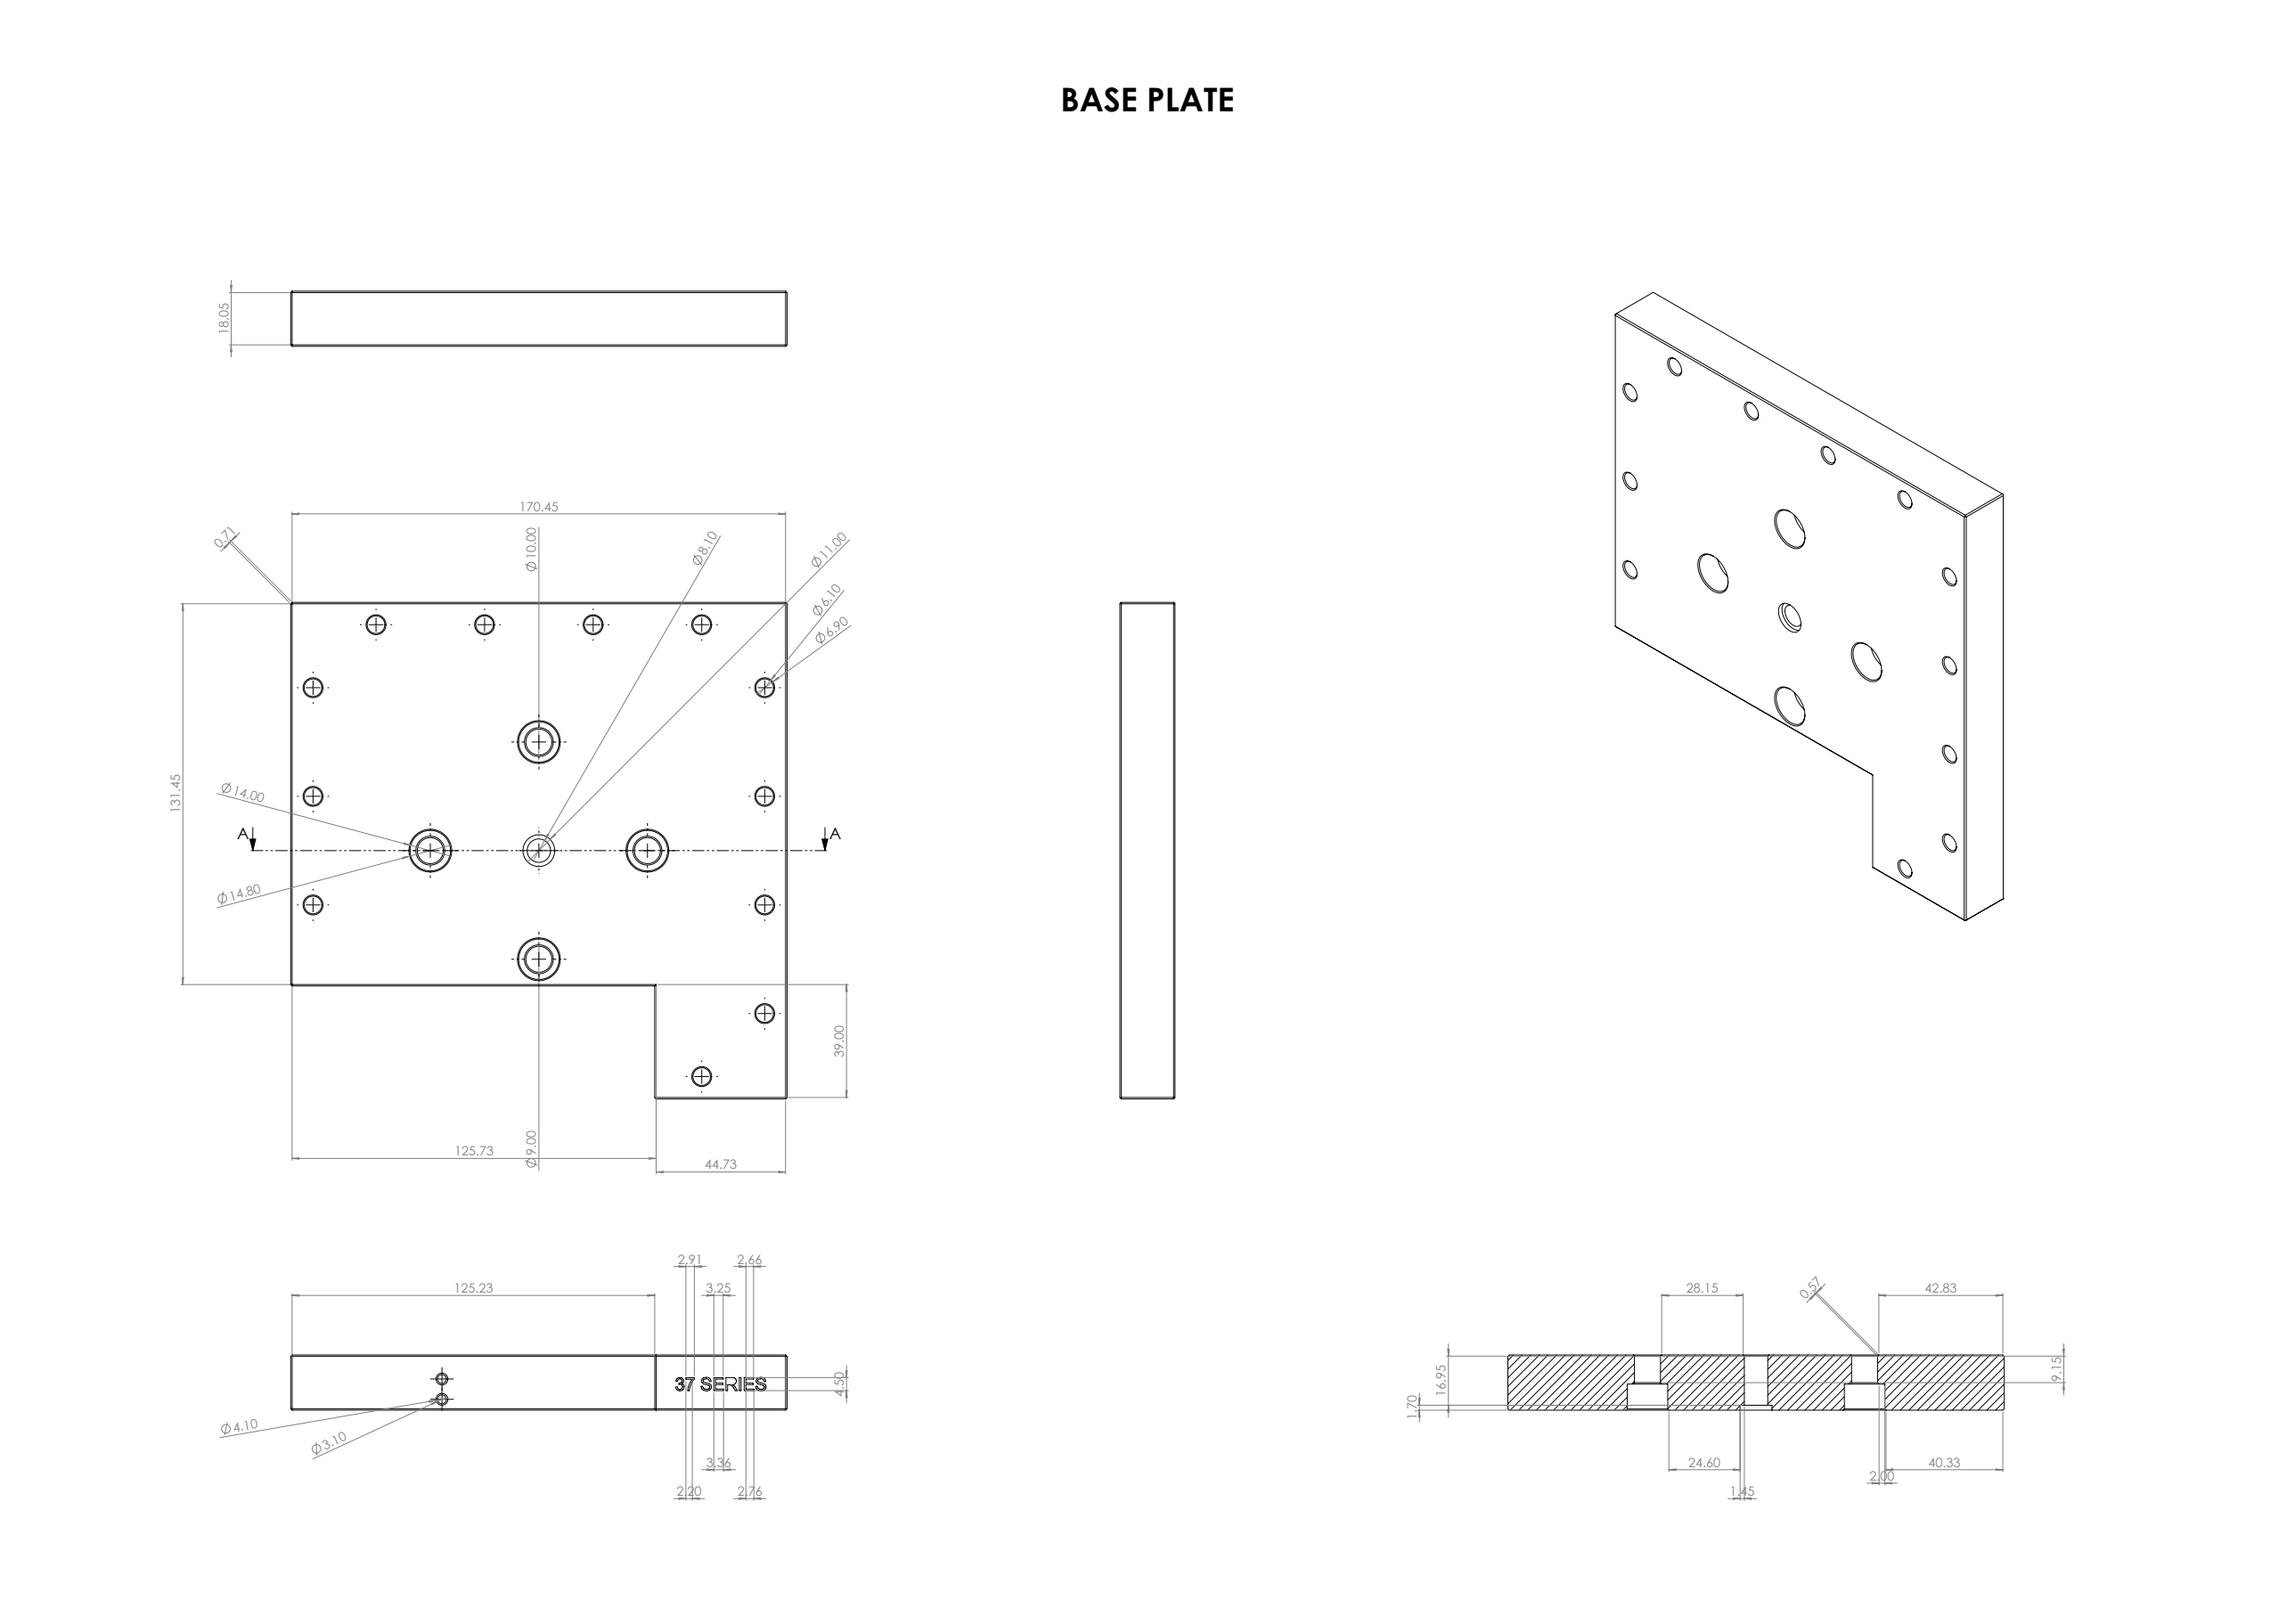
ISO-10303-21;
HEADER;
/* Generated by software containing ST-Developer
 * from STEP Tools, Inc. (www.steptools.com) 
 */

FILE_DESCRIPTION(
/* description */ (''),
/* implementation_level */ '2;1');

FILE_NAME(
/* name */ '01_Base_Plate.step',
/* time_stamp */ '2026-10-21T01:56:51-07:00',
/* author */ (''),
/* organization */ (''),
/* preprocessor_version */ 'ST-DEVELOPER v20.2',
/* originating_system */ 'Autodesk Translation Framework v15.15.0.0',
/* authorisation */ '');

FILE_SCHEMA (('AUTOMOTIVE_DESIGN { 1 0 10303 214 3 1 1 }'));
ENDSEC;

DATA;
#10=MECHANICAL_DESIGN_GEOMETRIC_PRESENTATION_REPRESENTATION('',(#270),#82384);
#232=SHAPE_REPRESENTATION_RELATIONSHIP('SRR','None',#82466,#251);
#251=ADVANCED_BREP_SHAPE_REPRESENTATION('',(#289),#82365);
#270=STYLED_ITEM('',(#82610),#289);
#289=MANIFOLD_SOLID_BREP('Body1',#30661);
#308=B_SPLINE_SURFACE_WITH_KNOTS('',2,1,((#41609,#41610),(#41611,#41612),
(#41613,#41614)),.UNSPECIFIED.,.F.,.F.,.F.,(3,3),(2,2),(0.,1.),(0.,0.0299999999999994),
 .UNSPECIFIED.);
#309=B_SPLINE_SURFACE_WITH_KNOTS('',2,1,((#41620,#41621),(#41622,#41623),
(#41624,#41625)),.UNSPECIFIED.,.F.,.F.,.F.,(3,3),(2,2),(0.,1.),(0.,0.0299999999999994),
 .UNSPECIFIED.);
#310=B_SPLINE_SURFACE_WITH_KNOTS('',2,1,((#41631,#41632),(#41633,#41634),
(#41635,#41636)),.UNSPECIFIED.,.F.,.F.,.F.,(3,3),(2,2),(0.,1.),(0.,0.0299999999999994),
 .UNSPECIFIED.);
#311=B_SPLINE_SURFACE_WITH_KNOTS('',2,1,((#41642,#41643),(#41644,#41645),
(#41646,#41647)),.UNSPECIFIED.,.F.,.F.,.F.,(3,3),(2,2),(0.,1.),(0.,0.0299999999999994),
 .UNSPECIFIED.);
#312=B_SPLINE_SURFACE_WITH_KNOTS('',2,1,((#41665,#41666),(#41667,#41668),
(#41669,#41670)),.UNSPECIFIED.,.F.,.F.,.F.,(3,3),(2,2),(0.,1.),(0.,0.0299999999999994),
 .UNSPECIFIED.);
#313=B_SPLINE_SURFACE_WITH_KNOTS('',2,1,((#41676,#41677),(#41678,#41679),
(#41680,#41681)),.UNSPECIFIED.,.F.,.F.,.F.,(3,3),(2,2),(0.,1.),(0.,0.0299999999999994),
 .UNSPECIFIED.);
#314=B_SPLINE_SURFACE_WITH_KNOTS('',2,1,((#41687,#41688),(#41689,#41690),
(#41691,#41692)),.UNSPECIFIED.,.F.,.F.,.F.,(3,3),(2,2),(0.,1.),(0.,0.0299999999999994),
 .UNSPECIFIED.);
#315=B_SPLINE_SURFACE_WITH_KNOTS('',2,1,((#41698,#41699),(#41700,#41701),
(#41702,#41703)),.UNSPECIFIED.,.F.,.F.,.F.,(3,3),(2,2),(0.,1.),(0.,0.0299999999999994),
 .UNSPECIFIED.);
#316=B_SPLINE_SURFACE_WITH_KNOTS('',2,1,((#41709,#41710),(#41711,#41712),
(#41713,#41714)),.UNSPECIFIED.,.F.,.F.,.F.,(3,3),(2,2),(0.,1.),(0.,0.0299999999999994),
 .UNSPECIFIED.);
#317=B_SPLINE_SURFACE_WITH_KNOTS('',2,1,((#41720,#41721),(#41722,#41723),
(#41724,#41725)),.UNSPECIFIED.,.F.,.F.,.F.,(3,3),(2,2),(0.,1.),(0.,0.0299999999999994),
 .UNSPECIFIED.);
#318=B_SPLINE_SURFACE_WITH_KNOTS('',2,1,((#41731,#41732),(#41733,#41734),
(#41735,#41736)),.UNSPECIFIED.,.F.,.F.,.F.,(3,3),(2,2),(0.,1.),(0.,0.0299999999999994),
 .UNSPECIFIED.);
#319=B_SPLINE_SURFACE_WITH_KNOTS('',2,1,((#41806,#41807),(#41808,#41809),
(#41810,#41811)),.UNSPECIFIED.,.F.,.F.,.F.,(3,3),(2,2),(0.,1.),(0.,0.0299999999999994),
 .UNSPECIFIED.);
#320=B_SPLINE_SURFACE_WITH_KNOTS('',2,1,((#41819,#41820),(#41821,#41822),
(#41823,#41824)),.UNSPECIFIED.,.F.,.F.,.F.,(3,3),(2,2),(0.,1.),(0.,0.0299999999999994),
 .UNSPECIFIED.);
#321=B_SPLINE_SURFACE_WITH_KNOTS('',2,1,((#41834,#41835),(#41836,#41837),
(#41838,#41839)),.UNSPECIFIED.,.F.,.F.,.F.,(3,3),(2,2),(0.,1.),(0.,0.0299999999999994),
 .UNSPECIFIED.);
#322=B_SPLINE_SURFACE_WITH_KNOTS('',2,1,((#41845,#41846),(#41847,#41848),
(#41849,#41850)),.UNSPECIFIED.,.F.,.F.,.F.,(3,3),(2,2),(0.,1.),(0.,0.0299999999999994),
 .UNSPECIFIED.);
#323=B_SPLINE_SURFACE_WITH_KNOTS('',2,1,((#41856,#41857),(#41858,#41859),
(#41860,#41861)),.UNSPECIFIED.,.F.,.F.,.F.,(3,3),(2,2),(0.,1.),(0.,0.0299999999999994),
 .UNSPECIFIED.);
#324=B_SPLINE_SURFACE_WITH_KNOTS('',2,1,((#41883,#41884),(#41885,#41886),
(#41887,#41888)),.UNSPECIFIED.,.F.,.F.,.F.,(3,3),(2,2),(0.,1.),(0.,0.0299999999999994),
 .UNSPECIFIED.);
#325=B_SPLINE_SURFACE_WITH_KNOTS('',2,1,((#41893,#41894),(#41895,#41896),
(#41897,#41898)),.UNSPECIFIED.,.F.,.F.,.F.,(3,3),(2,2),(0.,1.),(0.,0.0299999999999994),
 .UNSPECIFIED.);
#326=B_SPLINE_SURFACE_WITH_KNOTS('',2,1,((#41906,#41907),(#41908,#41909),
(#41910,#41911)),.UNSPECIFIED.,.F.,.F.,.F.,(3,3),(2,2),(0.,1.),(0.,0.0299999999999994),
 .UNSPECIFIED.);
#327=B_SPLINE_SURFACE_WITH_KNOTS('',2,1,((#41917,#41918),(#41919,#41920),
(#41921,#41922)),.UNSPECIFIED.,.F.,.F.,.F.,(3,3),(2,2),(0.,1.),(0.,0.0299999999999994),
 .UNSPECIFIED.);
#328=B_SPLINE_SURFACE_WITH_KNOTS('',2,1,((#41928,#41929),(#41930,#41931),
(#41932,#41933)),.UNSPECIFIED.,.F.,.F.,.F.,(3,3),(2,2),(0.,1.),(0.,0.0299999999999994),
 .UNSPECIFIED.);
#329=B_SPLINE_SURFACE_WITH_KNOTS('',2,1,((#41939,#41940),(#41941,#41942),
(#41943,#41944)),.UNSPECIFIED.,.F.,.F.,.F.,(3,3),(2,2),(0.,1.),(0.,0.0299999999999994),
 .UNSPECIFIED.);
#330=B_SPLINE_SURFACE_WITH_KNOTS('',2,1,((#41950,#41951),(#41952,#41953),
(#41954,#41955)),.UNSPECIFIED.,.F.,.F.,.F.,(3,3),(2,2),(0.,1.),(0.,0.0299999999999994),
 .UNSPECIFIED.);
#331=B_SPLINE_SURFACE_WITH_KNOTS('',2,1,((#41961,#41962),(#41963,#41964),
(#41965,#41966)),.UNSPECIFIED.,.F.,.F.,.F.,(3,3),(2,2),(0.,1.),(0.,0.0299999999999994),
 .UNSPECIFIED.);
#332=B_SPLINE_SURFACE_WITH_KNOTS('',2,1,((#41972,#41973),(#41974,#41975),
(#41976,#41977)),.UNSPECIFIED.,.F.,.F.,.F.,(3,3),(2,2),(0.,1.),(0.,0.0299999999999994),
 .UNSPECIFIED.);
#333=B_SPLINE_SURFACE_WITH_KNOTS('',2,1,((#41983,#41984),(#41985,#41986),
(#41987,#41988)),.UNSPECIFIED.,.F.,.F.,.F.,(3,3),(2,2),(0.,1.),(0.,0.0299999999999994),
 .UNSPECIFIED.);
#334=B_SPLINE_SURFACE_WITH_KNOTS('',2,1,((#41994,#41995),(#41996,#41997),
(#41998,#41999)),.UNSPECIFIED.,.F.,.F.,.F.,(3,3),(2,2),(0.,1.),(0.,0.0299999999999994),
 .UNSPECIFIED.);
#335=B_SPLINE_SURFACE_WITH_KNOTS('',2,1,((#42005,#42006),(#42007,#42008),
(#42009,#42010)),.UNSPECIFIED.,.F.,.F.,.F.,(3,3),(2,2),(0.,1.),(0.,0.0299999999999994),
 .UNSPECIFIED.);
#336=B_SPLINE_SURFACE_WITH_KNOTS('',2,1,((#42016,#42017),(#42018,#42019),
(#42020,#42021)),.UNSPECIFIED.,.F.,.F.,.F.,(3,3),(2,2),(0.,1.),(0.,0.0299999999999994),
 .UNSPECIFIED.);
#337=B_SPLINE_SURFACE_WITH_KNOTS('',2,1,((#42027,#42028),(#42029,#42030),
(#42031,#42032)),.UNSPECIFIED.,.F.,.F.,.F.,(3,3),(2,2),(0.,1.),(0.,0.0299999999999994),
 .UNSPECIFIED.);
#338=B_SPLINE_SURFACE_WITH_KNOTS('',2,1,((#42042,#42043),(#42044,#42045),
(#42046,#42047)),.UNSPECIFIED.,.F.,.F.,.F.,(3,3),(2,2),(0.,1.),(0.,0.0299999999999994),
 .UNSPECIFIED.);
#339=B_SPLINE_SURFACE_WITH_KNOTS('',2,1,((#42053,#42054),(#42055,#42056),
(#42057,#42058)),.UNSPECIFIED.,.F.,.F.,.F.,(3,3),(2,2),(0.,1.),(0.,0.0299999999999994),
 .UNSPECIFIED.);
#340=B_SPLINE_SURFACE_WITH_KNOTS('',2,1,((#42064,#42065),(#42066,#42067),
(#42068,#42069)),.UNSPECIFIED.,.F.,.F.,.F.,(3,3),(2,2),(0.,1.),(0.,0.0299999999999994),
 .UNSPECIFIED.);
#341=B_SPLINE_SURFACE_WITH_KNOTS('',2,1,((#42075,#42076),(#42077,#42078),
(#42079,#42080)),.UNSPECIFIED.,.F.,.F.,.F.,(3,3),(2,2),(0.,1.),(0.,0.0299999999999994),
 .UNSPECIFIED.);
#342=B_SPLINE_SURFACE_WITH_KNOTS('',2,1,((#42086,#42087),(#42088,#42089),
(#42090,#42091)),.UNSPECIFIED.,.F.,.F.,.F.,(3,3),(2,2),(0.,1.),(0.,0.0299999999999994),
 .UNSPECIFIED.);
#343=B_SPLINE_SURFACE_WITH_KNOTS('',2,1,((#42097,#42098),(#42099,#42100),
(#42101,#42102)),.UNSPECIFIED.,.F.,.F.,.F.,(3,3),(2,2),(0.,1.),(0.,0.0299999999999994),
 .UNSPECIFIED.);
#344=B_SPLINE_SURFACE_WITH_KNOTS('',2,1,((#42108,#42109),(#42110,#42111),
(#42112,#42113)),.UNSPECIFIED.,.F.,.F.,.F.,(3,3),(2,2),(0.,1.),(0.,0.0299999999999994),
 .UNSPECIFIED.);
#345=B_SPLINE_SURFACE_WITH_KNOTS('',2,1,((#42119,#42120),(#42121,#42122),
(#42123,#42124)),.UNSPECIFIED.,.F.,.F.,.F.,(3,3),(2,2),(0.,1.),(0.,0.0299999999999994),
 .UNSPECIFIED.);
#346=B_SPLINE_SURFACE_WITH_KNOTS('',2,1,((#42130,#42131),(#42132,#42133),
(#42134,#42135)),.UNSPECIFIED.,.F.,.F.,.F.,(3,3),(2,2),(0.,1.),(0.,0.0299999999999994),
 .UNSPECIFIED.);
#347=B_SPLINE_SURFACE_WITH_KNOTS('',2,1,((#42141,#42142),(#42143,#42144),
(#42145,#42146)),.UNSPECIFIED.,.F.,.F.,.F.,(3,3),(2,2),(0.,1.),(0.,0.0299999999999994),
 .UNSPECIFIED.);
#348=B_SPLINE_SURFACE_WITH_KNOTS('',2,1,((#42152,#42153),(#42154,#42155),
(#42156,#42157)),.UNSPECIFIED.,.F.,.F.,.F.,(3,3),(2,2),(0.,1.),(0.,0.0299999999999994),
 .UNSPECIFIED.);
#349=B_SPLINE_SURFACE_WITH_KNOTS('',2,1,((#42163,#42164),(#42165,#42166),
(#42167,#42168)),.UNSPECIFIED.,.F.,.F.,.F.,(3,3),(2,2),(0.,1.),(0.,0.0299999999999994),
 .UNSPECIFIED.);
#350=B_SPLINE_SURFACE_WITH_KNOTS('',2,1,((#42174,#42175),(#42176,#42177),
(#42178,#42179)),.UNSPECIFIED.,.F.,.F.,.F.,(3,3),(2,2),(0.,1.),(0.,0.0299999999999994),
 .UNSPECIFIED.);
#351=B_SPLINE_SURFACE_WITH_KNOTS('',2,1,((#42185,#42186),(#42187,#42188),
(#42189,#42190)),.UNSPECIFIED.,.F.,.F.,.F.,(3,3),(2,2),(0.,1.),(0.,0.0299999999999994),
 .UNSPECIFIED.);
#352=B_SPLINE_SURFACE_WITH_KNOTS('',2,1,((#42196,#42197),(#42198,#42199),
(#42200,#42201)),.UNSPECIFIED.,.F.,.F.,.F.,(3,3),(2,2),(0.,1.),(0.,0.0299999999999994),
 .UNSPECIFIED.);
#353=B_SPLINE_SURFACE_WITH_KNOTS('',2,1,((#42207,#42208),(#42209,#42210),
(#42211,#42212)),.UNSPECIFIED.,.F.,.F.,.F.,(3,3),(2,2),(0.,1.),(0.,0.0299999999999994),
 .UNSPECIFIED.);
#354=B_SPLINE_SURFACE_WITH_KNOTS('',2,1,((#42218,#42219),(#42220,#42221),
(#42222,#42223)),.UNSPECIFIED.,.F.,.F.,.F.,(3,3),(2,2),(0.,1.),(0.,0.0299999999999994),
 .UNSPECIFIED.);
#355=B_SPLINE_SURFACE_WITH_KNOTS('',2,1,((#42229,#42230),(#42231,#42232),
(#42233,#42234)),.UNSPECIFIED.,.F.,.F.,.F.,(3,3),(2,2),(0.,1.),(0.,0.0299999999999994),
 .UNSPECIFIED.);
#356=B_SPLINE_SURFACE_WITH_KNOTS('',2,1,((#42244,#42245),(#42246,#42247),
(#42248,#42249)),.UNSPECIFIED.,.F.,.F.,.F.,(3,3),(2,2),(0.,1.),(0.,0.0299999999999994),
 .UNSPECIFIED.);
#357=B_SPLINE_SURFACE_WITH_KNOTS('',2,1,((#42255,#42256),(#42257,#42258),
(#42259,#42260)),.UNSPECIFIED.,.F.,.F.,.F.,(3,3),(2,2),(0.,1.),(0.,0.0299999999999994),
 .UNSPECIFIED.);
#358=B_SPLINE_SURFACE_WITH_KNOTS('',2,1,((#42265,#42266),(#42267,#42268),
(#42269,#42270)),.UNSPECIFIED.,.F.,.F.,.F.,(3,3),(2,2),(0.,1.),(0.,0.0299999999999994),
 .UNSPECIFIED.);
#359=B_SPLINE_SURFACE_WITH_KNOTS('',2,1,((#42278,#42279),(#42280,#42281),
(#42282,#42283)),.UNSPECIFIED.,.F.,.F.,.F.,(3,3),(2,2),(0.,1.),(0.,0.0299999999999994),
 .UNSPECIFIED.);
#360=B_SPLINE_SURFACE_WITH_KNOTS('',2,1,((#42289,#42290),(#42291,#42292),
(#42293,#42294)),.UNSPECIFIED.,.F.,.F.,.F.,(3,3),(2,2),(0.,1.),(0.,0.0299999999999994),
 .UNSPECIFIED.);
#361=B_SPLINE_SURFACE_WITH_KNOTS('',2,1,((#42300,#42301),(#42302,#42303),
(#42304,#42305)),.UNSPECIFIED.,.F.,.F.,.F.,(3,3),(2,2),(0.,1.),(0.,0.0299999999999994),
 .UNSPECIFIED.);
#362=B_SPLINE_SURFACE_WITH_KNOTS('',2,1,((#42311,#42312),(#42313,#42314),
(#42315,#42316)),.UNSPECIFIED.,.F.,.F.,.F.,(3,3),(2,2),(0.,1.),(0.,0.0299999999999994),
 .UNSPECIFIED.);
#363=B_SPLINE_SURFACE_WITH_KNOTS('',2,1,((#42322,#42323),(#42324,#42325),
(#42326,#42327)),.UNSPECIFIED.,.F.,.F.,.F.,(3,3),(2,2),(0.,1.),(0.,0.0299999999999994),
 .UNSPECIFIED.);
#364=B_SPLINE_SURFACE_WITH_KNOTS('',2,1,((#42333,#42334),(#42335,#42336),
(#42337,#42338)),.UNSPECIFIED.,.F.,.F.,.F.,(3,3),(2,2),(0.,1.),(0.,0.0299999999999994),
 .UNSPECIFIED.);
#365=B_SPLINE_SURFACE_WITH_KNOTS('',2,1,((#42344,#42345),(#42346,#42347),
(#42348,#42349)),.UNSPECIFIED.,.F.,.F.,.F.,(3,3),(2,2),(0.,1.),(0.,0.0299999999999994),
 .UNSPECIFIED.);
#366=B_SPLINE_SURFACE_WITH_KNOTS('',2,1,((#42355,#42356),(#42357,#42358),
(#42359,#42360)),.UNSPECIFIED.,.F.,.F.,.F.,(3,3),(2,2),(0.,1.),(0.,0.0299999999999994),
 .UNSPECIFIED.);
#367=B_SPLINE_SURFACE_WITH_KNOTS('',2,1,((#42366,#42367),(#42368,#42369),
(#42370,#42371)),.UNSPECIFIED.,.F.,.F.,.F.,(3,3),(2,2),(0.,1.),(0.,0.0299999999999994),
 .UNSPECIFIED.);
#368=B_SPLINE_SURFACE_WITH_KNOTS('',2,1,((#42377,#42378),(#42379,#42380),
(#42381,#42382)),.UNSPECIFIED.,.F.,.F.,.F.,(3,3),(2,2),(0.,1.),(0.,0.0299999999999994),
 .UNSPECIFIED.);
#369=B_SPLINE_SURFACE_WITH_KNOTS('',2,1,((#42392,#42393),(#42394,#42395),
(#42396,#42397)),.UNSPECIFIED.,.F.,.F.,.F.,(3,3),(2,2),(0.,1.),(0.,0.0299999999999994),
 .UNSPECIFIED.);
#370=B_SPLINE_SURFACE_WITH_KNOTS('',2,1,((#42403,#42404),(#42405,#42406),
(#42407,#42408)),.UNSPECIFIED.,.F.,.F.,.F.,(3,3),(2,2),(0.,1.),(0.,0.0299999999999994),
 .UNSPECIFIED.);
#371=B_SPLINE_SURFACE_WITH_KNOTS('',2,1,((#42414,#42415),(#42416,#42417),
(#42418,#42419)),.UNSPECIFIED.,.F.,.F.,.F.,(3,3),(2,2),(0.,1.),(0.,0.0299999999999994),
 .UNSPECIFIED.);
#372=B_SPLINE_SURFACE_WITH_KNOTS('',2,1,((#42425,#42426),(#42427,#42428),
(#42429,#42430)),.UNSPECIFIED.,.F.,.F.,.F.,(3,3),(2,2),(0.,1.),(0.,0.0299999999999994),
 .UNSPECIFIED.);
#373=B_SPLINE_SURFACE_WITH_KNOTS('',2,1,((#42436,#42437),(#42438,#42439),
(#42440,#42441)),.UNSPECIFIED.,.F.,.F.,.F.,(3,3),(2,2),(0.,1.),(0.,0.0299999999999994),
 .UNSPECIFIED.);
#374=B_SPLINE_SURFACE_WITH_KNOTS('',2,1,((#42447,#42448),(#42449,#42450),
(#42451,#42452)),.UNSPECIFIED.,.F.,.F.,.F.,(3,3),(2,2),(0.,1.),(0.,0.0299999999999994),
 .UNSPECIFIED.);
#375=B_SPLINE_SURFACE_WITH_KNOTS('',2,1,((#42458,#42459),(#42460,#42461),
(#42462,#42463)),.UNSPECIFIED.,.F.,.F.,.F.,(3,3),(2,2),(0.,1.),(0.,0.0299999999999994),
 .UNSPECIFIED.);
#376=B_SPLINE_SURFACE_WITH_KNOTS('',2,1,((#42473,#42474),(#42475,#42476),
(#42477,#42478)),.UNSPECIFIED.,.F.,.F.,.F.,(3,3),(2,2),(0.,1.),(0.,0.0299999999999994),
 .UNSPECIFIED.);
#377=B_SPLINE_SURFACE_WITH_KNOTS('',2,1,((#42484,#42485),(#42486,#42487),
(#42488,#42489)),.UNSPECIFIED.,.F.,.F.,.F.,(3,3),(2,2),(0.,1.),(0.,0.0299999999999994),
 .UNSPECIFIED.);
#378=B_SPLINE_SURFACE_WITH_KNOTS('',2,1,((#42495,#42496),(#42497,#42498),
(#42499,#42500)),.UNSPECIFIED.,.F.,.F.,.F.,(3,3),(2,2),(0.,1.),(0.,0.0299999999999994),
 .UNSPECIFIED.);
#379=B_SPLINE_SURFACE_WITH_KNOTS('',2,1,((#42506,#42507),(#42508,#42509),
(#42510,#42511)),.UNSPECIFIED.,.F.,.F.,.F.,(3,3),(2,2),(0.,1.),(0.,0.0299999999999994),
 .UNSPECIFIED.);
#380=B_SPLINE_SURFACE_WITH_KNOTS('',2,1,((#42517,#42518),(#42519,#42520),
(#42521,#42522)),.UNSPECIFIED.,.F.,.F.,.F.,(3,3),(2,2),(0.,1.),(0.,0.0299999999999994),
 .UNSPECIFIED.);
#381=B_SPLINE_SURFACE_WITH_KNOTS('',2,1,((#42528,#42529),(#42530,#42531),
(#42532,#42533)),.UNSPECIFIED.,.F.,.F.,.F.,(3,3),(2,2),(0.,1.),(0.,0.0299999999999994),
 .UNSPECIFIED.);
#382=B_SPLINE_SURFACE_WITH_KNOTS('',2,1,((#42539,#42540),(#42541,#42542),
(#42543,#42544)),.UNSPECIFIED.,.F.,.F.,.F.,(3,3),(2,2),(0.,1.),(0.,0.0299999999999994),
 .UNSPECIFIED.);
#383=B_SPLINE_SURFACE_WITH_KNOTS('',2,1,((#42554,#42555),(#42556,#42557),
(#42558,#42559)),.UNSPECIFIED.,.F.,.F.,.F.,(3,3),(2,2),(0.,1.),(0.,0.0299999999999994),
 .UNSPECIFIED.);
#384=B_SPLINE_SURFACE_WITH_KNOTS('',2,1,((#42565,#42566),(#42567,#42568),
(#42569,#42570)),.UNSPECIFIED.,.F.,.F.,.F.,(3,3),(2,2),(0.,1.),(0.,0.0299999999999994),
 .UNSPECIFIED.);
#385=B_SPLINE_SURFACE_WITH_KNOTS('',2,1,((#42592,#42593),(#42594,#42595),
(#42596,#42597)),.UNSPECIFIED.,.F.,.F.,.F.,(3,3),(2,2),(0.,1.),(0.,0.0299999999999994),
 .UNSPECIFIED.);
#386=B_SPLINE_SURFACE_WITH_KNOTS('',2,1,((#42605,#42606),(#42607,#42608),
(#42609,#42610)),.UNSPECIFIED.,.F.,.F.,.F.,(3,3),(2,2),(0.,1.),(0.,0.0299999999999994),
 .UNSPECIFIED.);
#387=B_SPLINE_SURFACE_WITH_KNOTS('',2,1,((#42616,#42617),(#42618,#42619),
(#42620,#42621)),.UNSPECIFIED.,.F.,.F.,.F.,(3,3),(2,2),(0.,1.),(0.,0.0299999999999994),
 .UNSPECIFIED.);
#388=B_SPLINE_SURFACE_WITH_KNOTS('',2,1,((#42627,#42628),(#42629,#42630),
(#42631,#42632)),.UNSPECIFIED.,.F.,.F.,.F.,(3,3),(2,2),(0.,1.),(0.,0.0299999999999994),
 .UNSPECIFIED.);
#389=B_SPLINE_SURFACE_WITH_KNOTS('',2,1,((#42638,#42639),(#42640,#42641),
(#42642,#42643)),.UNSPECIFIED.,.F.,.F.,.F.,(3,3),(2,2),(0.,1.),(0.,0.0299999999999994),
 .UNSPECIFIED.);
#390=B_SPLINE_SURFACE_WITH_KNOTS('',2,1,((#42649,#42650),(#42651,#42652),
(#42653,#42654)),.UNSPECIFIED.,.F.,.F.,.F.,(3,3),(2,2),(0.,1.),(0.,0.0299999999999994),
 .UNSPECIFIED.);
#391=B_SPLINE_SURFACE_WITH_KNOTS('',2,1,((#42660,#42661),(#42662,#42663),
(#42664,#42665)),.UNSPECIFIED.,.F.,.F.,.F.,(3,3),(2,2),(0.,1.),(0.,0.0299999999999994),
 .UNSPECIFIED.);
#392=B_SPLINE_SURFACE_WITH_KNOTS('',2,1,((#42671,#42672),(#42673,#42674),
(#42675,#42676)),.UNSPECIFIED.,.F.,.F.,.F.,(3,3),(2,2),(0.,1.),(0.,0.0299999999999994),
 .UNSPECIFIED.);
#393=B_SPLINE_SURFACE_WITH_KNOTS('',2,1,((#42682,#42683),(#42684,#42685),
(#42686,#42687)),.UNSPECIFIED.,.F.,.F.,.F.,(3,3),(2,2),(0.,1.),(0.,0.0299999999999994),
 .UNSPECIFIED.);
#394=B_SPLINE_SURFACE_WITH_KNOTS('',2,1,((#42693,#42694),(#42695,#42696),
(#42697,#42698)),.UNSPECIFIED.,.F.,.F.,.F.,(3,3),(2,2),(0.,1.),(0.,0.0299999999999994),
 .UNSPECIFIED.);
#395=B_SPLINE_SURFACE_WITH_KNOTS('',2,1,((#42704,#42705),(#42706,#42707),
(#42708,#42709)),.UNSPECIFIED.,.F.,.F.,.F.,(3,3),(2,2),(0.,1.),(0.,0.0299999999999994),
 .UNSPECIFIED.);
#396=B_SPLINE_SURFACE_WITH_KNOTS('',2,1,((#42715,#42716),(#42717,#42718),
(#42719,#42720)),.UNSPECIFIED.,.F.,.F.,.F.,(3,3),(2,2),(0.,1.),(0.,0.0299999999999994),
 .UNSPECIFIED.);
#397=B_SPLINE_SURFACE_WITH_KNOTS('',2,1,((#42726,#42727),(#42728,#42729),
(#42730,#42731)),.UNSPECIFIED.,.F.,.F.,.F.,(3,3),(2,2),(0.,1.),(0.,0.0299999999999994),
 .UNSPECIFIED.);
#398=B_SPLINE_SURFACE_WITH_KNOTS('',2,1,((#42741,#42742),(#42743,#42744),
(#42745,#42746)),.UNSPECIFIED.,.F.,.F.,.F.,(3,3),(2,2),(0.,1.),(0.,0.0299999999999994),
 .UNSPECIFIED.);
#399=B_SPLINE_SURFACE_WITH_KNOTS('',2,1,((#42752,#42753),(#42754,#42755),
(#42756,#42757)),.UNSPECIFIED.,.F.,.F.,.F.,(3,3),(2,2),(0.,1.),(0.,0.0299999999999994),
 .UNSPECIFIED.);
#400=B_SPLINE_SURFACE_WITH_KNOTS('',2,1,((#42763,#42764),(#42765,#42766),
(#42767,#42768)),.UNSPECIFIED.,.F.,.F.,.F.,(3,3),(2,2),(0.,1.),(0.,0.0299999999999994),
 .UNSPECIFIED.);
#401=B_SPLINE_SURFACE_WITH_KNOTS('',2,1,((#42774,#42775),(#42776,#42777),
(#42778,#42779)),.UNSPECIFIED.,.F.,.F.,.F.,(3,3),(2,2),(0.,1.),(0.,0.0299999999999994),
 .UNSPECIFIED.);
#402=B_SPLINE_SURFACE_WITH_KNOTS('',2,1,((#42785,#42786),(#42787,#42788),
(#42789,#42790)),.UNSPECIFIED.,.F.,.F.,.F.,(3,3),(2,2),(0.,1.),(0.,0.0299999999999994),
 .UNSPECIFIED.);
#403=B_SPLINE_SURFACE_WITH_KNOTS('',2,1,((#42796,#42797),(#42798,#42799),
(#42800,#42801)),.UNSPECIFIED.,.F.,.F.,.F.,(3,3),(2,2),(0.,1.),(0.,0.0299999999999994),
 .UNSPECIFIED.);
#404=B_SPLINE_SURFACE_WITH_KNOTS('',2,1,((#42807,#42808),(#42809,#42810),
(#42811,#42812)),.UNSPECIFIED.,.F.,.F.,.F.,(3,3),(2,2),(0.,1.),(0.,0.0299999999999994),
 .UNSPECIFIED.);
#405=B_SPLINE_SURFACE_WITH_KNOTS('',2,1,((#42818,#42819),(#42820,#42821),
(#42822,#42823)),.UNSPECIFIED.,.F.,.F.,.F.,(3,3),(2,2),(0.,1.),(0.,0.0299999999999994),
 .UNSPECIFIED.);
#406=B_SPLINE_SURFACE_WITH_KNOTS('',2,1,((#42829,#42830),(#42831,#42832),
(#42833,#42834)),.UNSPECIFIED.,.F.,.F.,.F.,(3,3),(2,2),(0.,1.),(0.,0.0299999999999994),
 .UNSPECIFIED.);
#407=B_SPLINE_SURFACE_WITH_KNOTS('',2,1,((#42840,#42841),(#42842,#42843),
(#42844,#42845)),.UNSPECIFIED.,.F.,.F.,.F.,(3,3),(2,2),(0.,1.),(0.,0.0299999999999994),
 .UNSPECIFIED.);
#408=B_SPLINE_SURFACE_WITH_KNOTS('',2,1,((#42851,#42852),(#42853,#42854),
(#42855,#42856)),.UNSPECIFIED.,.F.,.F.,.F.,(3,3),(2,2),(0.,1.),(0.,0.0299999999999994),
 .UNSPECIFIED.);
#409=B_SPLINE_SURFACE_WITH_KNOTS('',2,1,((#42862,#42863),(#42864,#42865),
(#42866,#42867)),.UNSPECIFIED.,.F.,.F.,.F.,(3,3),(2,2),(0.,1.),(0.,0.0299999999999994),
 .UNSPECIFIED.);
#410=B_SPLINE_SURFACE_WITH_KNOTS('',2,1,((#42873,#42874),(#42875,#42876),
(#42877,#42878)),.UNSPECIFIED.,.F.,.F.,.F.,(3,3),(2,2),(0.,1.),(0.,0.0299999999999994),
 .UNSPECIFIED.);
#411=B_SPLINE_SURFACE_WITH_KNOTS('',2,1,((#42884,#42885),(#42886,#42887),
(#42888,#42889)),.UNSPECIFIED.,.F.,.F.,.F.,(3,3),(2,2),(0.,1.),(0.,0.0299999999999994),
 .UNSPECIFIED.);
#412=B_SPLINE_SURFACE_WITH_KNOTS('',2,1,((#42895,#42896),(#42897,#42898),
(#42899,#42900)),.UNSPECIFIED.,.F.,.F.,.F.,(3,3),(2,2),(0.,1.),(0.,0.0299999999999994),
 .UNSPECIFIED.);
#413=B_SPLINE_SURFACE_WITH_KNOTS('',2,1,((#42906,#42907),(#42908,#42909),
(#42910,#42911)),.UNSPECIFIED.,.F.,.F.,.F.,(3,3),(2,2),(0.,1.),(0.,0.0299999999999994),
 .UNSPECIFIED.);
#414=B_SPLINE_SURFACE_WITH_KNOTS('',2,1,((#42917,#42918),(#42919,#42920),
(#42921,#42922)),.UNSPECIFIED.,.F.,.F.,.F.,(3,3),(2,2),(0.,1.),(0.,0.0299999999999994),
 .UNSPECIFIED.);
#415=B_SPLINE_SURFACE_WITH_KNOTS('',2,1,((#42928,#42929),(#42930,#42931),
(#42932,#42933)),.UNSPECIFIED.,.F.,.F.,.F.,(3,3),(2,2),(0.,1.),(0.,0.0299999999999994),
 .UNSPECIFIED.);
#416=B_SPLINE_SURFACE_WITH_KNOTS('',2,1,((#42943,#42944),(#42945,#42946),
(#42947,#42948)),.UNSPECIFIED.,.F.,.F.,.F.,(3,3),(2,2),(0.,1.),(0.,0.0299999999999994),
 .UNSPECIFIED.);
#417=B_SPLINE_SURFACE_WITH_KNOTS('',2,1,((#42954,#42955),(#42956,#42957),
(#42958,#42959)),.UNSPECIFIED.,.F.,.F.,.F.,(3,3),(2,2),(0.,1.),(0.,0.0299999999999994),
 .UNSPECIFIED.);
#433=CYLINDRICAL_SURFACE('',#30907,1.55);
#434=CYLINDRICAL_SURFACE('',#30911,1.55);
#435=CYLINDRICAL_SURFACE('',#30916,4.5);
#436=CYLINDRICAL_SURFACE('',#30923,4.5);
#437=CYLINDRICAL_SURFACE('',#30930,4.5);
#438=CYLINDRICAL_SURFACE('',#30937,4.5);
#439=CYLINDRICAL_SURFACE('',#31038,4.05);
#440=CYLINDRICAL_SURFACE('',#31042,3.05);
#441=CYLINDRICAL_SURFACE('',#31046,3.05);
#442=CYLINDRICAL_SURFACE('',#31050,3.05);
#443=CYLINDRICAL_SURFACE('',#31054,3.05000000000001);
#444=CYLINDRICAL_SURFACE('',#31058,3.05);
#445=CYLINDRICAL_SURFACE('',#31062,3.05000000000001);
#446=CYLINDRICAL_SURFACE('',#31066,3.05);
#447=CYLINDRICAL_SURFACE('',#31070,3.05);
#448=CYLINDRICAL_SURFACE('',#31074,3.05000000000001);
#449=CYLINDRICAL_SURFACE('',#31078,3.05);
#450=CYLINDRICAL_SURFACE('',#31082,3.05000000000001);
#451=CYLINDRICAL_SURFACE('',#31086,3.05);
#452=CYLINDRICAL_SURFACE('',#31090,7.);
#453=CYLINDRICAL_SURFACE('',#31093,7.);
#454=CYLINDRICAL_SURFACE('',#31096,7.);
#455=CYLINDRICAL_SURFACE('',#31099,7.);
#456=CYLINDRICAL_SURFACE('',#31118,5.5);
#1036=CIRCLE('',#30903,2.05);
#1037=CIRCLE('',#30904,1.55);
#1038=CIRCLE('',#30906,2.05);
#1039=CIRCLE('',#30908,1.55);
#1040=CIRCLE('',#30910,1.55);
#1041=CIRCLE('',#30912,1.55);
#1042=CIRCLE('',#30914,4.5);
#1043=CIRCLE('',#30915,5.);
#1044=CIRCLE('',#30917,4.5);
#1045=CIRCLE('',#30919,7.);
#1046=CIRCLE('',#30921,4.5);
#1047=CIRCLE('',#30922,5.);
#1048=CIRCLE('',#30924,4.5);
#1049=CIRCLE('',#30926,7.);
#1050=CIRCLE('',#30928,4.5);
#1051=CIRCLE('',#30929,5.);
#1052=CIRCLE('',#30931,4.5);
#1053=CIRCLE('',#30933,7.);
#1054=CIRCLE('',#30935,4.5);
#1055=CIRCLE('',#30936,5.);
#1056=CIRCLE('',#30938,4.5);
#1057=CIRCLE('',#30940,7.);
#1058=CIRCLE('',#30956,3.45);
#1059=CIRCLE('',#30957,3.45);
#1060=CIRCLE('',#30958,3.45);
#1061=CIRCLE('',#30959,3.45);
#1062=CIRCLE('',#30960,3.45);
#1063=CIRCLE('',#30961,3.45);
#1064=CIRCLE('',#30962,7.4);
#1065=CIRCLE('',#30963,7.4);
#1066=CIRCLE('',#30964,5.5);
#1067=CIRCLE('',#30965,7.4);
#1068=CIRCLE('',#30966,7.4);
#1069=CIRCLE('',#30967,3.45);
#1070=CIRCLE('',#30968,3.45);
#1071=CIRCLE('',#30969,3.45);
#1072=CIRCLE('',#30970,3.45);
#1073=CIRCLE('',#30971,3.45);
#1074=CIRCLE('',#30972,3.45);
#1075=CIRCLE('',#30975,4.45);
#1076=CIRCLE('',#30976,4.9);
#1077=CIRCLE('',#30977,4.9);
#1078=CIRCLE('',#30978,4.9);
#1079=CIRCLE('',#30979,4.9);
#1080=CIRCLE('',#31037,4.05);
#1081=CIRCLE('',#31039,4.05);
#1082=CIRCLE('',#31041,3.05);
#1083=CIRCLE('',#31043,3.05);
#1084=CIRCLE('',#31045,3.05);
#1085=CIRCLE('',#31047,3.05);
#1086=CIRCLE('',#31049,3.05);
#1087=CIRCLE('',#31051,3.05);
#1088=CIRCLE('',#31053,3.05000000000001);
#1089=CIRCLE('',#31055,3.05000000000001);
#1090=CIRCLE('',#31057,3.05);
#1091=CIRCLE('',#31059,3.05);
#1092=CIRCLE('',#31061,3.05000000000001);
#1093=CIRCLE('',#31063,3.05000000000001);
#1094=CIRCLE('',#31065,3.05);
#1095=CIRCLE('',#31067,3.05);
#1096=CIRCLE('',#31069,3.05);
#1097=CIRCLE('',#31071,3.05);
#1098=CIRCLE('',#31073,3.05000000000001);
#1099=CIRCLE('',#31075,3.05000000000001);
#1100=CIRCLE('',#31077,3.05);
#1101=CIRCLE('',#31079,3.05);
#1102=CIRCLE('',#31081,3.05000000000001);
#1103=CIRCLE('',#31083,3.05000000000001);
#1104=CIRCLE('',#31085,3.05);
#1105=CIRCLE('',#31087,3.05);
#1106=CIRCLE('',#31089,7.);
#1107=CIRCLE('',#31092,7.);
#1108=CIRCLE('',#31095,7.);
#1109=CIRCLE('',#31098,7.);
#1110=CIRCLE('',#31119,5.5);
#1872=CONICAL_SURFACE('',#30902,1.8,0.785398163397448);
#1873=CONICAL_SURFACE('',#30909,1.8,0.785398163397448);
#1874=CONICAL_SURFACE('',#30913,4.75,0.785398163397448);
#1875=CONICAL_SURFACE('',#30920,4.75,0.785398163397446);
#1876=CONICAL_SURFACE('',#30927,4.75,0.785398163397446);
#1877=CONICAL_SURFACE('',#30934,4.75,0.785398163397448);
#1878=CONICAL_SURFACE('',#31036,4.25,0.785398163397448);
#1879=CONICAL_SURFACE('',#31040,3.25,0.785398163397448);
#1880=CONICAL_SURFACE('',#31044,3.25,0.785398163397448);
#1881=CONICAL_SURFACE('',#31048,3.25,0.785398163397448);
#1882=CONICAL_SURFACE('',#31052,3.25,0.785398163397437);
#1883=CONICAL_SURFACE('',#31056,3.25,0.785398163397448);
#1884=CONICAL_SURFACE('',#31060,3.25,0.785398163397437);
#1885=CONICAL_SURFACE('',#31064,3.25,0.785398163397448);
#1886=CONICAL_SURFACE('',#31068,3.25,0.785398163397448);
#1887=CONICAL_SURFACE('',#31072,3.25,0.785398163397437);
#1888=CONICAL_SURFACE('',#31076,3.25,0.785398163397448);
#1889=CONICAL_SURFACE('',#31080,3.25,0.785398163397437);
#1890=CONICAL_SURFACE('',#31084,3.25,0.785398163397448);
#1891=CONICAL_SURFACE('',#31088,7.2,0.785398163397448);
#1892=CONICAL_SURFACE('',#31091,7.2,0.785398163397448);
#1893=CONICAL_SURFACE('',#31094,7.2,0.785398163397448);
#1894=CONICAL_SURFACE('',#31097,7.2,0.785398163397448);
#1895=CONICAL_SURFACE('',#31100,4.7,0.785398163397448);
#1896=CONICAL_SURFACE('',#31101,4.7,0.785398163397448);
#1897=CONICAL_SURFACE('',#31102,4.7,0.785398163397448);
#1898=CONICAL_SURFACE('',#31103,4.7,0.785398163397448);
#2083=B_SPLINE_CURVE_WITH_KNOTS('',2,(#40862,#40863,#40864),
 .UNSPECIFIED.,.F.,.F.,(3,3),(0.,1.),.UNSPECIFIED.);
#2084=B_SPLINE_CURVE_WITH_KNOTS('',2,(#40866,#40867,#40868),
 .UNSPECIFIED.,.F.,.F.,(3,3),(0.,1.),.UNSPECIFIED.);
#2085=B_SPLINE_CURVE_WITH_KNOTS('',2,(#40870,#40871,#40872),
 .UNSPECIFIED.,.F.,.F.,(3,3),(0.,1.),.UNSPECIFIED.);
#2086=B_SPLINE_CURVE_WITH_KNOTS('',2,(#40874,#40875,#40876),
 .UNSPECIFIED.,.F.,.F.,(3,3),(0.,1.),.UNSPECIFIED.);
#2087=B_SPLINE_CURVE_WITH_KNOTS('',2,(#40878,#40879,#40880),
 .UNSPECIFIED.,.F.,.F.,(3,3),(0.,1.),.UNSPECIFIED.);
#2088=B_SPLINE_CURVE_WITH_KNOTS('',2,(#40882,#40883,#40884),
 .UNSPECIFIED.,.F.,.F.,(3,3),(0.,1.),.UNSPECIFIED.);
#2089=B_SPLINE_CURVE_WITH_KNOTS('',2,(#40886,#40887,#40888),
 .UNSPECIFIED.,.F.,.F.,(3,3),(0.,1.),.UNSPECIFIED.);
#2090=B_SPLINE_CURVE_WITH_KNOTS('',2,(#40896,#40897,#40898),
 .UNSPECIFIED.,.F.,.F.,(3,3),(0.,1.),.UNSPECIFIED.);
#2091=B_SPLINE_CURVE_WITH_KNOTS('',2,(#40900,#40901,#40902),
 .UNSPECIFIED.,.F.,.F.,(3,3),(0.,1.),.UNSPECIFIED.);
#2092=B_SPLINE_CURVE_WITH_KNOTS('',2,(#40904,#40905,#40906),
 .UNSPECIFIED.,.F.,.F.,(3,3),(0.,1.),.UNSPECIFIED.);
#2093=B_SPLINE_CURVE_WITH_KNOTS('',2,(#40907,#40908,#40909),
 .UNSPECIFIED.,.F.,.F.,(3,3),(0.,1.),.UNSPECIFIED.);
#2094=B_SPLINE_CURVE_WITH_KNOTS('',2,(#40936,#40937,#40938),
 .UNSPECIFIED.,.F.,.F.,(3,3),(0.,1.),.UNSPECIFIED.);
#2095=B_SPLINE_CURVE_WITH_KNOTS('',2,(#40940,#40941,#40942),
 .UNSPECIFIED.,.F.,.F.,(3,3),(0.,1.),.UNSPECIFIED.);
#2096=B_SPLINE_CURVE_WITH_KNOTS('',2,(#40952,#40953,#40954),
 .UNSPECIFIED.,.F.,.F.,(3,3),(0.,1.),.UNSPECIFIED.);
#2097=B_SPLINE_CURVE_WITH_KNOTS('',2,(#40956,#40957,#40958),
 .UNSPECIFIED.,.F.,.F.,(3,3),(0.,1.),.UNSPECIFIED.);
#2098=B_SPLINE_CURVE_WITH_KNOTS('',2,(#40960,#40961,#40962),
 .UNSPECIFIED.,.F.,.F.,(3,3),(0.,1.),.UNSPECIFIED.);
#2099=B_SPLINE_CURVE_WITH_KNOTS('',2,(#40965,#40966,#40967),
 .UNSPECIFIED.,.F.,.F.,(3,3),(0.,1.),.UNSPECIFIED.);
#2100=B_SPLINE_CURVE_WITH_KNOTS('',2,(#40970,#40971,#40972),
 .UNSPECIFIED.,.F.,.F.,(3,3),(0.,1.),.UNSPECIFIED.);
#2101=B_SPLINE_CURVE_WITH_KNOTS('',2,(#40974,#40975,#40976),
 .UNSPECIFIED.,.F.,.F.,(3,3),(0.,1.),.UNSPECIFIED.);
#2102=B_SPLINE_CURVE_WITH_KNOTS('',2,(#40978,#40979,#40980),
 .UNSPECIFIED.,.F.,.F.,(3,3),(0.,1.),.UNSPECIFIED.);
#2103=B_SPLINE_CURVE_WITH_KNOTS('',2,(#40984,#40985,#40986),
 .UNSPECIFIED.,.F.,.F.,(3,3),(0.,1.),.UNSPECIFIED.);
#2104=B_SPLINE_CURVE_WITH_KNOTS('',2,(#40988,#40989,#40990),
 .UNSPECIFIED.,.F.,.F.,(3,3),(0.,1.),.UNSPECIFIED.);
#2105=B_SPLINE_CURVE_WITH_KNOTS('',2,(#40992,#40993,#40994),
 .UNSPECIFIED.,.F.,.F.,(3,3),(0.,1.),.UNSPECIFIED.);
#2106=B_SPLINE_CURVE_WITH_KNOTS('',2,(#40996,#40997,#40998),
 .UNSPECIFIED.,.F.,.F.,(3,3),(0.,1.),.UNSPECIFIED.);
#2107=B_SPLINE_CURVE_WITH_KNOTS('',2,(#41000,#41001,#41002),
 .UNSPECIFIED.,.F.,.F.,(3,3),(0.,1.),.UNSPECIFIED.);
#2108=B_SPLINE_CURVE_WITH_KNOTS('',2,(#41004,#41005,#41006),
 .UNSPECIFIED.,.F.,.F.,(3,3),(0.,1.),.UNSPECIFIED.);
#2109=B_SPLINE_CURVE_WITH_KNOTS('',2,(#41008,#41009,#41010),
 .UNSPECIFIED.,.F.,.F.,(3,3),(0.,1.),.UNSPECIFIED.);
#2110=B_SPLINE_CURVE_WITH_KNOTS('',2,(#41012,#41013,#41014),
 .UNSPECIFIED.,.F.,.F.,(3,3),(0.,1.),.UNSPECIFIED.);
#2111=B_SPLINE_CURVE_WITH_KNOTS('',2,(#41016,#41017,#41018),
 .UNSPECIFIED.,.F.,.F.,(3,3),(0.,1.),.UNSPECIFIED.);
#2112=B_SPLINE_CURVE_WITH_KNOTS('',2,(#41020,#41021,#41022),
 .UNSPECIFIED.,.F.,.F.,(3,3),(0.,1.),.UNSPECIFIED.);
#2113=B_SPLINE_CURVE_WITH_KNOTS('',2,(#41024,#41025,#41026),
 .UNSPECIFIED.,.F.,.F.,(3,3),(0.,1.),.UNSPECIFIED.);
#2114=B_SPLINE_CURVE_WITH_KNOTS('',2,(#41028,#41029,#41030),
 .UNSPECIFIED.,.F.,.F.,(3,3),(0.,1.),.UNSPECIFIED.);
#2115=B_SPLINE_CURVE_WITH_KNOTS('',2,(#41032,#41033,#41034),
 .UNSPECIFIED.,.F.,.F.,(3,3),(0.,1.),.UNSPECIFIED.);
#2116=B_SPLINE_CURVE_WITH_KNOTS('',2,(#41036,#41037,#41038),
 .UNSPECIFIED.,.F.,.F.,(3,3),(0.,1.),.UNSPECIFIED.);
#2117=B_SPLINE_CURVE_WITH_KNOTS('',2,(#41040,#41041,#41042),
 .UNSPECIFIED.,.F.,.F.,(3,3),(0.,1.),.UNSPECIFIED.);
#2118=B_SPLINE_CURVE_WITH_KNOTS('',2,(#41044,#41045,#41046),
 .UNSPECIFIED.,.F.,.F.,(3,3),(0.,1.),.UNSPECIFIED.);
#2119=B_SPLINE_CURVE_WITH_KNOTS('',2,(#41048,#41049,#41050),
 .UNSPECIFIED.,.F.,.F.,(3,3),(0.,1.),.UNSPECIFIED.);
#2120=B_SPLINE_CURVE_WITH_KNOTS('',2,(#41052,#41053,#41054),
 .UNSPECIFIED.,.F.,.F.,(3,3),(0.,1.),.UNSPECIFIED.);
#2121=B_SPLINE_CURVE_WITH_KNOTS('',2,(#41058,#41059,#41060),
 .UNSPECIFIED.,.F.,.F.,(3,3),(0.,1.),.UNSPECIFIED.);
#2122=B_SPLINE_CURVE_WITH_KNOTS('',2,(#41062,#41063,#41064),
 .UNSPECIFIED.,.F.,.F.,(3,3),(0.,1.),.UNSPECIFIED.);
#2123=B_SPLINE_CURVE_WITH_KNOTS('',2,(#41066,#41067,#41068),
 .UNSPECIFIED.,.F.,.F.,(3,3),(0.,1.),.UNSPECIFIED.);
#2124=B_SPLINE_CURVE_WITH_KNOTS('',2,(#41070,#41071,#41072),
 .UNSPECIFIED.,.F.,.F.,(3,3),(0.,1.),.UNSPECIFIED.);
#2125=B_SPLINE_CURVE_WITH_KNOTS('',2,(#41074,#41075,#41076),
 .UNSPECIFIED.,.F.,.F.,(3,3),(0.,1.),.UNSPECIFIED.);
#2126=B_SPLINE_CURVE_WITH_KNOTS('',2,(#41078,#41079,#41080),
 .UNSPECIFIED.,.F.,.F.,(3,3),(0.,1.),.UNSPECIFIED.);
#2127=B_SPLINE_CURVE_WITH_KNOTS('',2,(#41082,#41083,#41084),
 .UNSPECIFIED.,.F.,.F.,(3,3),(0.,1.),.UNSPECIFIED.);
#2128=B_SPLINE_CURVE_WITH_KNOTS('',2,(#41086,#41087,#41088),
 .UNSPECIFIED.,.F.,.F.,(3,3),(0.,1.),.UNSPECIFIED.);
#2129=B_SPLINE_CURVE_WITH_KNOTS('',2,(#41090,#41091,#41092),
 .UNSPECIFIED.,.F.,.F.,(3,3),(0.,1.),.UNSPECIFIED.);
#2130=B_SPLINE_CURVE_WITH_KNOTS('',2,(#41094,#41095,#41096),
 .UNSPECIFIED.,.F.,.F.,(3,3),(0.,1.),.UNSPECIFIED.);
#2131=B_SPLINE_CURVE_WITH_KNOTS('',2,(#41098,#41099,#41100),
 .UNSPECIFIED.,.F.,.F.,(3,3),(0.,1.),.UNSPECIFIED.);
#2132=B_SPLINE_CURVE_WITH_KNOTS('',2,(#41101,#41102,#41103),
 .UNSPECIFIED.,.F.,.F.,(3,3),(0.,1.),.UNSPECIFIED.);
#2133=B_SPLINE_CURVE_WITH_KNOTS('',2,(#41106,#41107,#41108),
 .UNSPECIFIED.,.F.,.F.,(3,3),(0.,1.),.UNSPECIFIED.);
#2134=B_SPLINE_CURVE_WITH_KNOTS('',2,(#41110,#41111,#41112),
 .UNSPECIFIED.,.F.,.F.,(3,3),(0.,1.),.UNSPECIFIED.);
#2135=B_SPLINE_CURVE_WITH_KNOTS('',2,(#41114,#41115,#41116),
 .UNSPECIFIED.,.F.,.F.,(3,3),(0.,1.),.UNSPECIFIED.);
#2136=B_SPLINE_CURVE_WITH_KNOTS('',2,(#41120,#41121,#41122),
 .UNSPECIFIED.,.F.,.F.,(3,3),(0.,1.),.UNSPECIFIED.);
#2137=B_SPLINE_CURVE_WITH_KNOTS('',2,(#41124,#41125,#41126),
 .UNSPECIFIED.,.F.,.F.,(3,3),(0.,1.),.UNSPECIFIED.);
#2138=B_SPLINE_CURVE_WITH_KNOTS('',2,(#41128,#41129,#41130),
 .UNSPECIFIED.,.F.,.F.,(3,3),(0.,1.),.UNSPECIFIED.);
#2139=B_SPLINE_CURVE_WITH_KNOTS('',2,(#41132,#41133,#41134),
 .UNSPECIFIED.,.F.,.F.,(3,3),(0.,1.),.UNSPECIFIED.);
#2140=B_SPLINE_CURVE_WITH_KNOTS('',2,(#41136,#41137,#41138),
 .UNSPECIFIED.,.F.,.F.,(3,3),(0.,1.),.UNSPECIFIED.);
#2141=B_SPLINE_CURVE_WITH_KNOTS('',2,(#41140,#41141,#41142),
 .UNSPECIFIED.,.F.,.F.,(3,3),(0.,1.),.UNSPECIFIED.);
#2142=B_SPLINE_CURVE_WITH_KNOTS('',2,(#41144,#41145,#41146),
 .UNSPECIFIED.,.F.,.F.,(3,3),(0.,1.),.UNSPECIFIED.);
#2143=B_SPLINE_CURVE_WITH_KNOTS('',2,(#41150,#41151,#41152),
 .UNSPECIFIED.,.F.,.F.,(3,3),(0.,1.),.UNSPECIFIED.);
#2144=B_SPLINE_CURVE_WITH_KNOTS('',2,(#41154,#41155,#41156),
 .UNSPECIFIED.,.F.,.F.,(3,3),(0.,1.),.UNSPECIFIED.);
#2145=B_SPLINE_CURVE_WITH_KNOTS('',2,(#41158,#41159,#41160),
 .UNSPECIFIED.,.F.,.F.,(3,3),(0.,1.),.UNSPECIFIED.);
#2146=B_SPLINE_CURVE_WITH_KNOTS('',2,(#41162,#41163,#41164),
 .UNSPECIFIED.,.F.,.F.,(3,3),(0.,1.),.UNSPECIFIED.);
#2147=B_SPLINE_CURVE_WITH_KNOTS('',2,(#41166,#41167,#41168),
 .UNSPECIFIED.,.F.,.F.,(3,3),(0.,1.),.UNSPECIFIED.);
#2148=B_SPLINE_CURVE_WITH_KNOTS('',2,(#41170,#41171,#41172),
 .UNSPECIFIED.,.F.,.F.,(3,3),(0.,1.),.UNSPECIFIED.);
#2149=B_SPLINE_CURVE_WITH_KNOTS('',2,(#41174,#41175,#41176),
 .UNSPECIFIED.,.F.,.F.,(3,3),(0.,1.),.UNSPECIFIED.);
#2150=B_SPLINE_CURVE_WITH_KNOTS('',2,(#41180,#41181,#41182),
 .UNSPECIFIED.,.F.,.F.,(3,3),(0.,1.),.UNSPECIFIED.);
#2151=B_SPLINE_CURVE_WITH_KNOTS('',2,(#41184,#41185,#41186),
 .UNSPECIFIED.,.F.,.F.,(3,3),(0.,1.),.UNSPECIFIED.);
#2152=B_SPLINE_CURVE_WITH_KNOTS('',2,(#41188,#41189,#41190),
 .UNSPECIFIED.,.F.,.F.,(3,3),(0.,1.),.UNSPECIFIED.);
#2153=B_SPLINE_CURVE_WITH_KNOTS('',2,(#41192,#41193,#41194),
 .UNSPECIFIED.,.F.,.F.,(3,3),(0.,1.),.UNSPECIFIED.);
#2154=B_SPLINE_CURVE_WITH_KNOTS('',2,(#41196,#41197,#41198),
 .UNSPECIFIED.,.F.,.F.,(3,3),(0.,1.),.UNSPECIFIED.);
#2155=B_SPLINE_CURVE_WITH_KNOTS('',2,(#41200,#41201,#41202),
 .UNSPECIFIED.,.F.,.F.,(3,3),(0.,1.),.UNSPECIFIED.);
#2156=B_SPLINE_CURVE_WITH_KNOTS('',2,(#41204,#41205,#41206),
 .UNSPECIFIED.,.F.,.F.,(3,3),(0.,1.),.UNSPECIFIED.);
#2157=B_SPLINE_CURVE_WITH_KNOTS('',2,(#41208,#41209,#41210),
 .UNSPECIFIED.,.F.,.F.,(3,3),(0.,1.),.UNSPECIFIED.);
#2158=B_SPLINE_CURVE_WITH_KNOTS('',2,(#41212,#41213,#41214),
 .UNSPECIFIED.,.F.,.F.,(3,3),(0.,1.),.UNSPECIFIED.);
#2159=B_SPLINE_CURVE_WITH_KNOTS('',2,(#41215,#41216,#41217),
 .UNSPECIFIED.,.F.,.F.,(3,3),(0.,1.),.UNSPECIFIED.);
#2160=B_SPLINE_CURVE_WITH_KNOTS('',2,(#41228,#41229,#41230),
 .UNSPECIFIED.,.F.,.F.,(3,3),(0.,1.),.UNSPECIFIED.);
#2161=B_SPLINE_CURVE_WITH_KNOTS('',2,(#41232,#41233,#41234),
 .UNSPECIFIED.,.F.,.F.,(3,3),(0.,1.),.UNSPECIFIED.);
#2162=B_SPLINE_CURVE_WITH_KNOTS('',2,(#41236,#41237,#41238),
 .UNSPECIFIED.,.F.,.F.,(3,3),(0.,1.),.UNSPECIFIED.);
#2163=B_SPLINE_CURVE_WITH_KNOTS('',2,(#41242,#41243,#41244),
 .UNSPECIFIED.,.F.,.F.,(3,3),(0.,1.),.UNSPECIFIED.);
#2164=B_SPLINE_CURVE_WITH_KNOTS('',2,(#41246,#41247,#41248),
 .UNSPECIFIED.,.F.,.F.,(3,3),(0.,1.),.UNSPECIFIED.);
#2165=B_SPLINE_CURVE_WITH_KNOTS('',2,(#41250,#41251,#41252),
 .UNSPECIFIED.,.F.,.F.,(3,3),(0.,1.),.UNSPECIFIED.);
#2166=B_SPLINE_CURVE_WITH_KNOTS('',2,(#41254,#41255,#41256),
 .UNSPECIFIED.,.F.,.F.,(3,3),(0.,1.),.UNSPECIFIED.);
#2167=B_SPLINE_CURVE_WITH_KNOTS('',2,(#41258,#41259,#41260),
 .UNSPECIFIED.,.F.,.F.,(3,3),(0.,1.),.UNSPECIFIED.);
#2168=B_SPLINE_CURVE_WITH_KNOTS('',2,(#41262,#41263,#41264),
 .UNSPECIFIED.,.F.,.F.,(3,3),(0.,1.),.UNSPECIFIED.);
#2169=B_SPLINE_CURVE_WITH_KNOTS('',2,(#41266,#41267,#41268),
 .UNSPECIFIED.,.F.,.F.,(3,3),(0.,1.),.UNSPECIFIED.);
#2170=B_SPLINE_CURVE_WITH_KNOTS('',2,(#41270,#41271,#41272),
 .UNSPECIFIED.,.F.,.F.,(3,3),(0.,1.),.UNSPECIFIED.);
#2171=B_SPLINE_CURVE_WITH_KNOTS('',2,(#41274,#41275,#41276),
 .UNSPECIFIED.,.F.,.F.,(3,3),(0.,1.),.UNSPECIFIED.);
#2172=B_SPLINE_CURVE_WITH_KNOTS('',2,(#41278,#41279,#41280),
 .UNSPECIFIED.,.F.,.F.,(3,3),(0.,1.),.UNSPECIFIED.);
#2173=B_SPLINE_CURVE_WITH_KNOTS('',2,(#41282,#41283,#41284),
 .UNSPECIFIED.,.F.,.F.,(3,3),(0.,1.),.UNSPECIFIED.);
#2174=B_SPLINE_CURVE_WITH_KNOTS('',2,(#41286,#41287,#41288),
 .UNSPECIFIED.,.F.,.F.,(3,3),(0.,1.),.UNSPECIFIED.);
#2175=B_SPLINE_CURVE_WITH_KNOTS('',2,(#41290,#41291,#41292),
 .UNSPECIFIED.,.F.,.F.,(3,3),(0.,1.),.UNSPECIFIED.);
#2176=B_SPLINE_CURVE_WITH_KNOTS('',2,(#41294,#41295,#41296),
 .UNSPECIFIED.,.F.,.F.,(3,3),(0.,1.),.UNSPECIFIED.);
#2177=B_SPLINE_CURVE_WITH_KNOTS('',2,(#41298,#41299,#41300),
 .UNSPECIFIED.,.F.,.F.,(3,3),(0.,1.),.UNSPECIFIED.);
#2178=B_SPLINE_CURVE_WITH_KNOTS('',2,(#41302,#41303,#41304),
 .UNSPECIFIED.,.F.,.F.,(3,3),(0.,1.),.UNSPECIFIED.);
#2179=B_SPLINE_CURVE_WITH_KNOTS('',2,(#41306,#41307,#41308),
 .UNSPECIFIED.,.F.,.F.,(3,3),(0.,1.),.UNSPECIFIED.);
#2180=B_SPLINE_CURVE_WITH_KNOTS('',2,(#41310,#41311,#41312),
 .UNSPECIFIED.,.F.,.F.,(3,3),(0.,1.),.UNSPECIFIED.);
#2181=B_SPLINE_CURVE_WITH_KNOTS('',2,(#41316,#41317,#41318),
 .UNSPECIFIED.,.F.,.F.,(3,3),(0.,1.),.UNSPECIFIED.);
#2182=B_SPLINE_CURVE_WITH_KNOTS('',2,(#41320,#41321,#41322),
 .UNSPECIFIED.,.F.,.F.,(3,3),(0.,1.),.UNSPECIFIED.);
#2183=B_SPLINE_CURVE_WITH_KNOTS('',2,(#41324,#41325,#41326),
 .UNSPECIFIED.,.F.,.F.,(3,3),(0.,1.),.UNSPECIFIED.);
#2184=B_SPLINE_CURVE_WITH_KNOTS('',2,(#41328,#41329,#41330),
 .UNSPECIFIED.,.F.,.F.,(3,3),(0.,1.),.UNSPECIFIED.);
#2185=B_SPLINE_CURVE_WITH_KNOTS('',2,(#41332,#41333,#41334),
 .UNSPECIFIED.,.F.,.F.,(3,3),(0.,1.),.UNSPECIFIED.);
#2186=B_SPLINE_CURVE_WITH_KNOTS('',2,(#41336,#41337,#41338),
 .UNSPECIFIED.,.F.,.F.,(3,3),(0.,1.),.UNSPECIFIED.);
#2187=B_SPLINE_CURVE_WITH_KNOTS('',2,(#41340,#41341,#41342),
 .UNSPECIFIED.,.F.,.F.,(3,3),(0.,1.),.UNSPECIFIED.);
#2188=B_SPLINE_CURVE_WITH_KNOTS('',2,(#41344,#41345,#41346),
 .UNSPECIFIED.,.F.,.F.,(3,3),(0.,1.),.UNSPECIFIED.);
#2189=B_SPLINE_CURVE_WITH_KNOTS('',2,(#41348,#41349,#41350),
 .UNSPECIFIED.,.F.,.F.,(3,3),(0.,1.),.UNSPECIFIED.);
#2190=B_SPLINE_CURVE_WITH_KNOTS('',2,(#41352,#41353,#41354),
 .UNSPECIFIED.,.F.,.F.,(3,3),(0.,1.),.UNSPECIFIED.);
#2191=B_SPLINE_CURVE_WITH_KNOTS('',2,(#41356,#41357,#41358),
 .UNSPECIFIED.,.F.,.F.,(3,3),(0.,1.),.UNSPECIFIED.);
#2192=B_SPLINE_CURVE_WITH_KNOTS('',2,(#41359,#41360,#41361),
 .UNSPECIFIED.,.F.,.F.,(3,3),(0.,1.),.UNSPECIFIED.);
#2193=B_SPLINE_CURVE_WITH_KNOTS('',2,(#41617,#41618,#41619),
 .UNSPECIFIED.,.F.,.F.,(3,3),(0.,1.),.UNSPECIFIED.);
#2194=B_SPLINE_CURVE_WITH_KNOTS('',2,(#41628,#41629,#41630),
 .UNSPECIFIED.,.F.,.F.,(3,3),(0.,1.),.UNSPECIFIED.);
#2195=B_SPLINE_CURVE_WITH_KNOTS('',2,(#41639,#41640,#41641),
 .UNSPECIFIED.,.F.,.F.,(3,3),(0.,1.),.UNSPECIFIED.);
#2196=B_SPLINE_CURVE_WITH_KNOTS('',2,(#41650,#41651,#41652),
 .UNSPECIFIED.,.F.,.F.,(3,3),(0.,1.),.UNSPECIFIED.);
#2197=B_SPLINE_CURVE_WITH_KNOTS('',2,(#41673,#41674,#41675),
 .UNSPECIFIED.,.F.,.F.,(3,3),(0.,1.),.UNSPECIFIED.);
#2198=B_SPLINE_CURVE_WITH_KNOTS('',2,(#41684,#41685,#41686),
 .UNSPECIFIED.,.F.,.F.,(3,3),(0.,1.),.UNSPECIFIED.);
#2199=B_SPLINE_CURVE_WITH_KNOTS('',2,(#41695,#41696,#41697),
 .UNSPECIFIED.,.F.,.F.,(3,3),(0.,1.),.UNSPECIFIED.);
#2200=B_SPLINE_CURVE_WITH_KNOTS('',2,(#41706,#41707,#41708),
 .UNSPECIFIED.,.F.,.F.,(3,3),(0.,1.),.UNSPECIFIED.);
#2201=B_SPLINE_CURVE_WITH_KNOTS('',2,(#41717,#41718,#41719),
 .UNSPECIFIED.,.F.,.F.,(3,3),(0.,1.),.UNSPECIFIED.);
#2202=B_SPLINE_CURVE_WITH_KNOTS('',2,(#41728,#41729,#41730),
 .UNSPECIFIED.,.F.,.F.,(3,3),(0.,1.),.UNSPECIFIED.);
#2203=B_SPLINE_CURVE_WITH_KNOTS('',2,(#41739,#41740,#41741),
 .UNSPECIFIED.,.F.,.F.,(3,3),(0.,1.),.UNSPECIFIED.);
#2204=B_SPLINE_CURVE_WITH_KNOTS('',2,(#41815,#41816,#41817),
 .UNSPECIFIED.,.F.,.F.,(3,3),(0.,1.),.UNSPECIFIED.);
#2205=B_SPLINE_CURVE_WITH_KNOTS('',2,(#41827,#41828,#41829),
 .UNSPECIFIED.,.F.,.F.,(3,3),(0.,1.),.UNSPECIFIED.);
#2206=B_SPLINE_CURVE_WITH_KNOTS('',2,(#41842,#41843,#41844),
 .UNSPECIFIED.,.F.,.F.,(3,3),(0.,1.),.UNSPECIFIED.);
#2207=B_SPLINE_CURVE_WITH_KNOTS('',2,(#41853,#41854,#41855),
 .UNSPECIFIED.,.F.,.F.,(3,3),(0.,1.),.UNSPECIFIED.);
#2208=B_SPLINE_CURVE_WITH_KNOTS('',2,(#41864,#41865,#41866),
 .UNSPECIFIED.,.F.,.F.,(3,3),(0.,1.),.UNSPECIFIED.);
#2209=B_SPLINE_CURVE_WITH_KNOTS('',2,(#41889,#41890,#41891),
 .UNSPECIFIED.,.F.,.F.,(3,3),(0.,1.),.UNSPECIFIED.);
#2210=B_SPLINE_CURVE_WITH_KNOTS('',2,(#41902,#41903,#41904),
 .UNSPECIFIED.,.F.,.F.,(3,3),(0.,1.),.UNSPECIFIED.);
#2211=B_SPLINE_CURVE_WITH_KNOTS('',2,(#41914,#41915,#41916),
 .UNSPECIFIED.,.F.,.F.,(3,3),(0.,1.),.UNSPECIFIED.);
#2212=B_SPLINE_CURVE_WITH_KNOTS('',2,(#41925,#41926,#41927),
 .UNSPECIFIED.,.F.,.F.,(3,3),(0.,1.),.UNSPECIFIED.);
#2213=B_SPLINE_CURVE_WITH_KNOTS('',2,(#41936,#41937,#41938),
 .UNSPECIFIED.,.F.,.F.,(3,3),(0.,1.),.UNSPECIFIED.);
#2214=B_SPLINE_CURVE_WITH_KNOTS('',2,(#41947,#41948,#41949),
 .UNSPECIFIED.,.F.,.F.,(3,3),(0.,1.),.UNSPECIFIED.);
#2215=B_SPLINE_CURVE_WITH_KNOTS('',2,(#41958,#41959,#41960),
 .UNSPECIFIED.,.F.,.F.,(3,3),(0.,1.),.UNSPECIFIED.);
#2216=B_SPLINE_CURVE_WITH_KNOTS('',2,(#41969,#41970,#41971),
 .UNSPECIFIED.,.F.,.F.,(3,3),(0.,1.),.UNSPECIFIED.);
#2217=B_SPLINE_CURVE_WITH_KNOTS('',2,(#41980,#41981,#41982),
 .UNSPECIFIED.,.F.,.F.,(3,3),(0.,1.),.UNSPECIFIED.);
#2218=B_SPLINE_CURVE_WITH_KNOTS('',2,(#41991,#41992,#41993),
 .UNSPECIFIED.,.F.,.F.,(3,3),(0.,1.),.UNSPECIFIED.);
#2219=B_SPLINE_CURVE_WITH_KNOTS('',2,(#42002,#42003,#42004),
 .UNSPECIFIED.,.F.,.F.,(3,3),(0.,1.),.UNSPECIFIED.);
#2220=B_SPLINE_CURVE_WITH_KNOTS('',2,(#42013,#42014,#42015),
 .UNSPECIFIED.,.F.,.F.,(3,3),(0.,1.),.UNSPECIFIED.);
#2221=B_SPLINE_CURVE_WITH_KNOTS('',2,(#42024,#42025,#42026),
 .UNSPECIFIED.,.F.,.F.,(3,3),(0.,1.),.UNSPECIFIED.);
#2222=B_SPLINE_CURVE_WITH_KNOTS('',2,(#42035,#42036,#42037),
 .UNSPECIFIED.,.F.,.F.,(3,3),(0.,1.),.UNSPECIFIED.);
#2223=B_SPLINE_CURVE_WITH_KNOTS('',2,(#42050,#42051,#42052),
 .UNSPECIFIED.,.F.,.F.,(3,3),(0.,1.),.UNSPECIFIED.);
#2224=B_SPLINE_CURVE_WITH_KNOTS('',2,(#42061,#42062,#42063),
 .UNSPECIFIED.,.F.,.F.,(3,3),(0.,1.),.UNSPECIFIED.);
#2225=B_SPLINE_CURVE_WITH_KNOTS('',2,(#42072,#42073,#42074),
 .UNSPECIFIED.,.F.,.F.,(3,3),(0.,1.),.UNSPECIFIED.);
#2226=B_SPLINE_CURVE_WITH_KNOTS('',2,(#42083,#42084,#42085),
 .UNSPECIFIED.,.F.,.F.,(3,3),(0.,1.),.UNSPECIFIED.);
#2227=B_SPLINE_CURVE_WITH_KNOTS('',2,(#42094,#42095,#42096),
 .UNSPECIFIED.,.F.,.F.,(3,3),(0.,1.),.UNSPECIFIED.);
#2228=B_SPLINE_CURVE_WITH_KNOTS('',2,(#42105,#42106,#42107),
 .UNSPECIFIED.,.F.,.F.,(3,3),(0.,1.),.UNSPECIFIED.);
#2229=B_SPLINE_CURVE_WITH_KNOTS('',2,(#42116,#42117,#42118),
 .UNSPECIFIED.,.F.,.F.,(3,3),(0.,1.),.UNSPECIFIED.);
#2230=B_SPLINE_CURVE_WITH_KNOTS('',2,(#42127,#42128,#42129),
 .UNSPECIFIED.,.F.,.F.,(3,3),(0.,1.),.UNSPECIFIED.);
#2231=B_SPLINE_CURVE_WITH_KNOTS('',2,(#42138,#42139,#42140),
 .UNSPECIFIED.,.F.,.F.,(3,3),(0.,1.),.UNSPECIFIED.);
#2232=B_SPLINE_CURVE_WITH_KNOTS('',2,(#42149,#42150,#42151),
 .UNSPECIFIED.,.F.,.F.,(3,3),(0.,1.),.UNSPECIFIED.);
#2233=B_SPLINE_CURVE_WITH_KNOTS('',2,(#42160,#42161,#42162),
 .UNSPECIFIED.,.F.,.F.,(3,3),(0.,1.),.UNSPECIFIED.);
#2234=B_SPLINE_CURVE_WITH_KNOTS('',2,(#42171,#42172,#42173),
 .UNSPECIFIED.,.F.,.F.,(3,3),(0.,1.),.UNSPECIFIED.);
#2235=B_SPLINE_CURVE_WITH_KNOTS('',2,(#42182,#42183,#42184),
 .UNSPECIFIED.,.F.,.F.,(3,3),(0.,1.),.UNSPECIFIED.);
#2236=B_SPLINE_CURVE_WITH_KNOTS('',2,(#42193,#42194,#42195),
 .UNSPECIFIED.,.F.,.F.,(3,3),(0.,1.),.UNSPECIFIED.);
#2237=B_SPLINE_CURVE_WITH_KNOTS('',2,(#42204,#42205,#42206),
 .UNSPECIFIED.,.F.,.F.,(3,3),(0.,1.),.UNSPECIFIED.);
#2238=B_SPLINE_CURVE_WITH_KNOTS('',2,(#42215,#42216,#42217),
 .UNSPECIFIED.,.F.,.F.,(3,3),(0.,1.),.UNSPECIFIED.);
#2239=B_SPLINE_CURVE_WITH_KNOTS('',2,(#42226,#42227,#42228),
 .UNSPECIFIED.,.F.,.F.,(3,3),(0.,1.),.UNSPECIFIED.);
#2240=B_SPLINE_CURVE_WITH_KNOTS('',2,(#42237,#42238,#42239),
 .UNSPECIFIED.,.F.,.F.,(3,3),(0.,1.),.UNSPECIFIED.);
#2241=B_SPLINE_CURVE_WITH_KNOTS('',2,(#42252,#42253,#42254),
 .UNSPECIFIED.,.F.,.F.,(3,3),(0.,1.),.UNSPECIFIED.);
#2242=B_SPLINE_CURVE_WITH_KNOTS('',2,(#42261,#42262,#42263),
 .UNSPECIFIED.,.F.,.F.,(3,3),(0.,1.),.UNSPECIFIED.);
#2243=B_SPLINE_CURVE_WITH_KNOTS('',2,(#42274,#42275,#42276),
 .UNSPECIFIED.,.F.,.F.,(3,3),(0.,1.),.UNSPECIFIED.);
#2244=B_SPLINE_CURVE_WITH_KNOTS('',2,(#42286,#42287,#42288),
 .UNSPECIFIED.,.F.,.F.,(3,3),(0.,1.),.UNSPECIFIED.);
#2245=B_SPLINE_CURVE_WITH_KNOTS('',2,(#42297,#42298,#42299),
 .UNSPECIFIED.,.F.,.F.,(3,3),(0.,1.),.UNSPECIFIED.);
#2246=B_SPLINE_CURVE_WITH_KNOTS('',2,(#42308,#42309,#42310),
 .UNSPECIFIED.,.F.,.F.,(3,3),(0.,1.),.UNSPECIFIED.);
#2247=B_SPLINE_CURVE_WITH_KNOTS('',2,(#42319,#42320,#42321),
 .UNSPECIFIED.,.F.,.F.,(3,3),(0.,1.),.UNSPECIFIED.);
#2248=B_SPLINE_CURVE_WITH_KNOTS('',2,(#42330,#42331,#42332),
 .UNSPECIFIED.,.F.,.F.,(3,3),(0.,1.),.UNSPECIFIED.);
#2249=B_SPLINE_CURVE_WITH_KNOTS('',2,(#42341,#42342,#42343),
 .UNSPECIFIED.,.F.,.F.,(3,3),(0.,1.),.UNSPECIFIED.);
#2250=B_SPLINE_CURVE_WITH_KNOTS('',2,(#42352,#42353,#42354),
 .UNSPECIFIED.,.F.,.F.,(3,3),(0.,1.),.UNSPECIFIED.);
#2251=B_SPLINE_CURVE_WITH_KNOTS('',2,(#42363,#42364,#42365),
 .UNSPECIFIED.,.F.,.F.,(3,3),(0.,1.),.UNSPECIFIED.);
#2252=B_SPLINE_CURVE_WITH_KNOTS('',2,(#42374,#42375,#42376),
 .UNSPECIFIED.,.F.,.F.,(3,3),(0.,1.),.UNSPECIFIED.);
#2253=B_SPLINE_CURVE_WITH_KNOTS('',2,(#42385,#42386,#42387),
 .UNSPECIFIED.,.F.,.F.,(3,3),(0.,1.),.UNSPECIFIED.);
#2254=B_SPLINE_CURVE_WITH_KNOTS('',2,(#42400,#42401,#42402),
 .UNSPECIFIED.,.F.,.F.,(3,3),(0.,1.),.UNSPECIFIED.);
#2255=B_SPLINE_CURVE_WITH_KNOTS('',2,(#42411,#42412,#42413),
 .UNSPECIFIED.,.F.,.F.,(3,3),(0.,1.),.UNSPECIFIED.);
#2256=B_SPLINE_CURVE_WITH_KNOTS('',2,(#42422,#42423,#42424),
 .UNSPECIFIED.,.F.,.F.,(3,3),(0.,1.),.UNSPECIFIED.);
#2257=B_SPLINE_CURVE_WITH_KNOTS('',2,(#42433,#42434,#42435),
 .UNSPECIFIED.,.F.,.F.,(3,3),(0.,1.),.UNSPECIFIED.);
#2258=B_SPLINE_CURVE_WITH_KNOTS('',2,(#42444,#42445,#42446),
 .UNSPECIFIED.,.F.,.F.,(3,3),(0.,1.),.UNSPECIFIED.);
#2259=B_SPLINE_CURVE_WITH_KNOTS('',2,(#42455,#42456,#42457),
 .UNSPECIFIED.,.F.,.F.,(3,3),(0.,1.),.UNSPECIFIED.);
#2260=B_SPLINE_CURVE_WITH_KNOTS('',2,(#42466,#42467,#42468),
 .UNSPECIFIED.,.F.,.F.,(3,3),(0.,1.),.UNSPECIFIED.);
#2261=B_SPLINE_CURVE_WITH_KNOTS('',2,(#42481,#42482,#42483),
 .UNSPECIFIED.,.F.,.F.,(3,3),(0.,1.),.UNSPECIFIED.);
#2262=B_SPLINE_CURVE_WITH_KNOTS('',2,(#42492,#42493,#42494),
 .UNSPECIFIED.,.F.,.F.,(3,3),(0.,1.),.UNSPECIFIED.);
#2263=B_SPLINE_CURVE_WITH_KNOTS('',2,(#42503,#42504,#42505),
 .UNSPECIFIED.,.F.,.F.,(3,3),(0.,1.),.UNSPECIFIED.);
#2264=B_SPLINE_CURVE_WITH_KNOTS('',2,(#42514,#42515,#42516),
 .UNSPECIFIED.,.F.,.F.,(3,3),(0.,1.),.UNSPECIFIED.);
#2265=B_SPLINE_CURVE_WITH_KNOTS('',2,(#42525,#42526,#42527),
 .UNSPECIFIED.,.F.,.F.,(3,3),(0.,1.),.UNSPECIFIED.);
#2266=B_SPLINE_CURVE_WITH_KNOTS('',2,(#42536,#42537,#42538),
 .UNSPECIFIED.,.F.,.F.,(3,3),(0.,1.),.UNSPECIFIED.);
#2267=B_SPLINE_CURVE_WITH_KNOTS('',2,(#42547,#42548,#42549),
 .UNSPECIFIED.,.F.,.F.,(3,3),(0.,1.),.UNSPECIFIED.);
#2268=B_SPLINE_CURVE_WITH_KNOTS('',2,(#42562,#42563,#42564),
 .UNSPECIFIED.,.F.,.F.,(3,3),(0.,1.),.UNSPECIFIED.);
#2269=B_SPLINE_CURVE_WITH_KNOTS('',2,(#42571,#42572,#42573),
 .UNSPECIFIED.,.F.,.F.,(3,3),(0.,1.),.UNSPECIFIED.);
#2270=B_SPLINE_CURVE_WITH_KNOTS('',2,(#42601,#42602,#42603),
 .UNSPECIFIED.,.F.,.F.,(3,3),(0.,1.),.UNSPECIFIED.);
#2271=B_SPLINE_CURVE_WITH_KNOTS('',2,(#42613,#42614,#42615),
 .UNSPECIFIED.,.F.,.F.,(3,3),(0.,1.),.UNSPECIFIED.);
#2272=B_SPLINE_CURVE_WITH_KNOTS('',2,(#42624,#42625,#42626),
 .UNSPECIFIED.,.F.,.F.,(3,3),(0.,1.),.UNSPECIFIED.);
#2273=B_SPLINE_CURVE_WITH_KNOTS('',2,(#42635,#42636,#42637),
 .UNSPECIFIED.,.F.,.F.,(3,3),(0.,1.),.UNSPECIFIED.);
#2274=B_SPLINE_CURVE_WITH_KNOTS('',2,(#42646,#42647,#42648),
 .UNSPECIFIED.,.F.,.F.,(3,3),(0.,1.),.UNSPECIFIED.);
#2275=B_SPLINE_CURVE_WITH_KNOTS('',2,(#42657,#42658,#42659),
 .UNSPECIFIED.,.F.,.F.,(3,3),(0.,1.),.UNSPECIFIED.);
#2276=B_SPLINE_CURVE_WITH_KNOTS('',2,(#42668,#42669,#42670),
 .UNSPECIFIED.,.F.,.F.,(3,3),(0.,1.),.UNSPECIFIED.);
#2277=B_SPLINE_CURVE_WITH_KNOTS('',2,(#42679,#42680,#42681),
 .UNSPECIFIED.,.F.,.F.,(3,3),(0.,1.),.UNSPECIFIED.);
#2278=B_SPLINE_CURVE_WITH_KNOTS('',2,(#42690,#42691,#42692),
 .UNSPECIFIED.,.F.,.F.,(3,3),(0.,1.),.UNSPECIFIED.);
#2279=B_SPLINE_CURVE_WITH_KNOTS('',2,(#42701,#42702,#42703),
 .UNSPECIFIED.,.F.,.F.,(3,3),(0.,1.),.UNSPECIFIED.);
#2280=B_SPLINE_CURVE_WITH_KNOTS('',2,(#42712,#42713,#42714),
 .UNSPECIFIED.,.F.,.F.,(3,3),(0.,1.),.UNSPECIFIED.);
#2281=B_SPLINE_CURVE_WITH_KNOTS('',2,(#42723,#42724,#42725),
 .UNSPECIFIED.,.F.,.F.,(3,3),(0.,1.),.UNSPECIFIED.);
#2282=B_SPLINE_CURVE_WITH_KNOTS('',2,(#42734,#42735,#42736),
 .UNSPECIFIED.,.F.,.F.,(3,3),(0.,1.),.UNSPECIFIED.);
#2283=B_SPLINE_CURVE_WITH_KNOTS('',2,(#42749,#42750,#42751),
 .UNSPECIFIED.,.F.,.F.,(3,3),(0.,1.),.UNSPECIFIED.);
#2284=B_SPLINE_CURVE_WITH_KNOTS('',2,(#42760,#42761,#42762),
 .UNSPECIFIED.,.F.,.F.,(3,3),(0.,1.),.UNSPECIFIED.);
#2285=B_SPLINE_CURVE_WITH_KNOTS('',2,(#42771,#42772,#42773),
 .UNSPECIFIED.,.F.,.F.,(3,3),(0.,1.),.UNSPECIFIED.);
#2286=B_SPLINE_CURVE_WITH_KNOTS('',2,(#42782,#42783,#42784),
 .UNSPECIFIED.,.F.,.F.,(3,3),(0.,1.),.UNSPECIFIED.);
#2287=B_SPLINE_CURVE_WITH_KNOTS('',2,(#42793,#42794,#42795),
 .UNSPECIFIED.,.F.,.F.,(3,3),(0.,1.),.UNSPECIFIED.);
#2288=B_SPLINE_CURVE_WITH_KNOTS('',2,(#42804,#42805,#42806),
 .UNSPECIFIED.,.F.,.F.,(3,3),(0.,1.),.UNSPECIFIED.);
#2289=B_SPLINE_CURVE_WITH_KNOTS('',2,(#42815,#42816,#42817),
 .UNSPECIFIED.,.F.,.F.,(3,3),(0.,1.),.UNSPECIFIED.);
#2290=B_SPLINE_CURVE_WITH_KNOTS('',2,(#42826,#42827,#42828),
 .UNSPECIFIED.,.F.,.F.,(3,3),(0.,1.),.UNSPECIFIED.);
#2291=B_SPLINE_CURVE_WITH_KNOTS('',2,(#42837,#42838,#42839),
 .UNSPECIFIED.,.F.,.F.,(3,3),(0.,1.),.UNSPECIFIED.);
#2292=B_SPLINE_CURVE_WITH_KNOTS('',2,(#42848,#42849,#42850),
 .UNSPECIFIED.,.F.,.F.,(3,3),(0.,1.),.UNSPECIFIED.);
#2293=B_SPLINE_CURVE_WITH_KNOTS('',2,(#42859,#42860,#42861),
 .UNSPECIFIED.,.F.,.F.,(3,3),(0.,1.),.UNSPECIFIED.);
#2294=B_SPLINE_CURVE_WITH_KNOTS('',2,(#42870,#42871,#42872),
 .UNSPECIFIED.,.F.,.F.,(3,3),(0.,1.),.UNSPECIFIED.);
#2295=B_SPLINE_CURVE_WITH_KNOTS('',2,(#42881,#42882,#42883),
 .UNSPECIFIED.,.F.,.F.,(3,3),(0.,1.),.UNSPECIFIED.);
#2296=B_SPLINE_CURVE_WITH_KNOTS('',2,(#42892,#42893,#42894),
 .UNSPECIFIED.,.F.,.F.,(3,3),(0.,1.),.UNSPECIFIED.);
#2297=B_SPLINE_CURVE_WITH_KNOTS('',2,(#42903,#42904,#42905),
 .UNSPECIFIED.,.F.,.F.,(3,3),(0.,1.),.UNSPECIFIED.);
#2298=B_SPLINE_CURVE_WITH_KNOTS('',2,(#42914,#42915,#42916),
 .UNSPECIFIED.,.F.,.F.,(3,3),(0.,1.),.UNSPECIFIED.);
#2299=B_SPLINE_CURVE_WITH_KNOTS('',2,(#42925,#42926,#42927),
 .UNSPECIFIED.,.F.,.F.,(3,3),(0.,1.),.UNSPECIFIED.);
#2300=B_SPLINE_CURVE_WITH_KNOTS('',2,(#42936,#42937,#42938),
 .UNSPECIFIED.,.F.,.F.,(3,3),(0.,1.),.UNSPECIFIED.);
#2301=B_SPLINE_CURVE_WITH_KNOTS('',2,(#42951,#42952,#42953),
 .UNSPECIFIED.,.F.,.F.,(3,3),(0.,1.),.UNSPECIFIED.);
#2302=B_SPLINE_CURVE_WITH_KNOTS('',2,(#42960,#42961,#42962),
 .UNSPECIFIED.,.F.,.F.,(3,3),(0.,1.),.UNSPECIFIED.);
#3284=FACE_BOUND('',#5341,.T.);
#3285=FACE_BOUND('',#5342,.T.);
#3286=FACE_BOUND('',#5343,.T.);
#3287=FACE_BOUND('',#5344,.T.);
#3288=FACE_BOUND('',#5345,.T.);
#3289=FACE_BOUND('',#5346,.T.);
#3290=FACE_BOUND('',#5347,.T.);
#3291=FACE_BOUND('',#5348,.T.);
#3292=FACE_BOUND('',#5353,.T.);
#3293=FACE_BOUND('',#5354,.T.);
#3294=FACE_BOUND('',#5361,.T.);
#3295=FACE_BOUND('',#5365,.T.);
#3296=FACE_BOUND('',#5369,.T.);
#3297=FACE_BOUND('',#5373,.T.);
#3298=FACE_BOUND('',#5389,.T.);
#3299=FACE_BOUND('',#5390,.T.);
#3300=FACE_BOUND('',#5391,.T.);
#3301=FACE_BOUND('',#5392,.T.);
#3302=FACE_BOUND('',#5393,.T.);
#3303=FACE_BOUND('',#5394,.T.);
#3304=FACE_BOUND('',#5395,.T.);
#3305=FACE_BOUND('',#5396,.T.);
#3306=FACE_BOUND('',#5397,.T.);
#3307=FACE_BOUND('',#5398,.T.);
#3308=FACE_BOUND('',#5399,.T.);
#3309=FACE_BOUND('',#5400,.T.);
#3310=FACE_BOUND('',#5401,.T.);
#3311=FACE_BOUND('',#5402,.T.);
#3312=FACE_BOUND('',#5403,.T.);
#3313=FACE_BOUND('',#5404,.T.);
#3314=FACE_BOUND('',#5405,.T.);
#3315=FACE_BOUND('',#5408,.T.);
#3316=FACE_BOUND('',#5409,.T.);
#3317=FACE_BOUND('',#5410,.T.);
#3318=FACE_BOUND('',#5411,.T.);
#3319=FACE_BOUND('',#5412,.T.);
#3320=FACE_BOUND('',#5633,.T.);
#3577=FACE_OUTER_BOUND('',#5333,.T.);
#3578=FACE_OUTER_BOUND('',#5334,.T.);
#3579=FACE_OUTER_BOUND('',#5335,.T.);
#3580=FACE_OUTER_BOUND('',#5336,.T.);
#3581=FACE_OUTER_BOUND('',#5337,.T.);
#3582=FACE_OUTER_BOUND('',#5338,.T.);
#3583=FACE_OUTER_BOUND('',#5339,.T.);
#3584=FACE_OUTER_BOUND('',#5340,.T.);
#3585=FACE_OUTER_BOUND('',#5349,.T.);
#3586=FACE_OUTER_BOUND('',#5350,.T.);
#3587=FACE_OUTER_BOUND('',#5351,.T.);
#3588=FACE_OUTER_BOUND('',#5352,.T.);
#3589=FACE_OUTER_BOUND('',#5355,.T.);
#3590=FACE_OUTER_BOUND('',#5356,.T.);
#3591=FACE_OUTER_BOUND('',#5357,.T.);
#3592=FACE_OUTER_BOUND('',#5358,.T.);
#3593=FACE_OUTER_BOUND('',#5359,.T.);
#3594=FACE_OUTER_BOUND('',#5360,.T.);
#3595=FACE_OUTER_BOUND('',#5362,.T.);
#3596=FACE_OUTER_BOUND('',#5363,.T.);
#3597=FACE_OUTER_BOUND('',#5364,.T.);
#3598=FACE_OUTER_BOUND('',#5366,.T.);
#3599=FACE_OUTER_BOUND('',#5367,.T.);
#3600=FACE_OUTER_BOUND('',#5368,.T.);
#3601=FACE_OUTER_BOUND('',#5370,.T.);
#3602=FACE_OUTER_BOUND('',#5371,.T.);
#3603=FACE_OUTER_BOUND('',#5372,.T.);
#3604=FACE_OUTER_BOUND('',#5374,.T.);
#3605=FACE_OUTER_BOUND('',#5375,.T.);
#3606=FACE_OUTER_BOUND('',#5376,.T.);
#3607=FACE_OUTER_BOUND('',#5377,.T.);
#3608=FACE_OUTER_BOUND('',#5378,.T.);
#3609=FACE_OUTER_BOUND('',#5379,.T.);
#3610=FACE_OUTER_BOUND('',#5380,.T.);
#3611=FACE_OUTER_BOUND('',#5381,.T.);
#3612=FACE_OUTER_BOUND('',#5382,.T.);
#3613=FACE_OUTER_BOUND('',#5383,.T.);
#3614=FACE_OUTER_BOUND('',#5384,.T.);
#3615=FACE_OUTER_BOUND('',#5385,.T.);
#3616=FACE_OUTER_BOUND('',#5386,.T.);
#3617=FACE_OUTER_BOUND('',#5387,.T.);
#3618=FACE_OUTER_BOUND('',#5388,.T.);
#3619=FACE_OUTER_BOUND('',#5406,.T.);
#3620=FACE_OUTER_BOUND('',#5407,.T.);
#3621=FACE_OUTER_BOUND('',#5413,.T.);
#3622=FACE_OUTER_BOUND('',#5414,.T.);
#3623=FACE_OUTER_BOUND('',#5415,.T.);
#3624=FACE_OUTER_BOUND('',#5416,.T.);
#3625=FACE_OUTER_BOUND('',#5417,.T.);
#3626=FACE_OUTER_BOUND('',#5418,.T.);
#3627=FACE_OUTER_BOUND('',#5419,.T.);
#3628=FACE_OUTER_BOUND('',#5420,.T.);
#3629=FACE_OUTER_BOUND('',#5421,.T.);
#3630=FACE_OUTER_BOUND('',#5422,.T.);
#3631=FACE_OUTER_BOUND('',#5423,.T.);
#3632=FACE_OUTER_BOUND('',#5424,.T.);
#3633=FACE_OUTER_BOUND('',#5425,.T.);
#3634=FACE_OUTER_BOUND('',#5426,.T.);
#3635=FACE_OUTER_BOUND('',#5427,.T.);
#3636=FACE_OUTER_BOUND('',#5428,.T.);
#3637=FACE_OUTER_BOUND('',#5429,.T.);
#3638=FACE_OUTER_BOUND('',#5430,.T.);
#3639=FACE_OUTER_BOUND('',#5431,.T.);
#3640=FACE_OUTER_BOUND('',#5432,.T.);
#3641=FACE_OUTER_BOUND('',#5433,.T.);
#3642=FACE_OUTER_BOUND('',#5434,.T.);
#3643=FACE_OUTER_BOUND('',#5435,.T.);
#3644=FACE_OUTER_BOUND('',#5436,.T.);
#3645=FACE_OUTER_BOUND('',#5437,.T.);
#3646=FACE_OUTER_BOUND('',#5438,.T.);
#3647=FACE_OUTER_BOUND('',#5439,.T.);
#3648=FACE_OUTER_BOUND('',#5440,.T.);
#3649=FACE_OUTER_BOUND('',#5441,.T.);
#3650=FACE_OUTER_BOUND('',#5442,.T.);
#3651=FACE_OUTER_BOUND('',#5443,.T.);
#3652=FACE_OUTER_BOUND('',#5444,.T.);
#3653=FACE_OUTER_BOUND('',#5445,.T.);
#3654=FACE_OUTER_BOUND('',#5446,.T.);
#3655=FACE_OUTER_BOUND('',#5447,.T.);
#3656=FACE_OUTER_BOUND('',#5448,.T.);
#3657=FACE_OUTER_BOUND('',#5449,.T.);
#3658=FACE_OUTER_BOUND('',#5450,.T.);
#3659=FACE_OUTER_BOUND('',#5451,.T.);
#3660=FACE_OUTER_BOUND('',#5452,.T.);
#3661=FACE_OUTER_BOUND('',#5453,.T.);
#3662=FACE_OUTER_BOUND('',#5454,.T.);
#3663=FACE_OUTER_BOUND('',#5455,.T.);
#3664=FACE_OUTER_BOUND('',#5456,.T.);
#3665=FACE_OUTER_BOUND('',#5457,.T.);
#3666=FACE_OUTER_BOUND('',#5458,.T.);
#3667=FACE_OUTER_BOUND('',#5459,.T.);
#3668=FACE_OUTER_BOUND('',#5460,.T.);
#3669=FACE_OUTER_BOUND('',#5461,.T.);
#3670=FACE_OUTER_BOUND('',#5462,.T.);
#3671=FACE_OUTER_BOUND('',#5463,.T.);
#3672=FACE_OUTER_BOUND('',#5464,.T.);
#3673=FACE_OUTER_BOUND('',#5465,.T.);
#3674=FACE_OUTER_BOUND('',#5466,.T.);
#3675=FACE_OUTER_BOUND('',#5467,.T.);
#3676=FACE_OUTER_BOUND('',#5468,.T.);
#3677=FACE_OUTER_BOUND('',#5469,.T.);
#3678=FACE_OUTER_BOUND('',#5470,.T.);
#3679=FACE_OUTER_BOUND('',#5471,.T.);
#3680=FACE_OUTER_BOUND('',#5472,.T.);
#3681=FACE_OUTER_BOUND('',#5473,.T.);
#3682=FACE_OUTER_BOUND('',#5474,.T.);
#3683=FACE_OUTER_BOUND('',#5475,.T.);
#3684=FACE_OUTER_BOUND('',#5476,.T.);
#3685=FACE_OUTER_BOUND('',#5477,.T.);
#3686=FACE_OUTER_BOUND('',#5478,.T.);
#3687=FACE_OUTER_BOUND('',#5479,.T.);
#3688=FACE_OUTER_BOUND('',#5480,.T.);
#3689=FACE_OUTER_BOUND('',#5481,.T.);
#3690=FACE_OUTER_BOUND('',#5482,.T.);
#3691=FACE_OUTER_BOUND('',#5483,.T.);
#3692=FACE_OUTER_BOUND('',#5484,.T.);
#3693=FACE_OUTER_BOUND('',#5485,.T.);
#3694=FACE_OUTER_BOUND('',#5486,.T.);
#3695=FACE_OUTER_BOUND('',#5487,.T.);
#3696=FACE_OUTER_BOUND('',#5488,.T.);
#3697=FACE_OUTER_BOUND('',#5489,.T.);
#3698=FACE_OUTER_BOUND('',#5490,.T.);
#3699=FACE_OUTER_BOUND('',#5491,.T.);
#3700=FACE_OUTER_BOUND('',#5492,.T.);
#3701=FACE_OUTER_BOUND('',#5493,.T.);
#3702=FACE_OUTER_BOUND('',#5494,.T.);
#3703=FACE_OUTER_BOUND('',#5495,.T.);
#3704=FACE_OUTER_BOUND('',#5496,.T.);
#3705=FACE_OUTER_BOUND('',#5497,.T.);
#3706=FACE_OUTER_BOUND('',#5498,.T.);
#3707=FACE_OUTER_BOUND('',#5499,.T.);
#3708=FACE_OUTER_BOUND('',#5500,.T.);
#3709=FACE_OUTER_BOUND('',#5501,.T.);
#3710=FACE_OUTER_BOUND('',#5502,.T.);
#3711=FACE_OUTER_BOUND('',#5503,.T.);
#3712=FACE_OUTER_BOUND('',#5504,.T.);
#3713=FACE_OUTER_BOUND('',#5505,.T.);
#3714=FACE_OUTER_BOUND('',#5506,.T.);
#3715=FACE_OUTER_BOUND('',#5507,.T.);
#3716=FACE_OUTER_BOUND('',#5508,.T.);
#3717=FACE_OUTER_BOUND('',#5509,.T.);
#3718=FACE_OUTER_BOUND('',#5510,.T.);
#3719=FACE_OUTER_BOUND('',#5511,.T.);
#3720=FACE_OUTER_BOUND('',#5512,.T.);
#3721=FACE_OUTER_BOUND('',#5513,.T.);
#3722=FACE_OUTER_BOUND('',#5514,.T.);
#3723=FACE_OUTER_BOUND('',#5515,.T.);
#3724=FACE_OUTER_BOUND('',#5516,.T.);
#3725=FACE_OUTER_BOUND('',#5517,.T.);
#3726=FACE_OUTER_BOUND('',#5518,.T.);
#3727=FACE_OUTER_BOUND('',#5519,.T.);
#3728=FACE_OUTER_BOUND('',#5520,.T.);
#3729=FACE_OUTER_BOUND('',#5521,.T.);
#3730=FACE_OUTER_BOUND('',#5522,.T.);
#3731=FACE_OUTER_BOUND('',#5523,.T.);
#3732=FACE_OUTER_BOUND('',#5524,.T.);
#3733=FACE_OUTER_BOUND('',#5525,.T.);
#3734=FACE_OUTER_BOUND('',#5526,.T.);
#3735=FACE_OUTER_BOUND('',#5527,.T.);
#3736=FACE_OUTER_BOUND('',#5528,.T.);
#3737=FACE_OUTER_BOUND('',#5529,.T.);
#3738=FACE_OUTER_BOUND('',#5530,.T.);
#3739=FACE_OUTER_BOUND('',#5531,.T.);
#3740=FACE_OUTER_BOUND('',#5532,.T.);
#3741=FACE_OUTER_BOUND('',#5533,.T.);
#3742=FACE_OUTER_BOUND('',#5534,.T.);
#3743=FACE_OUTER_BOUND('',#5535,.T.);
#3744=FACE_OUTER_BOUND('',#5536,.T.);
#3745=FACE_OUTER_BOUND('',#5537,.T.);
#3746=FACE_OUTER_BOUND('',#5538,.T.);
#3747=FACE_OUTER_BOUND('',#5539,.T.);
#3748=FACE_OUTER_BOUND('',#5540,.T.);
#3749=FACE_OUTER_BOUND('',#5541,.T.);
#3750=FACE_OUTER_BOUND('',#5542,.T.);
#3751=FACE_OUTER_BOUND('',#5543,.T.);
#3752=FACE_OUTER_BOUND('',#5544,.T.);
#3753=FACE_OUTER_BOUND('',#5545,.T.);
#3754=FACE_OUTER_BOUND('',#5546,.T.);
#3755=FACE_OUTER_BOUND('',#5547,.T.);
#3756=FACE_OUTER_BOUND('',#5548,.T.);
#3757=FACE_OUTER_BOUND('',#5549,.T.);
#3758=FACE_OUTER_BOUND('',#5550,.T.);
#3759=FACE_OUTER_BOUND('',#5551,.T.);
#3760=FACE_OUTER_BOUND('',#5552,.T.);
#3761=FACE_OUTER_BOUND('',#5553,.T.);
#3762=FACE_OUTER_BOUND('',#5554,.T.);
#3763=FACE_OUTER_BOUND('',#5555,.T.);
#3764=FACE_OUTER_BOUND('',#5556,.T.);
#3765=FACE_OUTER_BOUND('',#5557,.T.);
#3766=FACE_OUTER_BOUND('',#5558,.T.);
#3767=FACE_OUTER_BOUND('',#5559,.T.);
#3768=FACE_OUTER_BOUND('',#5560,.T.);
#3769=FACE_OUTER_BOUND('',#5561,.T.);
#3770=FACE_OUTER_BOUND('',#5562,.T.);
#3771=FACE_OUTER_BOUND('',#5563,.T.);
#3772=FACE_OUTER_BOUND('',#5564,.T.);
#3773=FACE_OUTER_BOUND('',#5565,.T.);
#3774=FACE_OUTER_BOUND('',#5566,.T.);
#3775=FACE_OUTER_BOUND('',#5567,.T.);
#3776=FACE_OUTER_BOUND('',#5568,.T.);
#3777=FACE_OUTER_BOUND('',#5569,.T.);
#3778=FACE_OUTER_BOUND('',#5570,.T.);
#3779=FACE_OUTER_BOUND('',#5571,.T.);
#3780=FACE_OUTER_BOUND('',#5572,.T.);
#3781=FACE_OUTER_BOUND('',#5573,.T.);
#3782=FACE_OUTER_BOUND('',#5574,.T.);
#3783=FACE_OUTER_BOUND('',#5575,.T.);
#3784=FACE_OUTER_BOUND('',#5576,.T.);
#3785=FACE_OUTER_BOUND('',#5577,.T.);
#3786=FACE_OUTER_BOUND('',#5578,.T.);
#3787=FACE_OUTER_BOUND('',#5579,.T.);
#3788=FACE_OUTER_BOUND('',#5580,.T.);
#3789=FACE_OUTER_BOUND('',#5581,.T.);
#3790=FACE_OUTER_BOUND('',#5582,.T.);
#3791=FACE_OUTER_BOUND('',#5583,.T.);
#3792=FACE_OUTER_BOUND('',#5584,.T.);
#3793=FACE_OUTER_BOUND('',#5585,.T.);
#3794=FACE_OUTER_BOUND('',#5586,.T.);
#3795=FACE_OUTER_BOUND('',#5587,.T.);
#3796=FACE_OUTER_BOUND('',#5588,.T.);
#3797=FACE_OUTER_BOUND('',#5589,.T.);
#3798=FACE_OUTER_BOUND('',#5590,.T.);
#3799=FACE_OUTER_BOUND('',#5591,.T.);
#3800=FACE_OUTER_BOUND('',#5592,.T.);
#3801=FACE_OUTER_BOUND('',#5593,.T.);
#3802=FACE_OUTER_BOUND('',#5594,.T.);
#3803=FACE_OUTER_BOUND('',#5595,.T.);
#3804=FACE_OUTER_BOUND('',#5596,.T.);
#3805=FACE_OUTER_BOUND('',#5597,.T.);
#3806=FACE_OUTER_BOUND('',#5598,.T.);
#3807=FACE_OUTER_BOUND('',#5599,.T.);
#3808=FACE_OUTER_BOUND('',#5600,.T.);
#3809=FACE_OUTER_BOUND('',#5601,.T.);
#3810=FACE_OUTER_BOUND('',#5602,.T.);
#3811=FACE_OUTER_BOUND('',#5603,.T.);
#3812=FACE_OUTER_BOUND('',#5604,.T.);
#3813=FACE_OUTER_BOUND('',#5605,.T.);
#3814=FACE_OUTER_BOUND('',#5606,.T.);
#3815=FACE_OUTER_BOUND('',#5607,.T.);
#3816=FACE_OUTER_BOUND('',#5608,.T.);
#3817=FACE_OUTER_BOUND('',#5609,.T.);
#3818=FACE_OUTER_BOUND('',#5610,.T.);
#3819=FACE_OUTER_BOUND('',#5611,.T.);
#3820=FACE_OUTER_BOUND('',#5612,.T.);
#3821=FACE_OUTER_BOUND('',#5613,.T.);
#3822=FACE_OUTER_BOUND('',#5614,.T.);
#3823=FACE_OUTER_BOUND('',#5615,.T.);
#3824=FACE_OUTER_BOUND('',#5616,.T.);
#3825=FACE_OUTER_BOUND('',#5617,.T.);
#3826=FACE_OUTER_BOUND('',#5618,.T.);
#3827=FACE_OUTER_BOUND('',#5619,.T.);
#3828=FACE_OUTER_BOUND('',#5620,.T.);
#3829=FACE_OUTER_BOUND('',#5621,.T.);
#3830=FACE_OUTER_BOUND('',#5622,.T.);
#3831=FACE_OUTER_BOUND('',#5623,.T.);
#3832=FACE_OUTER_BOUND('',#5624,.T.);
#3833=FACE_OUTER_BOUND('',#5625,.T.);
#3834=FACE_OUTER_BOUND('',#5626,.T.);
#3835=FACE_OUTER_BOUND('',#5627,.T.);
#3836=FACE_OUTER_BOUND('',#5628,.T.);
#3837=FACE_OUTER_BOUND('',#5629,.T.);
#3838=FACE_OUTER_BOUND('',#5630,.T.);
#3839=FACE_OUTER_BOUND('',#5631,.T.);
#3840=FACE_OUTER_BOUND('',#5632,.T.);
#3841=FACE_OUTER_BOUND('',#5634,.T.);
#5333=EDGE_LOOP('',(#19269,#19270,#19271,#19272,#19273,#19274));
#5334=EDGE_LOOP('',(#19275,#19276,#19277,#19278));
#5335=EDGE_LOOP('',(#19279,#19280,#19281,#19282,#19283,#19284));
#5336=EDGE_LOOP('',(#19285,#19286,#19287,#19288,#19289));
#5337=EDGE_LOOP('',(#19290,#19291,#19292,#19293,#19294,#19295));
#5338=EDGE_LOOP('',(#19296,#19297,#19298,#19299,#19300,#19301));
#5339=EDGE_LOOP('',(#19302,#19303,#19304,#19305,#19306,#19307));
#5340=EDGE_LOOP('',(#19308,#19309,#19310,#19311));
#5341=EDGE_LOOP('',(#19312,#19313,#19314,#19315,#19316,#19317,#19318,#19319,
#19320,#19321,#19322,#19323));
#5342=EDGE_LOOP('',(#19324,#19325,#19326,#19327,#19328,#19329,#19330,#19331,
#19332,#19333,#19334,#19335,#19336,#19337,#19338,#19339,#19340,#19341,#19342));
#5343=EDGE_LOOP('',(#19343,#19344,#19345,#19346,#19347,#19348,#19349,#19350,
#19351,#19352,#19353,#19354));
#5344=EDGE_LOOP('',(#19355,#19356,#19357,#19358,#19359,#19360,#19361,#19362,
#19363,#19364,#19365));
#5345=EDGE_LOOP('',(#19366,#19367,#19368,#19369,#19370,#19371,#19372,#19373,
#19374,#19375,#19376,#19377,#19378,#19379,#19380,#19381,#19382,#19383,#19384,
#19385,#19386,#19387,#19388,#19389,#19390,#19391,#19392,#19393,#19394,#19395,
#19396,#19397,#19398,#19399,#19400));
#5346=EDGE_LOOP('',(#19401,#19402,#19403,#19404,#19405,#19406,#19407,#19408,
#19409,#19410,#19411,#19412,#19413,#19414,#19415,#19416,#19417,#19418,#19419,
#19420,#19421,#19422,#19423,#19424,#19425,#19426,#19427,#19428,#19429,#19430));
#5347=EDGE_LOOP('',(#19431,#19432,#19433,#19434));
#5348=EDGE_LOOP('',(#19435,#19436,#19437,#19438,#19439,#19440,#19441,#19442,
#19443,#19444,#19445,#19446,#19447,#19448,#19449,#19450,#19451,#19452,#19453,
#19454,#19455,#19456,#19457,#19458,#19459,#19460,#19461,#19462,#19463,#19464,
#19465,#19466,#19467,#19468,#19469));
#5349=EDGE_LOOP('',(#19470,#19471,#19472,#19473,#19474,#19475));
#5350=EDGE_LOOP('',(#19476,#19477,#19478,#19479,#19480));
#5351=EDGE_LOOP('',(#19481,#19482,#19483,#19484));
#5352=EDGE_LOOP('',(#19485,#19486,#19487,#19488));
#5353=EDGE_LOOP('',(#19489));
#5354=EDGE_LOOP('',(#19490));
#5355=EDGE_LOOP('',(#19491,#19492,#19493,#19494));
#5356=EDGE_LOOP('',(#19495,#19496,#19497,#19498));
#5357=EDGE_LOOP('',(#19499,#19500,#19501,#19502));
#5358=EDGE_LOOP('',(#19503,#19504,#19505,#19506));
#5359=EDGE_LOOP('',(#19507,#19508,#19509,#19510));
#5360=EDGE_LOOP('',(#19511));
#5361=EDGE_LOOP('',(#19512));
#5362=EDGE_LOOP('',(#19513,#19514,#19515,#19516));
#5363=EDGE_LOOP('',(#19517,#19518,#19519,#19520));
#5364=EDGE_LOOP('',(#19521));
#5365=EDGE_LOOP('',(#19522));
#5366=EDGE_LOOP('',(#19523,#19524,#19525,#19526));
#5367=EDGE_LOOP('',(#19527,#19528,#19529,#19530));
#5368=EDGE_LOOP('',(#19531));
#5369=EDGE_LOOP('',(#19532));
#5370=EDGE_LOOP('',(#19533,#19534,#19535,#19536));
#5371=EDGE_LOOP('',(#19537,#19538,#19539,#19540));
#5372=EDGE_LOOP('',(#19541));
#5373=EDGE_LOOP('',(#19542));
#5374=EDGE_LOOP('',(#19543,#19544,#19545,#19546,#19547,#19548));
#5375=EDGE_LOOP('',(#19549,#19550,#19551,#19552,#19553));
#5376=EDGE_LOOP('',(#19554,#19555,#19556));
#5377=EDGE_LOOP('',(#19557,#19558,#19559));
#5378=EDGE_LOOP('',(#19560,#19561,#19562));
#5379=EDGE_LOOP('',(#19563,#19564,#19565));
#5380=EDGE_LOOP('',(#19566,#19567,#19568,#19569));
#5381=EDGE_LOOP('',(#19570,#19571,#19572,#19573));
#5382=EDGE_LOOP('',(#19574,#19575,#19576,#19577));
#5383=EDGE_LOOP('',(#19578,#19579,#19580,#19581,#19582));
#5384=EDGE_LOOP('',(#19583,#19584,#19585,#19586));
#5385=EDGE_LOOP('',(#19587,#19588,#19589,#19590));
#5386=EDGE_LOOP('',(#19591,#19592,#19593,#19594));
#5387=EDGE_LOOP('',(#19595,#19596,#19597,#19598));
#5388=EDGE_LOOP('',(#19599,#19600,#19601,#19602,#19603,#19604));
#5389=EDGE_LOOP('',(#19605));
#5390=EDGE_LOOP('',(#19606));
#5391=EDGE_LOOP('',(#19607));
#5392=EDGE_LOOP('',(#19608));
#5393=EDGE_LOOP('',(#19609));
#5394=EDGE_LOOP('',(#19610));
#5395=EDGE_LOOP('',(#19611));
#5396=EDGE_LOOP('',(#19612));
#5397=EDGE_LOOP('',(#19613));
#5398=EDGE_LOOP('',(#19614));
#5399=EDGE_LOOP('',(#19615));
#5400=EDGE_LOOP('',(#19616));
#5401=EDGE_LOOP('',(#19617));
#5402=EDGE_LOOP('',(#19618));
#5403=EDGE_LOOP('',(#19619));
#5404=EDGE_LOOP('',(#19620));
#5405=EDGE_LOOP('',(#19621));
#5406=EDGE_LOOP('',(#19622,#19623,#19624,#19625));
#5407=EDGE_LOOP('',(#19626,#19627,#19628,#19629,#19630,#19631));
#5408=EDGE_LOOP('',(#19632));
#5409=EDGE_LOOP('',(#19633));
#5410=EDGE_LOOP('',(#19634));
#5411=EDGE_LOOP('',(#19635));
#5412=EDGE_LOOP('',(#19636));
#5413=EDGE_LOOP('',(#19637,#19638,#19639,#19640));
#5414=EDGE_LOOP('',(#19641,#19642,#19643,#19644));
#5415=EDGE_LOOP('',(#19645,#19646,#19647,#19648));
#5416=EDGE_LOOP('',(#19649,#19650,#19651,#19652));
#5417=EDGE_LOOP('',(#19653,#19654,#19655,#19656));
#5418=EDGE_LOOP('',(#19657,#19658,#19659,#19660));
#5419=EDGE_LOOP('',(#19661,#19662,#19663,#19664));
#5420=EDGE_LOOP('',(#19665,#19666,#19667,#19668));
#5421=EDGE_LOOP('',(#19669,#19670,#19671,#19672));
#5422=EDGE_LOOP('',(#19673,#19674,#19675,#19676));
#5423=EDGE_LOOP('',(#19677,#19678,#19679,#19680));
#5424=EDGE_LOOP('',(#19681,#19682,#19683,#19684));
#5425=EDGE_LOOP('',(#19685,#19686,#19687,#19688,#19689,#19690,#19691,#19692,
#19693,#19694,#19695,#19696));
#5426=EDGE_LOOP('',(#19697,#19698,#19699,#19700));
#5427=EDGE_LOOP('',(#19701,#19702,#19703,#19704));
#5428=EDGE_LOOP('',(#19705,#19706,#19707,#19708));
#5429=EDGE_LOOP('',(#19709,#19710,#19711,#19712));
#5430=EDGE_LOOP('',(#19713,#19714,#19715,#19716));
#5431=EDGE_LOOP('',(#19717,#19718,#19719,#19720));
#5432=EDGE_LOOP('',(#19721,#19722,#19723,#19724));
#5433=EDGE_LOOP('',(#19725,#19726,#19727,#19728));
#5434=EDGE_LOOP('',(#19729,#19730,#19731,#19732));
#5435=EDGE_LOOP('',(#19733,#19734,#19735,#19736));
#5436=EDGE_LOOP('',(#19737,#19738,#19739,#19740));
#5437=EDGE_LOOP('',(#19741,#19742,#19743,#19744));
#5438=EDGE_LOOP('',(#19745,#19746,#19747,#19748));
#5439=EDGE_LOOP('',(#19749,#19750,#19751,#19752));
#5440=EDGE_LOOP('',(#19753,#19754,#19755,#19756));
#5441=EDGE_LOOP('',(#19757,#19758,#19759,#19760));
#5442=EDGE_LOOP('',(#19761,#19762,#19763,#19764));
#5443=EDGE_LOOP('',(#19765,#19766,#19767,#19768));
#5444=EDGE_LOOP('',(#19769,#19770,#19771,#19772));
#5445=EDGE_LOOP('',(#19773,#19774,#19775,#19776,#19777,#19778,#19779,#19780,
#19781,#19782,#19783,#19784,#19785,#19786,#19787,#19788,#19789,#19790,#19791));
#5446=EDGE_LOOP('',(#19792,#19793,#19794,#19795));
#5447=EDGE_LOOP('',(#19796,#19797,#19798,#19799));
#5448=EDGE_LOOP('',(#19800,#19801,#19802,#19803));
#5449=EDGE_LOOP('',(#19804,#19805,#19806,#19807));
#5450=EDGE_LOOP('',(#19808,#19809,#19810,#19811));
#5451=EDGE_LOOP('',(#19812,#19813,#19814,#19815));
#5452=EDGE_LOOP('',(#19816,#19817,#19818,#19819));
#5453=EDGE_LOOP('',(#19820,#19821,#19822,#19823));
#5454=EDGE_LOOP('',(#19824,#19825,#19826,#19827));
#5455=EDGE_LOOP('',(#19828,#19829,#19830,#19831));
#5456=EDGE_LOOP('',(#19832,#19833,#19834,#19835));
#5457=EDGE_LOOP('',(#19836,#19837,#19838,#19839));
#5458=EDGE_LOOP('',(#19840,#19841,#19842,#19843,#19844,#19845,#19846,#19847,
#19848,#19849,#19850,#19851));
#5459=EDGE_LOOP('',(#19852,#19853,#19854,#19855));
#5460=EDGE_LOOP('',(#19856,#19857,#19858,#19859));
#5461=EDGE_LOOP('',(#19860,#19861,#19862,#19863));
#5462=EDGE_LOOP('',(#19864,#19865,#19866,#19867));
#5463=EDGE_LOOP('',(#19868,#19869,#19870,#19871));
#5464=EDGE_LOOP('',(#19872,#19873,#19874,#19875));
#5465=EDGE_LOOP('',(#19876,#19877,#19878,#19879));
#5466=EDGE_LOOP('',(#19880,#19881,#19882,#19883));
#5467=EDGE_LOOP('',(#19884,#19885,#19886,#19887));
#5468=EDGE_LOOP('',(#19888,#19889,#19890,#19891));
#5469=EDGE_LOOP('',(#19892,#19893,#19894,#19895));
#5470=EDGE_LOOP('',(#19896,#19897,#19898,#19899,#19900,#19901,#19902,#19903,
#19904,#19905,#19906));
#5471=EDGE_LOOP('',(#19907,#19908,#19909,#19910));
#5472=EDGE_LOOP('',(#19911,#19912,#19913,#19914));
#5473=EDGE_LOOP('',(#19915,#19916,#19917,#19918));
#5474=EDGE_LOOP('',(#19919,#19920,#19921,#19922));
#5475=EDGE_LOOP('',(#19923,#19924,#19925,#19926));
#5476=EDGE_LOOP('',(#19927,#19928,#19929,#19930));
#5477=EDGE_LOOP('',(#19931,#19932,#19933,#19934));
#5478=EDGE_LOOP('',(#19935,#19936,#19937,#19938));
#5479=EDGE_LOOP('',(#19939,#19940,#19941,#19942));
#5480=EDGE_LOOP('',(#19943,#19944,#19945,#19946));
#5481=EDGE_LOOP('',(#19947,#19948,#19949,#19950));
#5482=EDGE_LOOP('',(#19951,#19952,#19953,#19954));
#5483=EDGE_LOOP('',(#19955,#19956,#19957,#19958));
#5484=EDGE_LOOP('',(#19959,#19960,#19961,#19962));
#5485=EDGE_LOOP('',(#19963,#19964,#19965,#19966));
#5486=EDGE_LOOP('',(#19967,#19968,#19969,#19970));
#5487=EDGE_LOOP('',(#19971,#19972,#19973,#19974));
#5488=EDGE_LOOP('',(#19975,#19976,#19977,#19978));
#5489=EDGE_LOOP('',(#19979,#19980,#19981,#19982));
#5490=EDGE_LOOP('',(#19983,#19984,#19985,#19986));
#5491=EDGE_LOOP('',(#19987,#19988,#19989,#19990));
#5492=EDGE_LOOP('',(#19991,#19992,#19993,#19994));
#5493=EDGE_LOOP('',(#19995,#19996,#19997,#19998));
#5494=EDGE_LOOP('',(#19999,#20000,#20001,#20002));
#5495=EDGE_LOOP('',(#20003,#20004,#20005,#20006));
#5496=EDGE_LOOP('',(#20007,#20008,#20009,#20010));
#5497=EDGE_LOOP('',(#20011,#20012,#20013,#20014));
#5498=EDGE_LOOP('',(#20015,#20016,#20017,#20018));
#5499=EDGE_LOOP('',(#20019,#20020,#20021,#20022));
#5500=EDGE_LOOP('',(#20023,#20024,#20025,#20026));
#5501=EDGE_LOOP('',(#20027,#20028,#20029,#20030));
#5502=EDGE_LOOP('',(#20031,#20032,#20033,#20034));
#5503=EDGE_LOOP('',(#20035,#20036,#20037,#20038));
#5504=EDGE_LOOP('',(#20039,#20040,#20041,#20042));
#5505=EDGE_LOOP('',(#20043,#20044,#20045,#20046));
#5506=EDGE_LOOP('',(#20047,#20048,#20049,#20050,#20051,#20052,#20053,#20054,
#20055,#20056,#20057,#20058,#20059,#20060,#20061,#20062,#20063,#20064,#20065,
#20066,#20067,#20068,#20069,#20070,#20071,#20072,#20073,#20074,#20075,#20076,
#20077,#20078,#20079,#20080,#20081));
#5507=EDGE_LOOP('',(#20082,#20083,#20084,#20085));
#5508=EDGE_LOOP('',(#20086,#20087,#20088,#20089));
#5509=EDGE_LOOP('',(#20090,#20091,#20092,#20093));
#5510=EDGE_LOOP('',(#20094,#20095,#20096,#20097));
#5511=EDGE_LOOP('',(#20098,#20099,#20100,#20101));
#5512=EDGE_LOOP('',(#20102,#20103,#20104,#20105));
#5513=EDGE_LOOP('',(#20106,#20107,#20108,#20109));
#5514=EDGE_LOOP('',(#20110,#20111,#20112,#20113));
#5515=EDGE_LOOP('',(#20114,#20115,#20116,#20117));
#5516=EDGE_LOOP('',(#20118,#20119,#20120,#20121));
#5517=EDGE_LOOP('',(#20122,#20123,#20124,#20125));
#5518=EDGE_LOOP('',(#20126,#20127,#20128,#20129));
#5519=EDGE_LOOP('',(#20130,#20131,#20132,#20133));
#5520=EDGE_LOOP('',(#20134,#20135,#20136,#20137));
#5521=EDGE_LOOP('',(#20138,#20139,#20140,#20141));
#5522=EDGE_LOOP('',(#20142,#20143,#20144,#20145));
#5523=EDGE_LOOP('',(#20146,#20147,#20148,#20149));
#5524=EDGE_LOOP('',(#20150,#20151,#20152,#20153));
#5525=EDGE_LOOP('',(#20154,#20155,#20156,#20157));
#5526=EDGE_LOOP('',(#20158,#20159,#20160,#20161));
#5527=EDGE_LOOP('',(#20162,#20163,#20164,#20165));
#5528=EDGE_LOOP('',(#20166,#20167,#20168,#20169));
#5529=EDGE_LOOP('',(#20170,#20171,#20172,#20173));
#5530=EDGE_LOOP('',(#20174,#20175,#20176,#20177));
#5531=EDGE_LOOP('',(#20178,#20179,#20180,#20181));
#5532=EDGE_LOOP('',(#20182,#20183,#20184,#20185));
#5533=EDGE_LOOP('',(#20186,#20187,#20188,#20189));
#5534=EDGE_LOOP('',(#20190,#20191,#20192,#20193));
#5535=EDGE_LOOP('',(#20194,#20195,#20196,#20197));
#5536=EDGE_LOOP('',(#20198,#20199,#20200,#20201));
#5537=EDGE_LOOP('',(#20202,#20203,#20204,#20205,#20206,#20207,#20208,#20209,
#20210,#20211,#20212,#20213,#20214,#20215,#20216,#20217,#20218,#20219,#20220,
#20221,#20222,#20223,#20224,#20225,#20226,#20227,#20228,#20229,#20230,#20231));
#5538=EDGE_LOOP('',(#20232,#20233,#20234,#20235));
#5539=EDGE_LOOP('',(#20236,#20237,#20238,#20239));
#5540=EDGE_LOOP('',(#20240,#20241,#20242,#20243));
#5541=EDGE_LOOP('',(#20244,#20245,#20246,#20247));
#5542=EDGE_LOOP('',(#20248,#20249,#20250,#20251));
#5543=EDGE_LOOP('',(#20252,#20253,#20254,#20255));
#5544=EDGE_LOOP('',(#20256,#20257,#20258,#20259));
#5545=EDGE_LOOP('',(#20260,#20261,#20262,#20263));
#5546=EDGE_LOOP('',(#20264,#20265,#20266,#20267));
#5547=EDGE_LOOP('',(#20268,#20269,#20270,#20271));
#5548=EDGE_LOOP('',(#20272,#20273,#20274,#20275));
#5549=EDGE_LOOP('',(#20276,#20277,#20278,#20279));
#5550=EDGE_LOOP('',(#20280,#20281,#20282,#20283));
#5551=EDGE_LOOP('',(#20284,#20285,#20286,#20287));
#5552=EDGE_LOOP('',(#20288,#20289,#20290,#20291));
#5553=EDGE_LOOP('',(#20292,#20293,#20294,#20295));
#5554=EDGE_LOOP('',(#20296,#20297,#20298,#20299));
#5555=EDGE_LOOP('',(#20300,#20301,#20302,#20303));
#5556=EDGE_LOOP('',(#20304,#20305,#20306,#20307));
#5557=EDGE_LOOP('',(#20308,#20309,#20310,#20311));
#5558=EDGE_LOOP('',(#20312,#20313,#20314,#20315));
#5559=EDGE_LOOP('',(#20316,#20317,#20318,#20319));
#5560=EDGE_LOOP('',(#20320,#20321,#20322,#20323));
#5561=EDGE_LOOP('',(#20324,#20325,#20326,#20327));
#5562=EDGE_LOOP('',(#20328,#20329,#20330,#20331));
#5563=EDGE_LOOP('',(#20332,#20333,#20334,#20335));
#5564=EDGE_LOOP('',(#20336,#20337,#20338,#20339));
#5565=EDGE_LOOP('',(#20340,#20341,#20342,#20343));
#5566=EDGE_LOOP('',(#20344,#20345,#20346,#20347));
#5567=EDGE_LOOP('',(#20348,#20349,#20350,#20351));
#5568=EDGE_LOOP('',(#20352,#20353,#20354,#20355));
#5569=EDGE_LOOP('',(#20356,#20357,#20358,#20359));
#5570=EDGE_LOOP('',(#20360,#20361,#20362,#20363));
#5571=EDGE_LOOP('',(#20364,#20365,#20366,#20367));
#5572=EDGE_LOOP('',(#20368,#20369,#20370,#20371));
#5573=EDGE_LOOP('',(#20372,#20373,#20374,#20375));
#5574=EDGE_LOOP('',(#20376,#20377,#20378,#20379));
#5575=EDGE_LOOP('',(#20380,#20381,#20382,#20383));
#5576=EDGE_LOOP('',(#20384,#20385,#20386,#20387));
#5577=EDGE_LOOP('',(#20388,#20389,#20390,#20391));
#5578=EDGE_LOOP('',(#20392,#20393,#20394,#20395,#20396,#20397,#20398,#20399,
#20400,#20401,#20402,#20403,#20404,#20405,#20406,#20407,#20408,#20409,#20410,
#20411,#20412,#20413,#20414,#20415,#20416,#20417,#20418,#20419,#20420,#20421,
#20422,#20423,#20424,#20425,#20426));
#5579=EDGE_LOOP('',(#20427,#20428,#20429,#20430));
#5580=EDGE_LOOP('',(#20431,#20432,#20433,#20434));
#5581=EDGE_LOOP('',(#20435,#20436,#20437,#20438));
#5582=EDGE_LOOP('',(#20439,#20440,#20441,#20442));
#5583=EDGE_LOOP('',(#20443,#20444,#20445,#20446));
#5584=EDGE_LOOP('',(#20447,#20448,#20449,#20450));
#5585=EDGE_LOOP('',(#20451,#20452,#20453,#20454));
#5586=EDGE_LOOP('',(#20455,#20456,#20457,#20458));
#5587=EDGE_LOOP('',(#20459,#20460,#20461,#20462));
#5588=EDGE_LOOP('',(#20463,#20464,#20465,#20466));
#5589=EDGE_LOOP('',(#20467,#20468,#20469,#20470));
#5590=EDGE_LOOP('',(#20471,#20472,#20473,#20474));
#5591=EDGE_LOOP('',(#20475,#20476,#20477,#20478));
#5592=EDGE_LOOP('',(#20479,#20480,#20481,#20482));
#5593=EDGE_LOOP('',(#20483,#20484,#20485,#20486));
#5594=EDGE_LOOP('',(#20487,#20488,#20489,#20490));
#5595=EDGE_LOOP('',(#20491,#20492,#20493,#20494));
#5596=EDGE_LOOP('',(#20495,#20496,#20497,#20498));
#5597=EDGE_LOOP('',(#20499,#20500,#20501,#20502));
#5598=EDGE_LOOP('',(#20503,#20504,#20505,#20506));
#5599=EDGE_LOOP('',(#20507,#20508,#20509,#20510));
#5600=EDGE_LOOP('',(#20511,#20512,#20513,#20514));
#5601=EDGE_LOOP('',(#20515,#20516,#20517,#20518));
#5602=EDGE_LOOP('',(#20519,#20520,#20521,#20522));
#5603=EDGE_LOOP('',(#20523,#20524,#20525,#20526));
#5604=EDGE_LOOP('',(#20527,#20528,#20529,#20530));
#5605=EDGE_LOOP('',(#20531,#20532,#20533,#20534));
#5606=EDGE_LOOP('',(#20535,#20536,#20537,#20538));
#5607=EDGE_LOOP('',(#20539,#20540,#20541,#20542));
#5608=EDGE_LOOP('',(#20543,#20544,#20545,#20546));
#5609=EDGE_LOOP('',(#20547,#20548,#20549,#20550));
#5610=EDGE_LOOP('',(#20551,#20552,#20553,#20554));
#5611=EDGE_LOOP('',(#20555,#20556,#20557,#20558));
#5612=EDGE_LOOP('',(#20559,#20560,#20561,#20562));
#5613=EDGE_LOOP('',(#20563,#20564,#20565,#20566));
#5614=EDGE_LOOP('',(#20567,#20568,#20569,#20570));
#5615=EDGE_LOOP('',(#20571,#20572,#20573,#20574));
#5616=EDGE_LOOP('',(#20575,#20576,#20577,#20578));
#5617=EDGE_LOOP('',(#20579));
#5618=EDGE_LOOP('',(#20580));
#5619=EDGE_LOOP('',(#20581));
#5620=EDGE_LOOP('',(#20582));
#5621=EDGE_LOOP('',(#20583));
#5622=EDGE_LOOP('',(#20584));
#5623=EDGE_LOOP('',(#20585));
#5624=EDGE_LOOP('',(#20586));
#5625=EDGE_LOOP('',(#20587));
#5626=EDGE_LOOP('',(#20588));
#5627=EDGE_LOOP('',(#20589));
#5628=EDGE_LOOP('',(#20590));
#5629=EDGE_LOOP('',(#20591));
#5630=EDGE_LOOP('',(#20592));
#5631=EDGE_LOOP('',(#20593,#20594,#20595,#20596));
#5632=EDGE_LOOP('',(#20597));
#5633=EDGE_LOOP('',(#20598));
#5634=EDGE_LOOP('',(#20599,#20600,#20601,#20602));
#7382=LINE('',#40770,#9688);
#7383=LINE('',#40772,#9689);
#7384=LINE('',#40774,#9690);
#7385=LINE('',#40776,#9691);
#7386=LINE('',#40778,#9692);
#7387=LINE('',#40779,#9693);
#7388=LINE('',#40782,#9694);
#7389=LINE('',#40784,#9695);
#7390=LINE('',#40785,#9696);
#7391=LINE('',#40788,#9697);
#7392=LINE('',#40790,#9698);
#7393=LINE('',#40792,#9699);
#7394=LINE('',#40793,#9700);
#7395=LINE('',#40796,#9701);
#7396=LINE('',#40798,#9702);
#7397=LINE('',#40799,#9703);
#7398=LINE('',#40802,#9704);
#7399=LINE('',#40804,#9705);
#7400=LINE('',#40806,#9706);
#7401=LINE('',#40807,#9707);
#7402=LINE('',#40810,#9708);
#7403=LINE('',#40812,#9709);
#7404=LINE('',#40813,#9710);
#7405=LINE('',#40816,#9711);
#7406=LINE('',#40818,#9712);
#7407=LINE('',#40820,#9713);
#7408=LINE('',#40821,#9714);
#7409=LINE('',#40824,#9715);
#7410=LINE('',#40825,#9716);
#7411=LINE('',#40828,#9717);
#7412=LINE('',#40830,#9718);
#7413=LINE('',#40832,#9719);
#7414=LINE('',#40834,#9720);
#7415=LINE('',#40836,#9721);
#7416=LINE('',#40838,#9722);
#7417=LINE('',#40840,#9723);
#7418=LINE('',#40842,#9724);
#7419=LINE('',#40844,#9725);
#7420=LINE('',#40846,#9726);
#7421=LINE('',#40848,#9727);
#7422=LINE('',#40849,#9728);
#7423=LINE('',#40852,#9729);
#7424=LINE('',#40854,#9730);
#7425=LINE('',#40856,#9731);
#7426=LINE('',#40858,#9732);
#7427=LINE('',#40860,#9733);
#7428=LINE('',#40890,#9734);
#7429=LINE('',#40892,#9735);
#7430=LINE('',#40894,#9736);
#7431=LINE('',#40912,#9737);
#7432=LINE('',#40914,#9738);
#7433=LINE('',#40916,#9739);
#7434=LINE('',#40918,#9740);
#7435=LINE('',#40920,#9741);
#7436=LINE('',#40922,#9742);
#7437=LINE('',#40924,#9743);
#7438=LINE('',#40926,#9744);
#7439=LINE('',#40928,#9745);
#7440=LINE('',#40930,#9746);
#7441=LINE('',#40932,#9747);
#7442=LINE('',#40933,#9748);
#7443=LINE('',#40944,#9749);
#7444=LINE('',#40946,#9750);
#7445=LINE('',#40948,#9751);
#7446=LINE('',#40950,#9752);
#7447=LINE('',#40964,#9753);
#7448=LINE('',#40982,#9754);
#7449=LINE('',#41056,#9755);
#7450=LINE('',#41118,#9756);
#7451=LINE('',#41148,#9757);
#7452=LINE('',#41178,#9758);
#7453=LINE('',#41220,#9759);
#7454=LINE('',#41222,#9760);
#7455=LINE('',#41224,#9761);
#7456=LINE('',#41225,#9762);
#7457=LINE('',#41240,#9763);
#7458=LINE('',#41314,#9764);
#7459=LINE('',#41365,#9765);
#7460=LINE('',#41367,#9766);
#7461=LINE('',#41368,#9767);
#7462=LINE('',#41369,#9768);
#7463=LINE('',#41372,#9769);
#7464=LINE('',#41374,#9770);
#7465=LINE('',#41375,#9771);
#7466=LINE('',#41380,#9772);
#7467=LINE('',#41385,#9773);
#7468=LINE('',#41387,#9774);
#7469=LINE('',#41388,#9775);
#7470=LINE('',#41389,#9776);
#7471=LINE('',#41394,#9777);
#7472=LINE('',#41398,#9778);
#7473=LINE('',#41402,#9779);
#7474=LINE('',#41408,#9780);
#7475=LINE('',#41412,#9781);
#7476=LINE('',#41421,#9782);
#7477=LINE('',#41425,#9783);
#7478=LINE('',#41434,#9784);
#7479=LINE('',#41438,#9785);
#7480=LINE('',#41447,#9786);
#7481=LINE('',#41451,#9787);
#7482=LINE('',#41458,#9788);
#7483=LINE('',#41459,#9789);
#7484=LINE('',#41462,#9790);
#7485=LINE('',#41463,#9791);
#7486=LINE('',#41464,#9792);
#7487=LINE('',#41467,#9793);
#7488=LINE('',#41468,#9794);
#7489=LINE('',#41472,#9795);
#7490=LINE('',#41473,#9796);
#7491=LINE('',#41474,#9797);
#7492=LINE('',#41478,#9798);
#7493=LINE('',#41480,#9799);
#7494=LINE('',#41481,#9800);
#7495=LINE('',#41484,#9801);
#7496=LINE('',#41486,#9802);
#7497=LINE('',#41487,#9803);
#7498=LINE('',#41489,#9804);
#7499=LINE('',#41490,#9805);
#7500=LINE('',#41492,#9806);
#7501=LINE('',#41494,#9807);
#7502=LINE('',#41496,#9808);
#7503=LINE('',#41497,#9809);
#7504=LINE('',#41499,#9810);
#7505=LINE('',#41500,#9811);
#7506=LINE('',#41502,#9812);
#7507=LINE('',#41504,#9813);
#7508=LINE('',#41505,#9814);
#7509=LINE('',#41556,#9815);
#7510=LINE('',#41558,#9816);
#7511=LINE('',#41559,#9817);
#7512=LINE('',#41562,#9818);
#7513=LINE('',#41563,#9819);
#7514=LINE('',#41566,#9820);
#7515=LINE('',#41567,#9821);
#7516=LINE('',#41570,#9822);
#7517=LINE('',#41571,#9823);
#7518=LINE('',#41574,#9824);
#7519=LINE('',#41575,#9825);
#7520=LINE('',#41578,#9826);
#7521=LINE('',#41579,#9827);
#7522=LINE('',#41582,#9828);
#7523=LINE('',#41583,#9829);
#7524=LINE('',#41586,#9830);
#7525=LINE('',#41587,#9831);
#7526=LINE('',#41590,#9832);
#7527=LINE('',#41591,#9833);
#7528=LINE('',#41594,#9834);
#7529=LINE('',#41595,#9835);
#7530=LINE('',#41598,#9836);
#7531=LINE('',#41599,#9837);
#7532=LINE('',#41601,#9838);
#7533=LINE('',#41605,#9839);
#7534=LINE('',#41607,#9840);
#7535=LINE('',#41608,#9841);
#7536=LINE('',#41616,#9842);
#7537=LINE('',#41627,#9843);
#7538=LINE('',#41638,#9844);
#7539=LINE('',#41649,#9845);
#7540=LINE('',#41655,#9846);
#7541=LINE('',#41656,#9847);
#7542=LINE('',#41659,#9848);
#7543=LINE('',#41660,#9849);
#7544=LINE('',#41663,#9850);
#7545=LINE('',#41664,#9851);
#7546=LINE('',#41672,#9852);
#7547=LINE('',#41683,#9853);
#7548=LINE('',#41694,#9854);
#7549=LINE('',#41705,#9855);
#7550=LINE('',#41716,#9856);
#7551=LINE('',#41727,#9857);
#7552=LINE('',#41738,#9858);
#7553=LINE('',#41744,#9859);
#7554=LINE('',#41745,#9860);
#7555=LINE('',#41748,#9861);
#7556=LINE('',#41749,#9862);
#7557=LINE('',#41752,#9863);
#7558=LINE('',#41753,#9864);
#7559=LINE('',#41755,#9865);
#7560=LINE('',#41759,#9866);
#7561=LINE('',#41761,#9867);
#7562=LINE('',#41762,#9868);
#7563=LINE('',#41765,#9869);
#7564=LINE('',#41766,#9870);
#7565=LINE('',#41769,#9871);
#7566=LINE('',#41770,#9872);
#7567=LINE('',#41773,#9873);
#7568=LINE('',#41774,#9874);
#7569=LINE('',#41777,#9875);
#7570=LINE('',#41778,#9876);
#7571=LINE('',#41781,#9877);
#7572=LINE('',#41782,#9878);
#7573=LINE('',#41785,#9879);
#7574=LINE('',#41786,#9880);
#7575=LINE('',#41789,#9881);
#7576=LINE('',#41790,#9882);
#7577=LINE('',#41793,#9883);
#7578=LINE('',#41794,#9884);
#7579=LINE('',#41797,#9885);
#7580=LINE('',#41798,#9886);
#7581=LINE('',#41801,#9887);
#7582=LINE('',#41802,#9888);
#7583=LINE('',#41804,#9889);
#7584=LINE('',#41813,#9890);
#7585=LINE('',#41818,#9891);
#7586=LINE('',#41826,#9892);
#7587=LINE('',#41832,#9893);
#7588=LINE('',#41833,#9894);
#7589=LINE('',#41841,#9895);
#7590=LINE('',#41852,#9896);
#7591=LINE('',#41863,#9897);
#7592=LINE('',#41869,#9898);
#7593=LINE('',#41870,#9899);
#7594=LINE('',#41873,#9900);
#7595=LINE('',#41874,#9901);
#7596=LINE('',#41877,#9902);
#7597=LINE('',#41878,#9903);
#7598=LINE('',#41881,#9904);
#7599=LINE('',#41882,#9905);
#7600=LINE('',#41900,#9906);
#7601=LINE('',#41905,#9907);
#7602=LINE('',#41913,#9908);
#7603=LINE('',#41924,#9909);
#7604=LINE('',#41935,#9910);
#7605=LINE('',#41946,#9911);
#7606=LINE('',#41957,#9912);
#7607=LINE('',#41968,#9913);
#7608=LINE('',#41979,#9914);
#7609=LINE('',#41990,#9915);
#7610=LINE('',#42001,#9916);
#7611=LINE('',#42012,#9917);
#7612=LINE('',#42023,#9918);
#7613=LINE('',#42034,#9919);
#7614=LINE('',#42040,#9920);
#7615=LINE('',#42041,#9921);
#7616=LINE('',#42049,#9922);
#7617=LINE('',#42060,#9923);
#7618=LINE('',#42071,#9924);
#7619=LINE('',#42082,#9925);
#7620=LINE('',#42093,#9926);
#7621=LINE('',#42104,#9927);
#7622=LINE('',#42115,#9928);
#7623=LINE('',#42126,#9929);
#7624=LINE('',#42137,#9930);
#7625=LINE('',#42148,#9931);
#7626=LINE('',#42159,#9932);
#7627=LINE('',#42170,#9933);
#7628=LINE('',#42181,#9934);
#7629=LINE('',#42192,#9935);
#7630=LINE('',#42203,#9936);
#7631=LINE('',#42214,#9937);
#7632=LINE('',#42225,#9938);
#7633=LINE('',#42236,#9939);
#7634=LINE('',#42242,#9940);
#7635=LINE('',#42243,#9941);
#7636=LINE('',#42251,#9942);
#7637=LINE('',#42272,#9943);
#7638=LINE('',#42277,#9944);
#7639=LINE('',#42285,#9945);
#7640=LINE('',#42296,#9946);
#7641=LINE('',#42307,#9947);
#7642=LINE('',#42318,#9948);
#7643=LINE('',#42329,#9949);
#7644=LINE('',#42340,#9950);
#7645=LINE('',#42351,#9951);
#7646=LINE('',#42362,#9952);
#7647=LINE('',#42373,#9953);
#7648=LINE('',#42384,#9954);
#7649=LINE('',#42390,#9955);
#7650=LINE('',#42391,#9956);
#7651=LINE('',#42399,#9957);
#7652=LINE('',#42410,#9958);
#7653=LINE('',#42421,#9959);
#7654=LINE('',#42432,#9960);
#7655=LINE('',#42443,#9961);
#7656=LINE('',#42454,#9962);
#7657=LINE('',#42465,#9963);
#7658=LINE('',#42471,#9964);
#7659=LINE('',#42472,#9965);
#7660=LINE('',#42480,#9966);
#7661=LINE('',#42491,#9967);
#7662=LINE('',#42502,#9968);
#7663=LINE('',#42513,#9969);
#7664=LINE('',#42524,#9970);
#7665=LINE('',#42535,#9971);
#7666=LINE('',#42546,#9972);
#7667=LINE('',#42552,#9973);
#7668=LINE('',#42553,#9974);
#7669=LINE('',#42561,#9975);
#7670=LINE('',#42577,#9976);
#7671=LINE('',#42579,#9977);
#7672=LINE('',#42580,#9978);
#7673=LINE('',#42583,#9979);
#7674=LINE('',#42584,#9980);
#7675=LINE('',#42587,#9981);
#7676=LINE('',#42588,#9982);
#7677=LINE('',#42590,#9983);
#7678=LINE('',#42599,#9984);
#7679=LINE('',#42604,#9985);
#7680=LINE('',#42612,#9986);
#7681=LINE('',#42623,#9987);
#7682=LINE('',#42634,#9988);
#7683=LINE('',#42645,#9989);
#7684=LINE('',#42656,#9990);
#7685=LINE('',#42667,#9991);
#7686=LINE('',#42678,#9992);
#7687=LINE('',#42689,#9993);
#7688=LINE('',#42700,#9994);
#7689=LINE('',#42711,#9995);
#7690=LINE('',#42722,#9996);
#7691=LINE('',#42733,#9997);
#7692=LINE('',#42739,#9998);
#7693=LINE('',#42740,#9999);
#7694=LINE('',#42748,#10000);
#7695=LINE('',#42759,#10001);
#7696=LINE('',#42770,#10002);
#7697=LINE('',#42781,#10003);
#7698=LINE('',#42792,#10004);
#7699=LINE('',#42803,#10005);
#7700=LINE('',#42814,#10006);
#7701=LINE('',#42825,#10007);
#7702=LINE('',#42836,#10008);
#7703=LINE('',#42847,#10009);
#7704=LINE('',#42858,#10010);
#7705=LINE('',#42869,#10011);
#7706=LINE('',#42880,#10012);
#7707=LINE('',#42891,#10013);
#7708=LINE('',#42902,#10014);
#7709=LINE('',#42913,#10015);
#7710=LINE('',#42924,#10016);
#7711=LINE('',#42935,#10017);
#7712=LINE('',#42941,#10018);
#7713=LINE('',#42942,#10019);
#7714=LINE('',#42950,#10020);
#7715=LINE('',#42966,#10021);
#7716=LINE('',#42971,#10022);
#7717=LINE('',#42974,#10023);
#7718=LINE('',#42978,#10024);
#7719=LINE('',#42982,#10025);
#7720=LINE('',#42986,#10026);
#7721=LINE('',#42990,#10027);
#7722=LINE('',#42994,#10028);
#7723=LINE('',#42998,#10029);
#7724=LINE('',#43002,#10030);
#7725=LINE('',#43006,#10031);
#7726=LINE('',#43010,#10032);
#7727=LINE('',#43014,#10033);
#7728=LINE('',#43018,#10034);
#7729=LINE('',#43022,#10035);
#7730=LINE('',#43026,#10036);
#7731=LINE('',#43030,#10037);
#7732=LINE('',#43034,#10038);
#7733=LINE('',#43038,#10039);
#7734=LINE('',#43042,#10040);
#7735=LINE('',#43046,#10041);
#7736=LINE('',#43050,#10042);
#7737=LINE('',#43054,#10043);
#7738=LINE('',#43058,#10044);
#7739=LINE('',#43062,#10045);
#7740=LINE('',#43066,#10046);
#7741=LINE('',#43070,#10047);
#7742=LINE('',#43073,#10048);
#7743=LINE('',#43076,#10049);
#7744=LINE('',#43079,#10050);
#7745=LINE('',#43082,#10051);
#7746=LINE('',#43085,#10052);
#7747=LINE('',#43088,#10053);
#7748=LINE('',#43091,#10054);
#7749=LINE('',#43093,#10055);
#7750=LINE('',#43095,#10056);
#7751=LINE('',#43097,#10057);
#7752=LINE('',#43099,#10058);
#7753=LINE('',#43116,#10059);
#9688=VECTOR('',#33419,10.);
#9689=VECTOR('',#33420,10.);
#9690=VECTOR('',#33421,10.);
#9691=VECTOR('',#33422,10.);
#9692=VECTOR('',#33423,10.);
#9693=VECTOR('',#33424,10.);
#9694=VECTOR('',#33427,10.);
#9695=VECTOR('',#33428,10.);
#9696=VECTOR('',#33429,10.);
#9697=VECTOR('',#33432,10.);
#9698=VECTOR('',#33433,10.);
#9699=VECTOR('',#33434,10.);
#9700=VECTOR('',#33435,10.);
#9701=VECTOR('',#33438,10.);
#9702=VECTOR('',#33439,10.);
#9703=VECTOR('',#33440,10.);
#9704=VECTOR('',#33443,10.);
#9705=VECTOR('',#33444,10.);
#9706=VECTOR('',#33445,10.);
#9707=VECTOR('',#33446,10.);
#9708=VECTOR('',#33449,10.);
#9709=VECTOR('',#33450,10.);
#9710=VECTOR('',#33451,10.);
#9711=VECTOR('',#33454,10.);
#9712=VECTOR('',#33455,10.);
#9713=VECTOR('',#33456,10.);
#9714=VECTOR('',#33457,10.);
#9715=VECTOR('',#33460,10.);
#9716=VECTOR('',#33461,10.);
#9717=VECTOR('',#33462,10.);
#9718=VECTOR('',#33463,10.);
#9719=VECTOR('',#33464,10.);
#9720=VECTOR('',#33465,10.);
#9721=VECTOR('',#33466,10.);
#9722=VECTOR('',#33467,10.);
#9723=VECTOR('',#33468,10.);
#9724=VECTOR('',#33469,10.);
#9725=VECTOR('',#33470,10.);
#9726=VECTOR('',#33471,10.);
#9727=VECTOR('',#33472,10.);
#9728=VECTOR('',#33473,10.);
#9729=VECTOR('',#33474,10.);
#9730=VECTOR('',#33475,10.);
#9731=VECTOR('',#33476,10.);
#9732=VECTOR('',#33477,10.);
#9733=VECTOR('',#33478,10.);
#9734=VECTOR('',#33479,10.);
#9735=VECTOR('',#33480,10.);
#9736=VECTOR('',#33481,10.);
#9737=VECTOR('',#33482,10.);
#9738=VECTOR('',#33483,10.);
#9739=VECTOR('',#33484,10.);
#9740=VECTOR('',#33485,10.);
#9741=VECTOR('',#33486,10.);
#9742=VECTOR('',#33487,10.);
#9743=VECTOR('',#33488,10.);
#9744=VECTOR('',#33489,10.);
#9745=VECTOR('',#33490,10.);
#9746=VECTOR('',#33491,10.);
#9747=VECTOR('',#33492,10.);
#9748=VECTOR('',#33493,10.);
#9749=VECTOR('',#33494,10.);
#9750=VECTOR('',#33495,10.);
#9751=VECTOR('',#33496,10.);
#9752=VECTOR('',#33497,10.);
#9753=VECTOR('',#33498,10.);
#9754=VECTOR('',#33499,10.);
#9755=VECTOR('',#33500,10.);
#9756=VECTOR('',#33501,10.);
#9757=VECTOR('',#33502,10.);
#9758=VECTOR('',#33503,10.);
#9759=VECTOR('',#33504,10.);
#9760=VECTOR('',#33505,10.);
#9761=VECTOR('',#33506,10.);
#9762=VECTOR('',#33507,10.);
#9763=VECTOR('',#33508,10.);
#9764=VECTOR('',#33509,10.);
#9765=VECTOR('',#33512,10.);
#9766=VECTOR('',#33513,10.);
#9767=VECTOR('',#33514,10.);
#9768=VECTOR('',#33515,10.);
#9769=VECTOR('',#33518,10.);
#9770=VECTOR('',#33519,10.);
#9771=VECTOR('',#33520,10.);
#9772=VECTOR('',#33525,1.8);
#9773=VECTOR('',#33530,10.);
#9774=VECTOR('',#33531,10.);
#9775=VECTOR('',#33532,10.);
#9776=VECTOR('',#33533,10.);
#9777=VECTOR('',#33538,1.55);
#9778=VECTOR('',#33543,1.8);
#9779=VECTOR('',#33548,1.55);
#9780=VECTOR('',#33555,4.75);
#9781=VECTOR('',#33560,4.5);
#9782=VECTOR('',#33571,4.75);
#9783=VECTOR('',#33576,4.5);
#9784=VECTOR('',#33587,4.75);
#9785=VECTOR('',#33592,4.5);
#9786=VECTOR('',#33603,4.75);
#9787=VECTOR('',#33608,4.5);
#9788=VECTOR('',#33617,10.);
#9789=VECTOR('',#33618,10.);
#9790=VECTOR('',#33621,10.);
#9791=VECTOR('',#33622,10.);
#9792=VECTOR('',#33623,10.);
#9793=VECTOR('',#33626,10.);
#9794=VECTOR('',#33627,10.);
#9795=VECTOR('',#33630,10.);
#9796=VECTOR('',#33631,10.);
#9797=VECTOR('',#33632,10.);
#9798=VECTOR('',#33635,10.);
#9799=VECTOR('',#33636,10.);
#9800=VECTOR('',#33637,10.);
#9801=VECTOR('',#33640,10.);
#9802=VECTOR('',#33641,10.);
#9803=VECTOR('',#33642,10.);
#9804=VECTOR('',#33645,10.);
#9805=VECTOR('',#33646,10.);
#9806=VECTOR('',#33649,10.);
#9807=VECTOR('',#33652,10.);
#9808=VECTOR('',#33655,10.);
#9809=VECTOR('',#33656,10.);
#9810=VECTOR('',#33659,10.);
#9811=VECTOR('',#33660,10.);
#9812=VECTOR('',#33663,10.);
#9813=VECTOR('',#33666,10.);
#9814=VECTOR('',#33667,10.);
#9815=VECTOR('',#33722,10.);
#9816=VECTOR('',#33723,10.);
#9817=VECTOR('',#33724,10.);
#9818=VECTOR('',#33727,10.);
#9819=VECTOR('',#33728,10.);
#9820=VECTOR('',#33731,10.);
#9821=VECTOR('',#33732,10.);
#9822=VECTOR('',#33735,10.);
#9823=VECTOR('',#33736,10.);
#9824=VECTOR('',#33739,10.);
#9825=VECTOR('',#33740,10.);
#9826=VECTOR('',#33743,10.);
#9827=VECTOR('',#33744,10.);
#9828=VECTOR('',#33747,10.);
#9829=VECTOR('',#33748,10.);
#9830=VECTOR('',#33751,10.);
#9831=VECTOR('',#33752,10.);
#9832=VECTOR('',#33755,10.);
#9833=VECTOR('',#33756,10.);
#9834=VECTOR('',#33759,10.);
#9835=VECTOR('',#33760,10.);
#9836=VECTOR('',#33763,10.);
#9837=VECTOR('',#33764,10.);
#9838=VECTOR('',#33767,10.);
#9839=VECTOR('',#33772,10.);
#9840=VECTOR('',#33773,10.);
#9841=VECTOR('',#33774,10.);
#9842=VECTOR('',#33775,10.);
#9843=VECTOR('',#33776,10.);
#9844=VECTOR('',#33777,10.);
#9845=VECTOR('',#33778,10.);
#9846=VECTOR('',#33781,10.);
#9847=VECTOR('',#33782,10.);
#9848=VECTOR('',#33785,10.);
#9849=VECTOR('',#33786,10.);
#9850=VECTOR('',#33789,10.);
#9851=VECTOR('',#33790,10.);
#9852=VECTOR('',#33791,10.);
#9853=VECTOR('',#33792,10.);
#9854=VECTOR('',#33793,10.);
#9855=VECTOR('',#33794,10.);
#9856=VECTOR('',#33795,10.);
#9857=VECTOR('',#33796,10.);
#9858=VECTOR('',#33797,10.);
#9859=VECTOR('',#33800,10.);
#9860=VECTOR('',#33801,10.);
#9861=VECTOR('',#33804,10.);
#9862=VECTOR('',#33805,10.);
#9863=VECTOR('',#33808,10.);
#9864=VECTOR('',#33809,10.);
#9865=VECTOR('',#33812,10.);
#9866=VECTOR('',#33817,10.);
#9867=VECTOR('',#33818,10.);
#9868=VECTOR('',#33819,10.);
#9869=VECTOR('',#33822,10.);
#9870=VECTOR('',#33823,10.);
#9871=VECTOR('',#33826,10.);
#9872=VECTOR('',#33827,10.);
#9873=VECTOR('',#33830,10.);
#9874=VECTOR('',#33831,10.);
#9875=VECTOR('',#33834,10.);
#9876=VECTOR('',#33835,10.);
#9877=VECTOR('',#33838,10.);
#9878=VECTOR('',#33839,10.);
#9879=VECTOR('',#33842,10.);
#9880=VECTOR('',#33843,10.);
#9881=VECTOR('',#33846,10.);
#9882=VECTOR('',#33847,10.);
#9883=VECTOR('',#33850,10.);
#9884=VECTOR('',#33851,10.);
#9885=VECTOR('',#33854,10.);
#9886=VECTOR('',#33855,10.);
#9887=VECTOR('',#33858,10.);
#9888=VECTOR('',#33859,10.);
#9889=VECTOR('',#33862,10.);
#9890=VECTOR('',#33865,10.);
#9891=VECTOR('',#33866,10.);
#9892=VECTOR('',#33867,10.);
#9893=VECTOR('',#33870,10.);
#9894=VECTOR('',#33871,10.);
#9895=VECTOR('',#33872,10.);
#9896=VECTOR('',#33873,10.);
#9897=VECTOR('',#33874,10.);
#9898=VECTOR('',#33877,10.);
#9899=VECTOR('',#33878,10.);
#9900=VECTOR('',#33881,10.);
#9901=VECTOR('',#33882,10.);
#9902=VECTOR('',#33885,10.);
#9903=VECTOR('',#33886,10.);
#9904=VECTOR('',#33889,10.);
#9905=VECTOR('',#33890,10.);
#9906=VECTOR('',#33893,10.);
#9907=VECTOR('',#33894,10.);
#9908=VECTOR('',#33895,10.);
#9909=VECTOR('',#33896,10.);
#9910=VECTOR('',#33897,10.);
#9911=VECTOR('',#33898,10.);
#9912=VECTOR('',#33899,10.);
#9913=VECTOR('',#33900,10.);
#9914=VECTOR('',#33901,10.);
#9915=VECTOR('',#33902,10.);
#9916=VECTOR('',#33903,10.);
#9917=VECTOR('',#33904,10.);
#9918=VECTOR('',#33905,10.);
#9919=VECTOR('',#33906,10.);
#9920=VECTOR('',#33909,10.);
#9921=VECTOR('',#33910,10.);
#9922=VECTOR('',#33911,10.);
#9923=VECTOR('',#33912,10.);
#9924=VECTOR('',#33913,10.);
#9925=VECTOR('',#33914,10.);
#9926=VECTOR('',#33915,10.);
#9927=VECTOR('',#33916,10.);
#9928=VECTOR('',#33917,10.);
#9929=VECTOR('',#33918,10.);
#9930=VECTOR('',#33919,10.);
#9931=VECTOR('',#33920,10.);
#9932=VECTOR('',#33921,10.);
#9933=VECTOR('',#33922,10.);
#9934=VECTOR('',#33923,10.);
#9935=VECTOR('',#33924,10.);
#9936=VECTOR('',#33925,10.);
#9937=VECTOR('',#33926,10.);
#9938=VECTOR('',#33927,10.);
#9939=VECTOR('',#33928,10.);
#9940=VECTOR('',#33931,10.);
#9941=VECTOR('',#33932,10.);
#9942=VECTOR('',#33933,10.);
#9943=VECTOR('',#33936,10.);
#9944=VECTOR('',#33937,10.);
#9945=VECTOR('',#33938,10.);
#9946=VECTOR('',#33939,10.);
#9947=VECTOR('',#33940,10.);
#9948=VECTOR('',#33941,10.);
#9949=VECTOR('',#33942,10.);
#9950=VECTOR('',#33943,10.);
#9951=VECTOR('',#33944,10.);
#9952=VECTOR('',#33945,10.);
#9953=VECTOR('',#33946,10.);
#9954=VECTOR('',#33947,10.);
#9955=VECTOR('',#33950,10.);
#9956=VECTOR('',#33951,10.);
#9957=VECTOR('',#33952,10.);
#9958=VECTOR('',#33953,10.);
#9959=VECTOR('',#33954,10.);
#9960=VECTOR('',#33955,10.);
#9961=VECTOR('',#33956,10.);
#9962=VECTOR('',#33957,10.);
#9963=VECTOR('',#33958,10.);
#9964=VECTOR('',#33961,10.);
#9965=VECTOR('',#33962,10.);
#9966=VECTOR('',#33963,10.);
#9967=VECTOR('',#33964,10.);
#9968=VECTOR('',#33965,10.);
#9969=VECTOR('',#33966,10.);
#9970=VECTOR('',#33967,10.);
#9971=VECTOR('',#33968,10.);
#9972=VECTOR('',#33969,10.);
#9973=VECTOR('',#33972,10.);
#9974=VECTOR('',#33973,10.);
#9975=VECTOR('',#33974,10.);
#9976=VECTOR('',#33979,10.);
#9977=VECTOR('',#33980,10.);
#9978=VECTOR('',#33981,10.);
#9979=VECTOR('',#33984,10.);
#9980=VECTOR('',#33985,10.);
#9981=VECTOR('',#33988,10.);
#9982=VECTOR('',#33989,10.);
#9983=VECTOR('',#33992,10.);
#9984=VECTOR('',#33995,10.);
#9985=VECTOR('',#33996,10.);
#9986=VECTOR('',#33997,10.);
#9987=VECTOR('',#33998,10.);
#9988=VECTOR('',#33999,10.);
#9989=VECTOR('',#34000,10.);
#9990=VECTOR('',#34001,10.);
#9991=VECTOR('',#34002,10.);
#9992=VECTOR('',#34003,10.);
#9993=VECTOR('',#34004,10.);
#9994=VECTOR('',#34005,10.);
#9995=VECTOR('',#34006,10.);
#9996=VECTOR('',#34007,10.);
#9997=VECTOR('',#34008,10.);
#9998=VECTOR('',#34011,10.);
#9999=VECTOR('',#34012,10.);
#10000=VECTOR('',#34013,10.);
#10001=VECTOR('',#34014,10.);
#10002=VECTOR('',#34015,10.);
#10003=VECTOR('',#34016,10.);
#10004=VECTOR('',#34017,10.);
#10005=VECTOR('',#34018,10.);
#10006=VECTOR('',#34019,10.);
#10007=VECTOR('',#34020,10.);
#10008=VECTOR('',#34021,10.);
#10009=VECTOR('',#34022,10.);
#10010=VECTOR('',#34023,10.);
#10011=VECTOR('',#34024,10.);
#10012=VECTOR('',#34025,10.);
#10013=VECTOR('',#34026,10.);
#10014=VECTOR('',#34027,10.);
#10015=VECTOR('',#34028,10.);
#10016=VECTOR('',#34029,10.);
#10017=VECTOR('',#34030,10.);
#10018=VECTOR('',#34033,10.);
#10019=VECTOR('',#34034,10.);
#10020=VECTOR('',#34035,10.);
#10021=VECTOR('',#34040,4.25);
#10022=VECTOR('',#34047,4.05);
#10023=VECTOR('',#34050,3.25);
#10024=VECTOR('',#34055,3.05);
#10025=VECTOR('',#34060,3.25);
#10026=VECTOR('',#34065,3.05);
#10027=VECTOR('',#34070,3.25);
#10028=VECTOR('',#34075,3.05);
#10029=VECTOR('',#34080,3.25);
#10030=VECTOR('',#34085,3.05000000000001);
#10031=VECTOR('',#34090,3.25);
#10032=VECTOR('',#34095,3.05);
#10033=VECTOR('',#34100,3.25);
#10034=VECTOR('',#34105,3.05000000000001);
#10035=VECTOR('',#34110,3.25);
#10036=VECTOR('',#34115,3.05);
#10037=VECTOR('',#34120,3.25);
#10038=VECTOR('',#34125,3.05);
#10039=VECTOR('',#34130,3.25);
#10040=VECTOR('',#34135,3.05000000000001);
#10041=VECTOR('',#34140,3.25);
#10042=VECTOR('',#34145,3.05);
#10043=VECTOR('',#34150,3.25);
#10044=VECTOR('',#34155,3.05000000000001);
#10045=VECTOR('',#34160,3.25);
#10046=VECTOR('',#34165,3.05);
#10047=VECTOR('',#34170,7.2);
#10048=VECTOR('',#34175,7.);
#10049=VECTOR('',#34178,7.2);
#10050=VECTOR('',#34183,7.);
#10051=VECTOR('',#34186,7.2);
#10052=VECTOR('',#34191,7.);
#10053=VECTOR('',#34194,7.2);
#10054=VECTOR('',#34199,7.);
#10055=VECTOR('',#34202,4.7);
#10056=VECTOR('',#34205,4.7);
#10057=VECTOR('',#34208,4.7);
#10058=VECTOR('',#34211,4.7);
#10059=VECTOR('',#34242,5.5);
#11994=VERTEX_POINT('',#40768);
#11995=VERTEX_POINT('',#40769);
#11996=VERTEX_POINT('',#40771);
#11997=VERTEX_POINT('',#40773);
#11998=VERTEX_POINT('',#40775);
#11999=VERTEX_POINT('',#40777);
#12000=VERTEX_POINT('',#40781);
#12001=VERTEX_POINT('',#40783);
#12002=VERTEX_POINT('',#40787);
#12003=VERTEX_POINT('',#40789);
#12004=VERTEX_POINT('',#40791);
#12005=VERTEX_POINT('',#40795);
#12006=VERTEX_POINT('',#40797);
#12007=VERTEX_POINT('',#40801);
#12008=VERTEX_POINT('',#40803);
#12009=VERTEX_POINT('',#40805);
#12010=VERTEX_POINT('',#40809);
#12011=VERTEX_POINT('',#40811);
#12012=VERTEX_POINT('',#40815);
#12013=VERTEX_POINT('',#40817);
#12014=VERTEX_POINT('',#40819);
#12015=VERTEX_POINT('',#40823);
#12016=VERTEX_POINT('',#40826);
#12017=VERTEX_POINT('',#40827);
#12018=VERTEX_POINT('',#40829);
#12019=VERTEX_POINT('',#40831);
#12020=VERTEX_POINT('',#40833);
#12021=VERTEX_POINT('',#40835);
#12022=VERTEX_POINT('',#40837);
#12023=VERTEX_POINT('',#40839);
#12024=VERTEX_POINT('',#40841);
#12025=VERTEX_POINT('',#40843);
#12026=VERTEX_POINT('',#40845);
#12027=VERTEX_POINT('',#40847);
#12028=VERTEX_POINT('',#40850);
#12029=VERTEX_POINT('',#40851);
#12030=VERTEX_POINT('',#40853);
#12031=VERTEX_POINT('',#40855);
#12032=VERTEX_POINT('',#40857);
#12033=VERTEX_POINT('',#40859);
#12034=VERTEX_POINT('',#40861);
#12035=VERTEX_POINT('',#40865);
#12036=VERTEX_POINT('',#40869);
#12037=VERTEX_POINT('',#40873);
#12038=VERTEX_POINT('',#40877);
#12039=VERTEX_POINT('',#40881);
#12040=VERTEX_POINT('',#40885);
#12041=VERTEX_POINT('',#40889);
#12042=VERTEX_POINT('',#40891);
#12043=VERTEX_POINT('',#40893);
#12044=VERTEX_POINT('',#40895);
#12045=VERTEX_POINT('',#40899);
#12046=VERTEX_POINT('',#40903);
#12047=VERTEX_POINT('',#40910);
#12048=VERTEX_POINT('',#40911);
#12049=VERTEX_POINT('',#40913);
#12050=VERTEX_POINT('',#40915);
#12051=VERTEX_POINT('',#40917);
#12052=VERTEX_POINT('',#40919);
#12053=VERTEX_POINT('',#40921);
#12054=VERTEX_POINT('',#40923);
#12055=VERTEX_POINT('',#40925);
#12056=VERTEX_POINT('',#40927);
#12057=VERTEX_POINT('',#40929);
#12058=VERTEX_POINT('',#40931);
#12059=VERTEX_POINT('',#40934);
#12060=VERTEX_POINT('',#40935);
#12061=VERTEX_POINT('',#40939);
#12062=VERTEX_POINT('',#40943);
#12063=VERTEX_POINT('',#40945);
#12064=VERTEX_POINT('',#40947);
#12065=VERTEX_POINT('',#40949);
#12066=VERTEX_POINT('',#40951);
#12067=VERTEX_POINT('',#40955);
#12068=VERTEX_POINT('',#40959);
#12069=VERTEX_POINT('',#40963);
#12070=VERTEX_POINT('',#40968);
#12071=VERTEX_POINT('',#40969);
#12072=VERTEX_POINT('',#40973);
#12073=VERTEX_POINT('',#40977);
#12074=VERTEX_POINT('',#40981);
#12075=VERTEX_POINT('',#40983);
#12076=VERTEX_POINT('',#40987);
#12077=VERTEX_POINT('',#40991);
#12078=VERTEX_POINT('',#40995);
#12079=VERTEX_POINT('',#40999);
#12080=VERTEX_POINT('',#41003);
#12081=VERTEX_POINT('',#41007);
#12082=VERTEX_POINT('',#41011);
#12083=VERTEX_POINT('',#41015);
#12084=VERTEX_POINT('',#41019);
#12085=VERTEX_POINT('',#41023);
#12086=VERTEX_POINT('',#41027);
#12087=VERTEX_POINT('',#41031);
#12088=VERTEX_POINT('',#41035);
#12089=VERTEX_POINT('',#41039);
#12090=VERTEX_POINT('',#41043);
#12091=VERTEX_POINT('',#41047);
#12092=VERTEX_POINT('',#41051);
#12093=VERTEX_POINT('',#41055);
#12094=VERTEX_POINT('',#41057);
#12095=VERTEX_POINT('',#41061);
#12096=VERTEX_POINT('',#41065);
#12097=VERTEX_POINT('',#41069);
#12098=VERTEX_POINT('',#41073);
#12099=VERTEX_POINT('',#41077);
#12100=VERTEX_POINT('',#41081);
#12101=VERTEX_POINT('',#41085);
#12102=VERTEX_POINT('',#41089);
#12103=VERTEX_POINT('',#41093);
#12104=VERTEX_POINT('',#41097);
#12105=VERTEX_POINT('',#41104);
#12106=VERTEX_POINT('',#41105);
#12107=VERTEX_POINT('',#41109);
#12108=VERTEX_POINT('',#41113);
#12109=VERTEX_POINT('',#41117);
#12110=VERTEX_POINT('',#41119);
#12111=VERTEX_POINT('',#41123);
#12112=VERTEX_POINT('',#41127);
#12113=VERTEX_POINT('',#41131);
#12114=VERTEX_POINT('',#41135);
#12115=VERTEX_POINT('',#41139);
#12116=VERTEX_POINT('',#41143);
#12117=VERTEX_POINT('',#41147);
#12118=VERTEX_POINT('',#41149);
#12119=VERTEX_POINT('',#41153);
#12120=VERTEX_POINT('',#41157);
#12121=VERTEX_POINT('',#41161);
#12122=VERTEX_POINT('',#41165);
#12123=VERTEX_POINT('',#41169);
#12124=VERTEX_POINT('',#41173);
#12125=VERTEX_POINT('',#41177);
#12126=VERTEX_POINT('',#41179);
#12127=VERTEX_POINT('',#41183);
#12128=VERTEX_POINT('',#41187);
#12129=VERTEX_POINT('',#41191);
#12130=VERTEX_POINT('',#41195);
#12131=VERTEX_POINT('',#41199);
#12132=VERTEX_POINT('',#41203);
#12133=VERTEX_POINT('',#41207);
#12134=VERTEX_POINT('',#41211);
#12135=VERTEX_POINT('',#41218);
#12136=VERTEX_POINT('',#41219);
#12137=VERTEX_POINT('',#41221);
#12138=VERTEX_POINT('',#41223);
#12139=VERTEX_POINT('',#41226);
#12140=VERTEX_POINT('',#41227);
#12141=VERTEX_POINT('',#41231);
#12142=VERTEX_POINT('',#41235);
#12143=VERTEX_POINT('',#41239);
#12144=VERTEX_POINT('',#41241);
#12145=VERTEX_POINT('',#41245);
#12146=VERTEX_POINT('',#41249);
#12147=VERTEX_POINT('',#41253);
#12148=VERTEX_POINT('',#41257);
#12149=VERTEX_POINT('',#41261);
#12150=VERTEX_POINT('',#41265);
#12151=VERTEX_POINT('',#41269);
#12152=VERTEX_POINT('',#41273);
#12153=VERTEX_POINT('',#41277);
#12154=VERTEX_POINT('',#41281);
#12155=VERTEX_POINT('',#41285);
#12156=VERTEX_POINT('',#41289);
#12157=VERTEX_POINT('',#41293);
#12158=VERTEX_POINT('',#41297);
#12159=VERTEX_POINT('',#41301);
#12160=VERTEX_POINT('',#41305);
#12161=VERTEX_POINT('',#41309);
#12162=VERTEX_POINT('',#41313);
#12163=VERTEX_POINT('',#41315);
#12164=VERTEX_POINT('',#41319);
#12165=VERTEX_POINT('',#41323);
#12166=VERTEX_POINT('',#41327);
#12167=VERTEX_POINT('',#41331);
#12168=VERTEX_POINT('',#41335);
#12169=VERTEX_POINT('',#41339);
#12170=VERTEX_POINT('',#41343);
#12171=VERTEX_POINT('',#41347);
#12172=VERTEX_POINT('',#41351);
#12173=VERTEX_POINT('',#41355);
#12174=VERTEX_POINT('',#41363);
#12175=VERTEX_POINT('',#41364);
#12176=VERTEX_POINT('',#41366);
#12177=VERTEX_POINT('',#41371);
#12178=VERTEX_POINT('',#41373);
#12179=VERTEX_POINT('',#41377);
#12180=VERTEX_POINT('',#41379);
#12181=VERTEX_POINT('',#41383);
#12182=VERTEX_POINT('',#41384);
#12183=VERTEX_POINT('',#41386);
#12184=VERTEX_POINT('',#41390);
#12185=VERTEX_POINT('',#41393);
#12186=VERTEX_POINT('',#41397);
#12187=VERTEX_POINT('',#41401);
#12188=VERTEX_POINT('',#41405);
#12189=VERTEX_POINT('',#41407);
#12190=VERTEX_POINT('',#41411);
#12191=VERTEX_POINT('',#41415);
#12192=VERTEX_POINT('',#41418);
#12193=VERTEX_POINT('',#41420);
#12194=VERTEX_POINT('',#41424);
#12195=VERTEX_POINT('',#41428);
#12196=VERTEX_POINT('',#41431);
#12197=VERTEX_POINT('',#41433);
#12198=VERTEX_POINT('',#41437);
#12199=VERTEX_POINT('',#41441);
#12200=VERTEX_POINT('',#41444);
#12201=VERTEX_POINT('',#41446);
#12202=VERTEX_POINT('',#41450);
#12203=VERTEX_POINT('',#41454);
#12204=VERTEX_POINT('',#41457);
#12205=VERTEX_POINT('',#41461);
#12206=VERTEX_POINT('',#41466);
#12207=VERTEX_POINT('',#41470);
#12208=VERTEX_POINT('',#41471);
#12209=VERTEX_POINT('',#41476);
#12210=VERTEX_POINT('',#41477);
#12211=VERTEX_POINT('',#41479);
#12212=VERTEX_POINT('',#41483);
#12213=VERTEX_POINT('',#41485);
#12214=VERTEX_POINT('',#41508);
#12215=VERTEX_POINT('',#41510);
#12216=VERTEX_POINT('',#41512);
#12217=VERTEX_POINT('',#41514);
#12218=VERTEX_POINT('',#41516);
#12219=VERTEX_POINT('',#41518);
#12220=VERTEX_POINT('',#41520);
#12221=VERTEX_POINT('',#41522);
#12222=VERTEX_POINT('',#41524);
#12223=VERTEX_POINT('',#41526);
#12224=VERTEX_POINT('',#41528);
#12225=VERTEX_POINT('',#41530);
#12226=VERTEX_POINT('',#41532);
#12227=VERTEX_POINT('',#41534);
#12228=VERTEX_POINT('',#41536);
#12229=VERTEX_POINT('',#41538);
#12230=VERTEX_POINT('',#41540);
#12231=VERTEX_POINT('',#41544);
#12232=VERTEX_POINT('',#41546);
#12233=VERTEX_POINT('',#41548);
#12234=VERTEX_POINT('',#41550);
#12235=VERTEX_POINT('',#41552);
#12236=VERTEX_POINT('',#41555);
#12237=VERTEX_POINT('',#41557);
#12238=VERTEX_POINT('',#41561);
#12239=VERTEX_POINT('',#41565);
#12240=VERTEX_POINT('',#41569);
#12241=VERTEX_POINT('',#41573);
#12242=VERTEX_POINT('',#41577);
#12243=VERTEX_POINT('',#41581);
#12244=VERTEX_POINT('',#41585);
#12245=VERTEX_POINT('',#41589);
#12246=VERTEX_POINT('',#41593);
#12247=VERTEX_POINT('',#41597);
#12248=VERTEX_POINT('',#41604);
#12249=VERTEX_POINT('',#41606);
#12250=VERTEX_POINT('',#41615);
#12251=VERTEX_POINT('',#41626);
#12252=VERTEX_POINT('',#41637);
#12253=VERTEX_POINT('',#41648);
#12254=VERTEX_POINT('',#41654);
#12255=VERTEX_POINT('',#41658);
#12256=VERTEX_POINT('',#41662);
#12257=VERTEX_POINT('',#41671);
#12258=VERTEX_POINT('',#41682);
#12259=VERTEX_POINT('',#41693);
#12260=VERTEX_POINT('',#41704);
#12261=VERTEX_POINT('',#41715);
#12262=VERTEX_POINT('',#41726);
#12263=VERTEX_POINT('',#41737);
#12264=VERTEX_POINT('',#41743);
#12265=VERTEX_POINT('',#41747);
#12266=VERTEX_POINT('',#41751);
#12267=VERTEX_POINT('',#41758);
#12268=VERTEX_POINT('',#41760);
#12269=VERTEX_POINT('',#41764);
#12270=VERTEX_POINT('',#41768);
#12271=VERTEX_POINT('',#41772);
#12272=VERTEX_POINT('',#41776);
#12273=VERTEX_POINT('',#41780);
#12274=VERTEX_POINT('',#41784);
#12275=VERTEX_POINT('',#41788);
#12276=VERTEX_POINT('',#41792);
#12277=VERTEX_POINT('',#41796);
#12278=VERTEX_POINT('',#41800);
#12279=VERTEX_POINT('',#41812);
#12280=VERTEX_POINT('',#41814);
#12281=VERTEX_POINT('',#41825);
#12282=VERTEX_POINT('',#41831);
#12283=VERTEX_POINT('',#41840);
#12284=VERTEX_POINT('',#41851);
#12285=VERTEX_POINT('',#41862);
#12286=VERTEX_POINT('',#41868);
#12287=VERTEX_POINT('',#41872);
#12288=VERTEX_POINT('',#41876);
#12289=VERTEX_POINT('',#41880);
#12290=VERTEX_POINT('',#41899);
#12291=VERTEX_POINT('',#41901);
#12292=VERTEX_POINT('',#41912);
#12293=VERTEX_POINT('',#41923);
#12294=VERTEX_POINT('',#41934);
#12295=VERTEX_POINT('',#41945);
#12296=VERTEX_POINT('',#41956);
#12297=VERTEX_POINT('',#41967);
#12298=VERTEX_POINT('',#41978);
#12299=VERTEX_POINT('',#41989);
#12300=VERTEX_POINT('',#42000);
#12301=VERTEX_POINT('',#42011);
#12302=VERTEX_POINT('',#42022);
#12303=VERTEX_POINT('',#42033);
#12304=VERTEX_POINT('',#42039);
#12305=VERTEX_POINT('',#42048);
#12306=VERTEX_POINT('',#42059);
#12307=VERTEX_POINT('',#42070);
#12308=VERTEX_POINT('',#42081);
#12309=VERTEX_POINT('',#42092);
#12310=VERTEX_POINT('',#42103);
#12311=VERTEX_POINT('',#42114);
#12312=VERTEX_POINT('',#42125);
#12313=VERTEX_POINT('',#42136);
#12314=VERTEX_POINT('',#42147);
#12315=VERTEX_POINT('',#42158);
#12316=VERTEX_POINT('',#42169);
#12317=VERTEX_POINT('',#42180);
#12318=VERTEX_POINT('',#42191);
#12319=VERTEX_POINT('',#42202);
#12320=VERTEX_POINT('',#42213);
#12321=VERTEX_POINT('',#42224);
#12322=VERTEX_POINT('',#42235);
#12323=VERTEX_POINT('',#42241);
#12324=VERTEX_POINT('',#42250);
#12325=VERTEX_POINT('',#42271);
#12326=VERTEX_POINT('',#42273);
#12327=VERTEX_POINT('',#42284);
#12328=VERTEX_POINT('',#42295);
#12329=VERTEX_POINT('',#42306);
#12330=VERTEX_POINT('',#42317);
#12331=VERTEX_POINT('',#42328);
#12332=VERTEX_POINT('',#42339);
#12333=VERTEX_POINT('',#42350);
#12334=VERTEX_POINT('',#42361);
#12335=VERTEX_POINT('',#42372);
#12336=VERTEX_POINT('',#42383);
#12337=VERTEX_POINT('',#42389);
#12338=VERTEX_POINT('',#42398);
#12339=VERTEX_POINT('',#42409);
#12340=VERTEX_POINT('',#42420);
#12341=VERTEX_POINT('',#42431);
#12342=VERTEX_POINT('',#42442);
#12343=VERTEX_POINT('',#42453);
#12344=VERTEX_POINT('',#42464);
#12345=VERTEX_POINT('',#42470);
#12346=VERTEX_POINT('',#42479);
#12347=VERTEX_POINT('',#42490);
#12348=VERTEX_POINT('',#42501);
#12349=VERTEX_POINT('',#42512);
#12350=VERTEX_POINT('',#42523);
#12351=VERTEX_POINT('',#42534);
#12352=VERTEX_POINT('',#42545);
#12353=VERTEX_POINT('',#42551);
#12354=VERTEX_POINT('',#42560);
#12355=VERTEX_POINT('',#42576);
#12356=VERTEX_POINT('',#42578);
#12357=VERTEX_POINT('',#42582);
#12358=VERTEX_POINT('',#42586);
#12359=VERTEX_POINT('',#42598);
#12360=VERTEX_POINT('',#42600);
#12361=VERTEX_POINT('',#42611);
#12362=VERTEX_POINT('',#42622);
#12363=VERTEX_POINT('',#42633);
#12364=VERTEX_POINT('',#42644);
#12365=VERTEX_POINT('',#42655);
#12366=VERTEX_POINT('',#42666);
#12367=VERTEX_POINT('',#42677);
#12368=VERTEX_POINT('',#42688);
#12369=VERTEX_POINT('',#42699);
#12370=VERTEX_POINT('',#42710);
#12371=VERTEX_POINT('',#42721);
#12372=VERTEX_POINT('',#42732);
#12373=VERTEX_POINT('',#42738);
#12374=VERTEX_POINT('',#42747);
#12375=VERTEX_POINT('',#42758);
#12376=VERTEX_POINT('',#42769);
#12377=VERTEX_POINT('',#42780);
#12378=VERTEX_POINT('',#42791);
#12379=VERTEX_POINT('',#42802);
#12380=VERTEX_POINT('',#42813);
#12381=VERTEX_POINT('',#42824);
#12382=VERTEX_POINT('',#42835);
#12383=VERTEX_POINT('',#42846);
#12384=VERTEX_POINT('',#42857);
#12385=VERTEX_POINT('',#42868);
#12386=VERTEX_POINT('',#42879);
#12387=VERTEX_POINT('',#42890);
#12388=VERTEX_POINT('',#42901);
#12389=VERTEX_POINT('',#42912);
#12390=VERTEX_POINT('',#42923);
#12391=VERTEX_POINT('',#42934);
#12392=VERTEX_POINT('',#42940);
#12393=VERTEX_POINT('',#42949);
#12394=VERTEX_POINT('',#42965);
#12395=VERTEX_POINT('',#42969);
#12396=VERTEX_POINT('',#42973);
#12397=VERTEX_POINT('',#42977);
#12398=VERTEX_POINT('',#42981);
#12399=VERTEX_POINT('',#42985);
#12400=VERTEX_POINT('',#42989);
#12401=VERTEX_POINT('',#42993);
#12402=VERTEX_POINT('',#42997);
#12403=VERTEX_POINT('',#43001);
#12404=VERTEX_POINT('',#43005);
#12405=VERTEX_POINT('',#43009);
#12406=VERTEX_POINT('',#43013);
#12407=VERTEX_POINT('',#43017);
#12408=VERTEX_POINT('',#43021);
#12409=VERTEX_POINT('',#43025);
#12410=VERTEX_POINT('',#43029);
#12411=VERTEX_POINT('',#43033);
#12412=VERTEX_POINT('',#43037);
#12413=VERTEX_POINT('',#43041);
#12414=VERTEX_POINT('',#43045);
#12415=VERTEX_POINT('',#43049);
#12416=VERTEX_POINT('',#43053);
#12417=VERTEX_POINT('',#43057);
#12418=VERTEX_POINT('',#43061);
#12419=VERTEX_POINT('',#43065);
#12420=VERTEX_POINT('',#43069);
#12421=VERTEX_POINT('',#43075);
#12422=VERTEX_POINT('',#43081);
#12423=VERTEX_POINT('',#43087);
#12424=VERTEX_POINT('',#43115);
#14856=EDGE_CURVE('',#11994,#11995,#7382,.T.);
#14857=EDGE_CURVE('',#11995,#11996,#7383,.T.);
#14858=EDGE_CURVE('',#11996,#11997,#7384,.T.);
#14859=EDGE_CURVE('',#11997,#11998,#7385,.T.);
#14860=EDGE_CURVE('',#11998,#11999,#7386,.T.);
#14861=EDGE_CURVE('',#11999,#11994,#7387,.T.);
#14862=EDGE_CURVE('',#12000,#11995,#7388,.T.);
#14863=EDGE_CURVE('',#12001,#12000,#7389,.T.);
#14864=EDGE_CURVE('',#11996,#12001,#7390,.T.);
#14865=EDGE_CURVE('',#12002,#11994,#7391,.T.);
#14866=EDGE_CURVE('',#12002,#12003,#7392,.T.);
#14867=EDGE_CURVE('',#12003,#12004,#7393,.T.);
#14868=EDGE_CURVE('',#12000,#12004,#7394,.T.);
#14869=EDGE_CURVE('',#11999,#12005,#7395,.T.);
#14870=EDGE_CURVE('',#12005,#12006,#7396,.T.);
#14871=EDGE_CURVE('',#12006,#12002,#7397,.T.);
#14872=EDGE_CURVE('',#12004,#12007,#7398,.T.);
#14873=EDGE_CURVE('',#12007,#12008,#7399,.T.);
#14874=EDGE_CURVE('',#12008,#12009,#7400,.T.);
#14875=EDGE_CURVE('',#12009,#12001,#7401,.T.);
#14876=EDGE_CURVE('',#12010,#12009,#7402,.T.);
#14877=EDGE_CURVE('',#12010,#12011,#7403,.T.);
#14878=EDGE_CURVE('',#12011,#11997,#7404,.T.);
#14879=EDGE_CURVE('',#12008,#12012,#7405,.T.);
#14880=EDGE_CURVE('',#12013,#12012,#7406,.T.);
#14881=EDGE_CURVE('',#12014,#12013,#7407,.T.);
#14882=EDGE_CURVE('',#12014,#12010,#7408,.T.);
#14883=EDGE_CURVE('',#12015,#12007,#7409,.T.);
#14884=EDGE_CURVE('',#12012,#12015,#7410,.T.);
#14885=EDGE_CURVE('',#12016,#12017,#7411,.T.);
#14886=EDGE_CURVE('',#12017,#12018,#7412,.T.);
#14887=EDGE_CURVE('',#12018,#12019,#7413,.T.);
#14888=EDGE_CURVE('',#12019,#12020,#7414,.T.);
#14889=EDGE_CURVE('',#12020,#12021,#7415,.T.);
#14890=EDGE_CURVE('',#12021,#12022,#7416,.T.);
#14891=EDGE_CURVE('',#12022,#12023,#7417,.T.);
#14892=EDGE_CURVE('',#12023,#12024,#7418,.T.);
#14893=EDGE_CURVE('',#12024,#12025,#7419,.T.);
#14894=EDGE_CURVE('',#12025,#12026,#7420,.T.);
#14895=EDGE_CURVE('',#12026,#12027,#7421,.T.);
#14896=EDGE_CURVE('',#12027,#12016,#7422,.T.);
#14897=EDGE_CURVE('',#12028,#12029,#7423,.T.);
#14898=EDGE_CURVE('',#12029,#12030,#7424,.T.);
#14899=EDGE_CURVE('',#12030,#12031,#7425,.T.);
#14900=EDGE_CURVE('',#12031,#12032,#7426,.T.);
#14901=EDGE_CURVE('',#12032,#12033,#7427,.T.);
#14902=EDGE_CURVE('',#12033,#12034,#2083,.T.);
#14903=EDGE_CURVE('',#12034,#12035,#2084,.T.);
#14904=EDGE_CURVE('',#12035,#12036,#2085,.T.);
#14905=EDGE_CURVE('',#12036,#12037,#2086,.T.);
#14906=EDGE_CURVE('',#12037,#12038,#2087,.T.);
#14907=EDGE_CURVE('',#12038,#12039,#2088,.T.);
#14908=EDGE_CURVE('',#12039,#12040,#2089,.T.);
#14909=EDGE_CURVE('',#12040,#12041,#7428,.T.);
#14910=EDGE_CURVE('',#12041,#12042,#7429,.T.);
#14911=EDGE_CURVE('',#12042,#12043,#7430,.T.);
#14912=EDGE_CURVE('',#12043,#12044,#2090,.T.);
#14913=EDGE_CURVE('',#12044,#12045,#2091,.T.);
#14914=EDGE_CURVE('',#12045,#12046,#2092,.T.);
#14915=EDGE_CURVE('',#12046,#12028,#2093,.T.);
#14916=EDGE_CURVE('',#12047,#12048,#7431,.T.);
#14917=EDGE_CURVE('',#12048,#12049,#7432,.T.);
#14918=EDGE_CURVE('',#12049,#12050,#7433,.T.);
#14919=EDGE_CURVE('',#12050,#12051,#7434,.T.);
#14920=EDGE_CURVE('',#12051,#12052,#7435,.T.);
#14921=EDGE_CURVE('',#12052,#12053,#7436,.T.);
#14922=EDGE_CURVE('',#12053,#12054,#7437,.T.);
#14923=EDGE_CURVE('',#12054,#12055,#7438,.T.);
#14924=EDGE_CURVE('',#12055,#12056,#7439,.T.);
#14925=EDGE_CURVE('',#12056,#12057,#7440,.T.);
#14926=EDGE_CURVE('',#12057,#12058,#7441,.T.);
#14927=EDGE_CURVE('',#12058,#12047,#7442,.T.);
#14928=EDGE_CURVE('',#12059,#12060,#2094,.T.);
#14929=EDGE_CURVE('',#12060,#12061,#2095,.T.);
#14930=EDGE_CURVE('',#12061,#12062,#7443,.T.);
#14931=EDGE_CURVE('',#12062,#12063,#7444,.T.);
#14932=EDGE_CURVE('',#12063,#12064,#7445,.T.);
#14933=EDGE_CURVE('',#12064,#12065,#7446,.T.);
#14934=EDGE_CURVE('',#12065,#12066,#2096,.T.);
#14935=EDGE_CURVE('',#12066,#12067,#2097,.T.);
#14936=EDGE_CURVE('',#12067,#12068,#2098,.T.);
#14937=EDGE_CURVE('',#12068,#12069,#7447,.T.);
#14938=EDGE_CURVE('',#12069,#12059,#2099,.T.);
#14939=EDGE_CURVE('',#12070,#12071,#2100,.T.);
#14940=EDGE_CURVE('',#12071,#12072,#2101,.T.);
#14941=EDGE_CURVE('',#12072,#12073,#2102,.T.);
#14942=EDGE_CURVE('',#12073,#12074,#7448,.T.);
#14943=EDGE_CURVE('',#12074,#12075,#2103,.T.);
#14944=EDGE_CURVE('',#12075,#12076,#2104,.T.);
#14945=EDGE_CURVE('',#12076,#12077,#2105,.T.);
#14946=EDGE_CURVE('',#12077,#12078,#2106,.T.);
#14947=EDGE_CURVE('',#12078,#12079,#2107,.T.);
#14948=EDGE_CURVE('',#12079,#12080,#2108,.T.);
#14949=EDGE_CURVE('',#12080,#12081,#2109,.T.);
#14950=EDGE_CURVE('',#12081,#12082,#2110,.T.);
#14951=EDGE_CURVE('',#12082,#12083,#2111,.T.);
#14952=EDGE_CURVE('',#12083,#12084,#2112,.T.);
#14953=EDGE_CURVE('',#12084,#12085,#2113,.T.);
#14954=EDGE_CURVE('',#12085,#12086,#2114,.T.);
#14955=EDGE_CURVE('',#12086,#12087,#2115,.T.);
#14956=EDGE_CURVE('',#12087,#12088,#2116,.T.);
#14957=EDGE_CURVE('',#12088,#12089,#2117,.T.);
#14958=EDGE_CURVE('',#12089,#12090,#2118,.T.);
#14959=EDGE_CURVE('',#12090,#12091,#2119,.T.);
#14960=EDGE_CURVE('',#12091,#12092,#2120,.T.);
#14961=EDGE_CURVE('',#12092,#12093,#7449,.T.);
#14962=EDGE_CURVE('',#12093,#12094,#2121,.T.);
#14963=EDGE_CURVE('',#12094,#12095,#2122,.T.);
#14964=EDGE_CURVE('',#12095,#12096,#2123,.T.);
#14965=EDGE_CURVE('',#12096,#12097,#2124,.T.);
#14966=EDGE_CURVE('',#12097,#12098,#2125,.T.);
#14967=EDGE_CURVE('',#12098,#12099,#2126,.T.);
#14968=EDGE_CURVE('',#12099,#12100,#2127,.T.);
#14969=EDGE_CURVE('',#12100,#12101,#2128,.T.);
#14970=EDGE_CURVE('',#12101,#12102,#2129,.T.);
#14971=EDGE_CURVE('',#12102,#12103,#2130,.T.);
#14972=EDGE_CURVE('',#12103,#12104,#2131,.T.);
#14973=EDGE_CURVE('',#12104,#12070,#2132,.T.);
#14974=EDGE_CURVE('',#12105,#12106,#2133,.T.);
#14975=EDGE_CURVE('',#12106,#12107,#2134,.T.);
#14976=EDGE_CURVE('',#12107,#12108,#2135,.T.);
#14977=EDGE_CURVE('',#12108,#12109,#7450,.T.);
#14978=EDGE_CURVE('',#12109,#12110,#2136,.T.);
#14979=EDGE_CURVE('',#12110,#12111,#2137,.T.);
#14980=EDGE_CURVE('',#12111,#12112,#2138,.T.);
#14981=EDGE_CURVE('',#12112,#12113,#2139,.T.);
#14982=EDGE_CURVE('',#12113,#12114,#2140,.T.);
#14983=EDGE_CURVE('',#12114,#12115,#2141,.T.);
#14984=EDGE_CURVE('',#12115,#12116,#2142,.T.);
#14985=EDGE_CURVE('',#12116,#12117,#7451,.T.);
#14986=EDGE_CURVE('',#12117,#12118,#2143,.T.);
#14987=EDGE_CURVE('',#12118,#12119,#2144,.T.);
#14988=EDGE_CURVE('',#12119,#12120,#2145,.T.);
#14989=EDGE_CURVE('',#12120,#12121,#2146,.T.);
#14990=EDGE_CURVE('',#12121,#12122,#2147,.T.);
#14991=EDGE_CURVE('',#12122,#12123,#2148,.T.);
#14992=EDGE_CURVE('',#12123,#12124,#2149,.T.);
#14993=EDGE_CURVE('',#12124,#12125,#7452,.T.);
#14994=EDGE_CURVE('',#12125,#12126,#2150,.T.);
#14995=EDGE_CURVE('',#12126,#12127,#2151,.T.);
#14996=EDGE_CURVE('',#12127,#12128,#2152,.T.);
#14997=EDGE_CURVE('',#12128,#12129,#2153,.T.);
#14998=EDGE_CURVE('',#12129,#12130,#2154,.T.);
#14999=EDGE_CURVE('',#12130,#12131,#2155,.T.);
#15000=EDGE_CURVE('',#12131,#12132,#2156,.T.);
#15001=EDGE_CURVE('',#12132,#12133,#2157,.T.);
#15002=EDGE_CURVE('',#12133,#12134,#2158,.T.);
#15003=EDGE_CURVE('',#12134,#12105,#2159,.T.);
#15004=EDGE_CURVE('',#12135,#12136,#7453,.T.);
#15005=EDGE_CURVE('',#12136,#12137,#7454,.T.);
#15006=EDGE_CURVE('',#12137,#12138,#7455,.T.);
#15007=EDGE_CURVE('',#12138,#12135,#7456,.T.);
#15008=EDGE_CURVE('',#12139,#12140,#2160,.T.);
#15009=EDGE_CURVE('',#12140,#12141,#2161,.T.);
#15010=EDGE_CURVE('',#12141,#12142,#2162,.T.);
#15011=EDGE_CURVE('',#12142,#12143,#7457,.T.);
#15012=EDGE_CURVE('',#12143,#12144,#2163,.T.);
#15013=EDGE_CURVE('',#12144,#12145,#2164,.T.);
#15014=EDGE_CURVE('',#12145,#12146,#2165,.T.);
#15015=EDGE_CURVE('',#12146,#12147,#2166,.T.);
#15016=EDGE_CURVE('',#12147,#12148,#2167,.T.);
#15017=EDGE_CURVE('',#12148,#12149,#2168,.T.);
#15018=EDGE_CURVE('',#12149,#12150,#2169,.T.);
#15019=EDGE_CURVE('',#12150,#12151,#2170,.T.);
#15020=EDGE_CURVE('',#12151,#12152,#2171,.T.);
#15021=EDGE_CURVE('',#12152,#12153,#2172,.T.);
#15022=EDGE_CURVE('',#12153,#12154,#2173,.T.);
#15023=EDGE_CURVE('',#12154,#12155,#2174,.T.);
#15024=EDGE_CURVE('',#12155,#12156,#2175,.T.);
#15025=EDGE_CURVE('',#12156,#12157,#2176,.T.);
#15026=EDGE_CURVE('',#12157,#12158,#2177,.T.);
#15027=EDGE_CURVE('',#12158,#12159,#2178,.T.);
#15028=EDGE_CURVE('',#12159,#12160,#2179,.T.);
#15029=EDGE_CURVE('',#12160,#12161,#2180,.T.);
#15030=EDGE_CURVE('',#12161,#12162,#7458,.T.);
#15031=EDGE_CURVE('',#12162,#12163,#2181,.T.);
#15032=EDGE_CURVE('',#12163,#12164,#2182,.T.);
#15033=EDGE_CURVE('',#12164,#12165,#2183,.T.);
#15034=EDGE_CURVE('',#12165,#12166,#2184,.T.);
#15035=EDGE_CURVE('',#12166,#12167,#2185,.T.);
#15036=EDGE_CURVE('',#12167,#12168,#2186,.T.);
#15037=EDGE_CURVE('',#12168,#12169,#2187,.T.);
#15038=EDGE_CURVE('',#12169,#12170,#2188,.T.);
#15039=EDGE_CURVE('',#12170,#12171,#2189,.T.);
#15040=EDGE_CURVE('',#12171,#12172,#2190,.T.);
#15041=EDGE_CURVE('',#12172,#12173,#2191,.T.);
#15042=EDGE_CURVE('',#12173,#12139,#2192,.T.);
#15043=EDGE_CURVE('',#12174,#12175,#7459,.T.);
#15044=EDGE_CURVE('',#12175,#12176,#7460,.T.);
#15045=EDGE_CURVE('',#12176,#12013,#7461,.T.);
#15046=EDGE_CURVE('',#12015,#12174,#7462,.T.);
#15047=EDGE_CURVE('',#12176,#12177,#7463,.T.);
#15048=EDGE_CURVE('',#12177,#12178,#7464,.T.);
#15049=EDGE_CURVE('',#12178,#12014,#7465,.T.);
#15050=EDGE_CURVE('',#12179,#12179,#1036,.T.);
#15051=EDGE_CURVE('',#12179,#12180,#7466,.T.);
#15052=EDGE_CURVE('',#12180,#12180,#1037,.T.);
#15053=EDGE_CURVE('',#12181,#12182,#7467,.T.);
#15054=EDGE_CURVE('',#12183,#12181,#7468,.T.);
#15055=EDGE_CURVE('',#12177,#12183,#7469,.T.);
#15056=EDGE_CURVE('',#12177,#12182,#7470,.T.);
#15057=EDGE_CURVE('',#12184,#12184,#1038,.T.);
#15058=EDGE_CURVE('',#12180,#12185,#7471,.T.);
#15059=EDGE_CURVE('',#12185,#12185,#1039,.T.);
#15060=EDGE_CURVE('',#12184,#12186,#7472,.T.);
#15061=EDGE_CURVE('',#12186,#12186,#1040,.T.);
#15062=EDGE_CURVE('',#12186,#12187,#7473,.T.);
#15063=EDGE_CURVE('',#12187,#12187,#1041,.T.);
#15064=EDGE_CURVE('',#12188,#12188,#1042,.T.);
#15065=EDGE_CURVE('',#12188,#12189,#7474,.T.);
#15066=EDGE_CURVE('',#12189,#12189,#1043,.T.);
#15067=EDGE_CURVE('',#12188,#12190,#7475,.T.);
#15068=EDGE_CURVE('',#12190,#12190,#1044,.T.);
#15069=EDGE_CURVE('',#12191,#12191,#1045,.T.);
#15070=EDGE_CURVE('',#12192,#12192,#1046,.T.);
#15071=EDGE_CURVE('',#12192,#12193,#7476,.T.);
#15072=EDGE_CURVE('',#12193,#12193,#1047,.T.);
#15073=EDGE_CURVE('',#12192,#12194,#7477,.T.);
#15074=EDGE_CURVE('',#12194,#12194,#1048,.T.);
#15075=EDGE_CURVE('',#12195,#12195,#1049,.T.);
#15076=EDGE_CURVE('',#12196,#12196,#1050,.T.);
#15077=EDGE_CURVE('',#12196,#12197,#7478,.T.);
#15078=EDGE_CURVE('',#12197,#12197,#1051,.T.);
#15079=EDGE_CURVE('',#12196,#12198,#7479,.T.);
#15080=EDGE_CURVE('',#12198,#12198,#1052,.T.);
#15081=EDGE_CURVE('',#12199,#12199,#1053,.T.);
#15082=EDGE_CURVE('',#12200,#12200,#1054,.T.);
#15083=EDGE_CURVE('',#12200,#12201,#7480,.T.);
#15084=EDGE_CURVE('',#12201,#12201,#1055,.T.);
#15085=EDGE_CURVE('',#12200,#12202,#7481,.T.);
#15086=EDGE_CURVE('',#12202,#12202,#1056,.T.);
#15087=EDGE_CURVE('',#12203,#12203,#1057,.T.);
#15088=EDGE_CURVE('',#12003,#12204,#7482,.T.);
#15089=EDGE_CURVE('',#12204,#12174,#7483,.T.);
#15090=EDGE_CURVE('',#12204,#12205,#7484,.T.);
#15091=EDGE_CURVE('',#12205,#12182,#7485,.T.);
#15092=EDGE_CURVE('',#12182,#12175,#7486,.T.);
#15093=EDGE_CURVE('',#12206,#12005,#7487,.T.);
#15094=EDGE_CURVE('',#12006,#12206,#7488,.T.);
#15095=EDGE_CURVE('',#12207,#12208,#7489,.T.);
#15096=EDGE_CURVE('',#12181,#12207,#7490,.T.);
#15097=EDGE_CURVE('',#12208,#12181,#7491,.T.);
#15098=EDGE_CURVE('',#12209,#12210,#7492,.T.);
#15099=EDGE_CURVE('',#12211,#12209,#7493,.T.);
#15100=EDGE_CURVE('',#12210,#12211,#7494,.T.);
#15101=EDGE_CURVE('',#12212,#12183,#7495,.T.);
#15102=EDGE_CURVE('',#12213,#12212,#7496,.T.);
#15103=EDGE_CURVE('',#12183,#12213,#7497,.T.);
#15104=EDGE_CURVE('',#12212,#12210,#7498,.T.);
#15105=EDGE_CURVE('',#12211,#12213,#7499,.T.);
#15106=EDGE_CURVE('',#12213,#12178,#7500,.T.);
#15107=EDGE_CURVE('',#12207,#12212,#7501,.T.);
#15108=EDGE_CURVE('',#12011,#12211,#7502,.T.);
#15109=EDGE_CURVE('',#12209,#11998,#7503,.T.);
#15110=EDGE_CURVE('',#12005,#12209,#7504,.T.);
#15111=EDGE_CURVE('',#12210,#12206,#7505,.T.);
#15112=EDGE_CURVE('',#12205,#12208,#7506,.T.);
#15113=EDGE_CURVE('',#12208,#12006,#7507,.T.);
#15114=EDGE_CURVE('',#12206,#12207,#7508,.T.);
#15115=EDGE_CURVE('',#12214,#12214,#1058,.T.);
#15116=EDGE_CURVE('',#12215,#12215,#1059,.T.);
#15117=EDGE_CURVE('',#12216,#12216,#1060,.T.);
#15118=EDGE_CURVE('',#12217,#12217,#1061,.T.);
#15119=EDGE_CURVE('',#12218,#12218,#1062,.T.);
#15120=EDGE_CURVE('',#12219,#12219,#1063,.T.);
#15121=EDGE_CURVE('',#12220,#12220,#1064,.T.);
#15122=EDGE_CURVE('',#12221,#12221,#1065,.T.);
#15123=EDGE_CURVE('',#12222,#12222,#1066,.T.);
#15124=EDGE_CURVE('',#12223,#12223,#1067,.T.);
#15125=EDGE_CURVE('',#12224,#12224,#1068,.T.);
#15126=EDGE_CURVE('',#12225,#12225,#1069,.T.);
#15127=EDGE_CURVE('',#12226,#12226,#1070,.T.);
#15128=EDGE_CURVE('',#12227,#12227,#1071,.T.);
#15129=EDGE_CURVE('',#12228,#12228,#1072,.T.);
#15130=EDGE_CURVE('',#12229,#12229,#1073,.T.);
#15131=EDGE_CURVE('',#12230,#12230,#1074,.T.);
#15132=EDGE_CURVE('',#12231,#12231,#1075,.T.);
#15133=EDGE_CURVE('',#12232,#12232,#1076,.T.);
#15134=EDGE_CURVE('',#12233,#12233,#1077,.T.);
#15135=EDGE_CURVE('',#12234,#12234,#1078,.T.);
#15136=EDGE_CURVE('',#12235,#12235,#1079,.T.);
#15137=EDGE_CURVE('',#12016,#12236,#7509,.T.);
#15138=EDGE_CURVE('',#12236,#12237,#7510,.T.);
#15139=EDGE_CURVE('',#12017,#12237,#7511,.T.);
#15140=EDGE_CURVE('',#12027,#12238,#7512,.T.);
#15141=EDGE_CURVE('',#12238,#12236,#7513,.T.);
#15142=EDGE_CURVE('',#12026,#12239,#7514,.T.);
#15143=EDGE_CURVE('',#12239,#12238,#7515,.T.);
#15144=EDGE_CURVE('',#12025,#12240,#7516,.T.);
#15145=EDGE_CURVE('',#12240,#12239,#7517,.T.);
#15146=EDGE_CURVE('',#12024,#12241,#7518,.T.);
#15147=EDGE_CURVE('',#12241,#12240,#7519,.T.);
#15148=EDGE_CURVE('',#12023,#12242,#7520,.T.);
#15149=EDGE_CURVE('',#12242,#12241,#7521,.T.);
#15150=EDGE_CURVE('',#12022,#12243,#7522,.T.);
#15151=EDGE_CURVE('',#12243,#12242,#7523,.T.);
#15152=EDGE_CURVE('',#12021,#12244,#7524,.T.);
#15153=EDGE_CURVE('',#12244,#12243,#7525,.T.);
#15154=EDGE_CURVE('',#12020,#12245,#7526,.T.);
#15155=EDGE_CURVE('',#12245,#12244,#7527,.T.);
#15156=EDGE_CURVE('',#12019,#12246,#7528,.T.);
#15157=EDGE_CURVE('',#12246,#12245,#7529,.T.);
#15158=EDGE_CURVE('',#12018,#12247,#7530,.T.);
#15159=EDGE_CURVE('',#12247,#12246,#7531,.T.);
#15160=EDGE_CURVE('',#12237,#12247,#7532,.T.);
#15161=EDGE_CURVE('',#12028,#12248,#7533,.T.);
#15162=EDGE_CURVE('',#12248,#12249,#7534,.T.);
#15163=EDGE_CURVE('',#12029,#12249,#7535,.T.);
#15164=EDGE_CURVE('',#12046,#12250,#7536,.T.);
#15165=EDGE_CURVE('',#12250,#12248,#2193,.T.);
#15166=EDGE_CURVE('',#12045,#12251,#7537,.T.);
#15167=EDGE_CURVE('',#12251,#12250,#2194,.T.);
#15168=EDGE_CURVE('',#12044,#12252,#7538,.T.);
#15169=EDGE_CURVE('',#12252,#12251,#2195,.T.);
#15170=EDGE_CURVE('',#12043,#12253,#7539,.T.);
#15171=EDGE_CURVE('',#12253,#12252,#2196,.T.);
#15172=EDGE_CURVE('',#12042,#12254,#7540,.T.);
#15173=EDGE_CURVE('',#12254,#12253,#7541,.T.);
#15174=EDGE_CURVE('',#12041,#12255,#7542,.T.);
#15175=EDGE_CURVE('',#12255,#12254,#7543,.T.);
#15176=EDGE_CURVE('',#12040,#12256,#7544,.T.);
#15177=EDGE_CURVE('',#12256,#12255,#7545,.T.);
#15178=EDGE_CURVE('',#12039,#12257,#7546,.T.);
#15179=EDGE_CURVE('',#12257,#12256,#2197,.T.);
#15180=EDGE_CURVE('',#12038,#12258,#7547,.T.);
#15181=EDGE_CURVE('',#12258,#12257,#2198,.T.);
#15182=EDGE_CURVE('',#12037,#12259,#7548,.T.);
#15183=EDGE_CURVE('',#12259,#12258,#2199,.T.);
#15184=EDGE_CURVE('',#12036,#12260,#7549,.T.);
#15185=EDGE_CURVE('',#12260,#12259,#2200,.T.);
#15186=EDGE_CURVE('',#12035,#12261,#7550,.T.);
#15187=EDGE_CURVE('',#12261,#12260,#2201,.T.);
#15188=EDGE_CURVE('',#12034,#12262,#7551,.T.);
#15189=EDGE_CURVE('',#12262,#12261,#2202,.T.);
#15190=EDGE_CURVE('',#12033,#12263,#7552,.T.);
#15191=EDGE_CURVE('',#12263,#12262,#2203,.T.);
#15192=EDGE_CURVE('',#12032,#12264,#7553,.T.);
#15193=EDGE_CURVE('',#12264,#12263,#7554,.T.);
#15194=EDGE_CURVE('',#12031,#12265,#7555,.T.);
#15195=EDGE_CURVE('',#12265,#12264,#7556,.T.);
#15196=EDGE_CURVE('',#12030,#12266,#7557,.T.);
#15197=EDGE_CURVE('',#12266,#12265,#7558,.T.);
#15198=EDGE_CURVE('',#12249,#12266,#7559,.T.);
#15199=EDGE_CURVE('',#12047,#12267,#7560,.T.);
#15200=EDGE_CURVE('',#12267,#12268,#7561,.T.);
#15201=EDGE_CURVE('',#12048,#12268,#7562,.T.);
#15202=EDGE_CURVE('',#12058,#12269,#7563,.T.);
#15203=EDGE_CURVE('',#12269,#12267,#7564,.T.);
#15204=EDGE_CURVE('',#12057,#12270,#7565,.T.);
#15205=EDGE_CURVE('',#12270,#12269,#7566,.T.);
#15206=EDGE_CURVE('',#12056,#12271,#7567,.T.);
#15207=EDGE_CURVE('',#12271,#12270,#7568,.T.);
#15208=EDGE_CURVE('',#12055,#12272,#7569,.T.);
#15209=EDGE_CURVE('',#12272,#12271,#7570,.T.);
#15210=EDGE_CURVE('',#12054,#12273,#7571,.T.);
#15211=EDGE_CURVE('',#12273,#12272,#7572,.T.);
#15212=EDGE_CURVE('',#12053,#12274,#7573,.T.);
#15213=EDGE_CURVE('',#12274,#12273,#7574,.T.);
#15214=EDGE_CURVE('',#12052,#12275,#7575,.T.);
#15215=EDGE_CURVE('',#12275,#12274,#7576,.T.);
#15216=EDGE_CURVE('',#12051,#12276,#7577,.T.);
#15217=EDGE_CURVE('',#12276,#12275,#7578,.T.);
#15218=EDGE_CURVE('',#12050,#12277,#7579,.T.);
#15219=EDGE_CURVE('',#12277,#12276,#7580,.T.);
#15220=EDGE_CURVE('',#12049,#12278,#7581,.T.);
#15221=EDGE_CURVE('',#12278,#12277,#7582,.T.);
#15222=EDGE_CURVE('',#12268,#12278,#7583,.T.);
#15223=EDGE_CURVE('',#12059,#12279,#7584,.T.);
#15224=EDGE_CURVE('',#12279,#12280,#2204,.T.);
#15225=EDGE_CURVE('',#12060,#12280,#7585,.T.);
#15226=EDGE_CURVE('',#12069,#12281,#7586,.T.);
#15227=EDGE_CURVE('',#12281,#12279,#2205,.T.);
#15228=EDGE_CURVE('',#12068,#12282,#7587,.T.);
#15229=EDGE_CURVE('',#12282,#12281,#7588,.T.);
#15230=EDGE_CURVE('',#12067,#12283,#7589,.T.);
#15231=EDGE_CURVE('',#12283,#12282,#2206,.T.);
#15232=EDGE_CURVE('',#12066,#12284,#7590,.T.);
#15233=EDGE_CURVE('',#12284,#12283,#2207,.T.);
#15234=EDGE_CURVE('',#12065,#12285,#7591,.T.);
#15235=EDGE_CURVE('',#12285,#12284,#2208,.T.);
#15236=EDGE_CURVE('',#12064,#12286,#7592,.T.);
#15237=EDGE_CURVE('',#12286,#12285,#7593,.T.);
#15238=EDGE_CURVE('',#12063,#12287,#7594,.T.);
#15239=EDGE_CURVE('',#12287,#12286,#7595,.T.);
#15240=EDGE_CURVE('',#12062,#12288,#7596,.T.);
#15241=EDGE_CURVE('',#12288,#12287,#7597,.T.);
#15242=EDGE_CURVE('',#12061,#12289,#7598,.T.);
#15243=EDGE_CURVE('',#12289,#12288,#7599,.T.);
#15244=EDGE_CURVE('',#12280,#12289,#2209,.T.);
#15245=EDGE_CURVE('',#12070,#12290,#7600,.T.);
#15246=EDGE_CURVE('',#12290,#12291,#2210,.T.);
#15247=EDGE_CURVE('',#12071,#12291,#7601,.T.);
#15248=EDGE_CURVE('',#12104,#12292,#7602,.T.);
#15249=EDGE_CURVE('',#12292,#12290,#2211,.T.);
#15250=EDGE_CURVE('',#12103,#12293,#7603,.T.);
#15251=EDGE_CURVE('',#12293,#12292,#2212,.T.);
#15252=EDGE_CURVE('',#12102,#12294,#7604,.T.);
#15253=EDGE_CURVE('',#12294,#12293,#2213,.T.);
#15254=EDGE_CURVE('',#12101,#12295,#7605,.T.);
#15255=EDGE_CURVE('',#12295,#12294,#2214,.T.);
#15256=EDGE_CURVE('',#12100,#12296,#7606,.T.);
#15257=EDGE_CURVE('',#12296,#12295,#2215,.T.);
#15258=EDGE_CURVE('',#12099,#12297,#7607,.T.);
#15259=EDGE_CURVE('',#12297,#12296,#2216,.T.);
#15260=EDGE_CURVE('',#12098,#12298,#7608,.T.);
#15261=EDGE_CURVE('',#12298,#12297,#2217,.T.);
#15262=EDGE_CURVE('',#12097,#12299,#7609,.T.);
#15263=EDGE_CURVE('',#12299,#12298,#2218,.T.);
#15264=EDGE_CURVE('',#12096,#12300,#7610,.T.);
#15265=EDGE_CURVE('',#12300,#12299,#2219,.T.);
#15266=EDGE_CURVE('',#12095,#12301,#7611,.T.);
#15267=EDGE_CURVE('',#12301,#12300,#2220,.T.);
#15268=EDGE_CURVE('',#12094,#12302,#7612,.T.);
#15269=EDGE_CURVE('',#12302,#12301,#2221,.T.);
#15270=EDGE_CURVE('',#12093,#12303,#7613,.T.);
#15271=EDGE_CURVE('',#12303,#12302,#2222,.T.);
#15272=EDGE_CURVE('',#12092,#12304,#7614,.T.);
#15273=EDGE_CURVE('',#12304,#12303,#7615,.T.);
#15274=EDGE_CURVE('',#12091,#12305,#7616,.T.);
#15275=EDGE_CURVE('',#12305,#12304,#2223,.T.);
#15276=EDGE_CURVE('',#12090,#12306,#7617,.T.);
#15277=EDGE_CURVE('',#12306,#12305,#2224,.T.);
#15278=EDGE_CURVE('',#12089,#12307,#7618,.T.);
#15279=EDGE_CURVE('',#12307,#12306,#2225,.T.);
#15280=EDGE_CURVE('',#12088,#12308,#7619,.T.);
#15281=EDGE_CURVE('',#12308,#12307,#2226,.T.);
#15282=EDGE_CURVE('',#12087,#12309,#7620,.T.);
#15283=EDGE_CURVE('',#12309,#12308,#2227,.T.);
#15284=EDGE_CURVE('',#12086,#12310,#7621,.T.);
#15285=EDGE_CURVE('',#12310,#12309,#2228,.T.);
#15286=EDGE_CURVE('',#12085,#12311,#7622,.T.);
#15287=EDGE_CURVE('',#12311,#12310,#2229,.T.);
#15288=EDGE_CURVE('',#12084,#12312,#7623,.T.);
#15289=EDGE_CURVE('',#12312,#12311,#2230,.T.);
#15290=EDGE_CURVE('',#12083,#12313,#7624,.T.);
#15291=EDGE_CURVE('',#12313,#12312,#2231,.T.);
#15292=EDGE_CURVE('',#12082,#12314,#7625,.T.);
#15293=EDGE_CURVE('',#12314,#12313,#2232,.T.);
#15294=EDGE_CURVE('',#12081,#12315,#7626,.T.);
#15295=EDGE_CURVE('',#12315,#12314,#2233,.T.);
#15296=EDGE_CURVE('',#12080,#12316,#7627,.T.);
#15297=EDGE_CURVE('',#12316,#12315,#2234,.T.);
#15298=EDGE_CURVE('',#12079,#12317,#7628,.T.);
#15299=EDGE_CURVE('',#12317,#12316,#2235,.T.);
#15300=EDGE_CURVE('',#12078,#12318,#7629,.T.);
#15301=EDGE_CURVE('',#12318,#12317,#2236,.T.);
#15302=EDGE_CURVE('',#12077,#12319,#7630,.T.);
#15303=EDGE_CURVE('',#12319,#12318,#2237,.T.);
#15304=EDGE_CURVE('',#12076,#12320,#7631,.T.);
#15305=EDGE_CURVE('',#12320,#12319,#2238,.T.);
#15306=EDGE_CURVE('',#12075,#12321,#7632,.T.);
#15307=EDGE_CURVE('',#12321,#12320,#2239,.T.);
#15308=EDGE_CURVE('',#12074,#12322,#7633,.T.);
#15309=EDGE_CURVE('',#12322,#12321,#2240,.T.);
#15310=EDGE_CURVE('',#12073,#12323,#7634,.T.);
#15311=EDGE_CURVE('',#12323,#12322,#7635,.T.);
#15312=EDGE_CURVE('',#12072,#12324,#7636,.T.);
#15313=EDGE_CURVE('',#12324,#12323,#2241,.T.);
#15314=EDGE_CURVE('',#12291,#12324,#2242,.T.);
#15315=EDGE_CURVE('',#12105,#12325,#7637,.T.);
#15316=EDGE_CURVE('',#12325,#12326,#2243,.T.);
#15317=EDGE_CURVE('',#12106,#12326,#7638,.T.);
#15318=EDGE_CURVE('',#12134,#12327,#7639,.T.);
#15319=EDGE_CURVE('',#12327,#12325,#2244,.T.);
#15320=EDGE_CURVE('',#12133,#12328,#7640,.T.);
#15321=EDGE_CURVE('',#12328,#12327,#2245,.T.);
#15322=EDGE_CURVE('',#12132,#12329,#7641,.T.);
#15323=EDGE_CURVE('',#12329,#12328,#2246,.T.);
#15324=EDGE_CURVE('',#12131,#12330,#7642,.T.);
#15325=EDGE_CURVE('',#12330,#12329,#2247,.T.);
#15326=EDGE_CURVE('',#12130,#12331,#7643,.T.);
#15327=EDGE_CURVE('',#12331,#12330,#2248,.T.);
#15328=EDGE_CURVE('',#12129,#12332,#7644,.T.);
#15329=EDGE_CURVE('',#12332,#12331,#2249,.T.);
#15330=EDGE_CURVE('',#12128,#12333,#7645,.T.);
#15331=EDGE_CURVE('',#12333,#12332,#2250,.T.);
#15332=EDGE_CURVE('',#12127,#12334,#7646,.T.);
#15333=EDGE_CURVE('',#12334,#12333,#2251,.T.);
#15334=EDGE_CURVE('',#12126,#12335,#7647,.T.);
#15335=EDGE_CURVE('',#12335,#12334,#2252,.T.);
#15336=EDGE_CURVE('',#12125,#12336,#7648,.T.);
#15337=EDGE_CURVE('',#12336,#12335,#2253,.T.);
#15338=EDGE_CURVE('',#12124,#12337,#7649,.T.);
#15339=EDGE_CURVE('',#12337,#12336,#7650,.T.);
#15340=EDGE_CURVE('',#12123,#12338,#7651,.T.);
#15341=EDGE_CURVE('',#12338,#12337,#2254,.T.);
#15342=EDGE_CURVE('',#12122,#12339,#7652,.T.);
#15343=EDGE_CURVE('',#12339,#12338,#2255,.T.);
#15344=EDGE_CURVE('',#12121,#12340,#7653,.T.);
#15345=EDGE_CURVE('',#12340,#12339,#2256,.T.);
#15346=EDGE_CURVE('',#12120,#12341,#7654,.T.);
#15347=EDGE_CURVE('',#12341,#12340,#2257,.T.);
#15348=EDGE_CURVE('',#12119,#12342,#7655,.T.);
#15349=EDGE_CURVE('',#12342,#12341,#2258,.T.);
#15350=EDGE_CURVE('',#12118,#12343,#7656,.T.);
#15351=EDGE_CURVE('',#12343,#12342,#2259,.T.);
#15352=EDGE_CURVE('',#12117,#12344,#7657,.T.);
#15353=EDGE_CURVE('',#12344,#12343,#2260,.T.);
#15354=EDGE_CURVE('',#12116,#12345,#7658,.T.);
#15355=EDGE_CURVE('',#12345,#12344,#7659,.T.);
#15356=EDGE_CURVE('',#12115,#12346,#7660,.T.);
#15357=EDGE_CURVE('',#12346,#12345,#2261,.T.);
#15358=EDGE_CURVE('',#12114,#12347,#7661,.T.);
#15359=EDGE_CURVE('',#12347,#12346,#2262,.T.);
#15360=EDGE_CURVE('',#12113,#12348,#7662,.T.);
#15361=EDGE_CURVE('',#12348,#12347,#2263,.T.);
#15362=EDGE_CURVE('',#12112,#12349,#7663,.T.);
#15363=EDGE_CURVE('',#12349,#12348,#2264,.T.);
#15364=EDGE_CURVE('',#12111,#12350,#7664,.T.);
#15365=EDGE_CURVE('',#12350,#12349,#2265,.T.);
#15366=EDGE_CURVE('',#12110,#12351,#7665,.T.);
#15367=EDGE_CURVE('',#12351,#12350,#2266,.T.);
#15368=EDGE_CURVE('',#12109,#12352,#7666,.T.);
#15369=EDGE_CURVE('',#12352,#12351,#2267,.T.);
#15370=EDGE_CURVE('',#12108,#12353,#7667,.T.);
#15371=EDGE_CURVE('',#12353,#12352,#7668,.T.);
#15372=EDGE_CURVE('',#12107,#12354,#7669,.T.);
#15373=EDGE_CURVE('',#12354,#12353,#2268,.T.);
#15374=EDGE_CURVE('',#12326,#12354,#2269,.T.);
#15375=EDGE_CURVE('',#12135,#12355,#7670,.T.);
#15376=EDGE_CURVE('',#12355,#12356,#7671,.T.);
#15377=EDGE_CURVE('',#12136,#12356,#7672,.T.);
#15378=EDGE_CURVE('',#12138,#12357,#7673,.T.);
#15379=EDGE_CURVE('',#12357,#12355,#7674,.T.);
#15380=EDGE_CURVE('',#12137,#12358,#7675,.T.);
#15381=EDGE_CURVE('',#12358,#12357,#7676,.T.);
#15382=EDGE_CURVE('',#12356,#12358,#7677,.T.);
#15383=EDGE_CURVE('',#12139,#12359,#7678,.T.);
#15384=EDGE_CURVE('',#12359,#12360,#2270,.T.);
#15385=EDGE_CURVE('',#12140,#12360,#7679,.T.);
#15386=EDGE_CURVE('',#12173,#12361,#7680,.T.);
#15387=EDGE_CURVE('',#12361,#12359,#2271,.T.);
#15388=EDGE_CURVE('',#12172,#12362,#7681,.T.);
#15389=EDGE_CURVE('',#12362,#12361,#2272,.T.);
#15390=EDGE_CURVE('',#12171,#12363,#7682,.T.);
#15391=EDGE_CURVE('',#12363,#12362,#2273,.T.);
#15392=EDGE_CURVE('',#12170,#12364,#7683,.T.);
#15393=EDGE_CURVE('',#12364,#12363,#2274,.T.);
#15394=EDGE_CURVE('',#12169,#12365,#7684,.T.);
#15395=EDGE_CURVE('',#12365,#12364,#2275,.T.);
#15396=EDGE_CURVE('',#12168,#12366,#7685,.T.);
#15397=EDGE_CURVE('',#12366,#12365,#2276,.T.);
#15398=EDGE_CURVE('',#12167,#12367,#7686,.T.);
#15399=EDGE_CURVE('',#12367,#12366,#2277,.T.);
#15400=EDGE_CURVE('',#12166,#12368,#7687,.T.);
#15401=EDGE_CURVE('',#12368,#12367,#2278,.T.);
#15402=EDGE_CURVE('',#12165,#12369,#7688,.T.);
#15403=EDGE_CURVE('',#12369,#12368,#2279,.T.);
#15404=EDGE_CURVE('',#12164,#12370,#7689,.T.);
#15405=EDGE_CURVE('',#12370,#12369,#2280,.T.);
#15406=EDGE_CURVE('',#12163,#12371,#7690,.T.);
#15407=EDGE_CURVE('',#12371,#12370,#2281,.T.);
#15408=EDGE_CURVE('',#12162,#12372,#7691,.T.);
#15409=EDGE_CURVE('',#12372,#12371,#2282,.T.);
#15410=EDGE_CURVE('',#12161,#12373,#7692,.T.);
#15411=EDGE_CURVE('',#12373,#12372,#7693,.T.);
#15412=EDGE_CURVE('',#12160,#12374,#7694,.T.);
#15413=EDGE_CURVE('',#12374,#12373,#2283,.T.);
#15414=EDGE_CURVE('',#12159,#12375,#7695,.T.);
#15415=EDGE_CURVE('',#12375,#12374,#2284,.T.);
#15416=EDGE_CURVE('',#12158,#12376,#7696,.T.);
#15417=EDGE_CURVE('',#12376,#12375,#2285,.T.);
#15418=EDGE_CURVE('',#12157,#12377,#7697,.T.);
#15419=EDGE_CURVE('',#12377,#12376,#2286,.T.);
#15420=EDGE_CURVE('',#12156,#12378,#7698,.T.);
#15421=EDGE_CURVE('',#12378,#12377,#2287,.T.);
#15422=EDGE_CURVE('',#12155,#12379,#7699,.T.);
#15423=EDGE_CURVE('',#12379,#12378,#2288,.T.);
#15424=EDGE_CURVE('',#12154,#12380,#7700,.T.);
#15425=EDGE_CURVE('',#12380,#12379,#2289,.T.);
#15426=EDGE_CURVE('',#12153,#12381,#7701,.T.);
#15427=EDGE_CURVE('',#12381,#12380,#2290,.T.);
#15428=EDGE_CURVE('',#12152,#12382,#7702,.T.);
#15429=EDGE_CURVE('',#12382,#12381,#2291,.T.);
#15430=EDGE_CURVE('',#12151,#12383,#7703,.T.);
#15431=EDGE_CURVE('',#12383,#12382,#2292,.T.);
#15432=EDGE_CURVE('',#12150,#12384,#7704,.T.);
#15433=EDGE_CURVE('',#12384,#12383,#2293,.T.);
#15434=EDGE_CURVE('',#12149,#12385,#7705,.T.);
#15435=EDGE_CURVE('',#12385,#12384,#2294,.T.);
#15436=EDGE_CURVE('',#12148,#12386,#7706,.T.);
#15437=EDGE_CURVE('',#12386,#12385,#2295,.T.);
#15438=EDGE_CURVE('',#12147,#12387,#7707,.T.);
#15439=EDGE_CURVE('',#12387,#12386,#2296,.T.);
#15440=EDGE_CURVE('',#12146,#12388,#7708,.T.);
#15441=EDGE_CURVE('',#12388,#12387,#2297,.T.);
#15442=EDGE_CURVE('',#12145,#12389,#7709,.T.);
#15443=EDGE_CURVE('',#12389,#12388,#2298,.T.);
#15444=EDGE_CURVE('',#12144,#12390,#7710,.T.);
#15445=EDGE_CURVE('',#12390,#12389,#2299,.T.);
#15446=EDGE_CURVE('',#12143,#12391,#7711,.T.);
#15447=EDGE_CURVE('',#12391,#12390,#2300,.T.);
#15448=EDGE_CURVE('',#12142,#12392,#7712,.T.);
#15449=EDGE_CURVE('',#12392,#12391,#7713,.T.);
#15450=EDGE_CURVE('',#12141,#12393,#7714,.T.);
#15451=EDGE_CURVE('',#12393,#12392,#2301,.T.);
#15452=EDGE_CURVE('',#12360,#12393,#2302,.T.);
#15453=EDGE_CURVE('',#12231,#12394,#7715,.T.);
#15454=EDGE_CURVE('',#12394,#12394,#1080,.T.);
#15455=EDGE_CURVE('',#12395,#12395,#1081,.T.);
#15456=EDGE_CURVE('',#12395,#12394,#7716,.T.);
#15457=EDGE_CURVE('',#12214,#12396,#7717,.T.);
#15458=EDGE_CURVE('',#12396,#12396,#1082,.T.);
#15459=EDGE_CURVE('',#12396,#12397,#7718,.T.);
#15460=EDGE_CURVE('',#12397,#12397,#1083,.T.);
#15461=EDGE_CURVE('',#12230,#12398,#7719,.T.);
#15462=EDGE_CURVE('',#12398,#12398,#1084,.T.);
#15463=EDGE_CURVE('',#12398,#12399,#7720,.T.);
#15464=EDGE_CURVE('',#12399,#12399,#1085,.T.);
#15465=EDGE_CURVE('',#12215,#12400,#7721,.T.);
#15466=EDGE_CURVE('',#12400,#12400,#1086,.T.);
#15467=EDGE_CURVE('',#12400,#12401,#7722,.T.);
#15468=EDGE_CURVE('',#12401,#12401,#1087,.T.);
#15469=EDGE_CURVE('',#12229,#12402,#7723,.T.);
#15470=EDGE_CURVE('',#12402,#12402,#1088,.T.);
#15471=EDGE_CURVE('',#12402,#12403,#7724,.T.);
#15472=EDGE_CURVE('',#12403,#12403,#1089,.T.);
#15473=EDGE_CURVE('',#12216,#12404,#7725,.T.);
#15474=EDGE_CURVE('',#12404,#12404,#1090,.T.);
#15475=EDGE_CURVE('',#12404,#12405,#7726,.T.);
#15476=EDGE_CURVE('',#12405,#12405,#1091,.T.);
#15477=EDGE_CURVE('',#12228,#12406,#7727,.T.);
#15478=EDGE_CURVE('',#12406,#12406,#1092,.T.);
#15479=EDGE_CURVE('',#12406,#12407,#7728,.T.);
#15480=EDGE_CURVE('',#12407,#12407,#1093,.T.);
#15481=EDGE_CURVE('',#12217,#12408,#7729,.T.);
#15482=EDGE_CURVE('',#12408,#12408,#1094,.T.);
#15483=EDGE_CURVE('',#12408,#12409,#7730,.T.);
#15484=EDGE_CURVE('',#12409,#12409,#1095,.T.);
#15485=EDGE_CURVE('',#12227,#12410,#7731,.T.);
#15486=EDGE_CURVE('',#12410,#12410,#1096,.T.);
#15487=EDGE_CURVE('',#12410,#12411,#7732,.T.);
#15488=EDGE_CURVE('',#12411,#12411,#1097,.T.);
#15489=EDGE_CURVE('',#12218,#12412,#7733,.T.);
#15490=EDGE_CURVE('',#12412,#12412,#1098,.T.);
#15491=EDGE_CURVE('',#12412,#12413,#7734,.T.);
#15492=EDGE_CURVE('',#12413,#12413,#1099,.T.);
#15493=EDGE_CURVE('',#12226,#12414,#7735,.T.);
#15494=EDGE_CURVE('',#12414,#12414,#1100,.T.);
#15495=EDGE_CURVE('',#12414,#12415,#7736,.T.);
#15496=EDGE_CURVE('',#12415,#12415,#1101,.T.);
#15497=EDGE_CURVE('',#12219,#12416,#7737,.T.);
#15498=EDGE_CURVE('',#12416,#12416,#1102,.T.);
#15499=EDGE_CURVE('',#12416,#12417,#7738,.T.);
#15500=EDGE_CURVE('',#12417,#12417,#1103,.T.);
#15501=EDGE_CURVE('',#12225,#12418,#7739,.T.);
#15502=EDGE_CURVE('',#12418,#12418,#1104,.T.);
#15503=EDGE_CURVE('',#12418,#12419,#7740,.T.);
#15504=EDGE_CURVE('',#12419,#12419,#1105,.T.);
#15505=EDGE_CURVE('',#12220,#12420,#7741,.T.);
#15506=EDGE_CURVE('',#12420,#12420,#1106,.T.);
#15507=EDGE_CURVE('',#12420,#12203,#7742,.T.);
#15508=EDGE_CURVE('',#12224,#12421,#7743,.T.);
#15509=EDGE_CURVE('',#12421,#12421,#1107,.T.);
#15510=EDGE_CURVE('',#12421,#12199,#7744,.T.);
#15511=EDGE_CURVE('',#12221,#12422,#7745,.T.);
#15512=EDGE_CURVE('',#12422,#12422,#1108,.T.);
#15513=EDGE_CURVE('',#12422,#12195,#7746,.T.);
#15514=EDGE_CURVE('',#12223,#12423,#7747,.T.);
#15515=EDGE_CURVE('',#12423,#12423,#1109,.T.);
#15516=EDGE_CURVE('',#12423,#12191,#7748,.T.);
#15517=EDGE_CURVE('',#12235,#12202,#7749,.T.);
#15518=EDGE_CURVE('',#12232,#12198,#7750,.T.);
#15519=EDGE_CURVE('',#12234,#12194,#7751,.T.);
#15520=EDGE_CURVE('',#12233,#12190,#7752,.T.);
#15521=EDGE_CURVE('',#12222,#12424,#7753,.T.);
#15522=EDGE_CURVE('',#12424,#12424,#1110,.T.);
#19269=ORIENTED_EDGE('',*,*,#14856,.T.);
#19270=ORIENTED_EDGE('',*,*,#14857,.T.);
#19271=ORIENTED_EDGE('',*,*,#14858,.T.);
#19272=ORIENTED_EDGE('',*,*,#14859,.T.);
#19273=ORIENTED_EDGE('',*,*,#14860,.T.);
#19274=ORIENTED_EDGE('',*,*,#14861,.T.);
#19275=ORIENTED_EDGE('',*,*,#14857,.F.);
#19276=ORIENTED_EDGE('',*,*,#14862,.F.);
#19277=ORIENTED_EDGE('',*,*,#14863,.F.);
#19278=ORIENTED_EDGE('',*,*,#14864,.F.);
#19279=ORIENTED_EDGE('',*,*,#14856,.F.);
#19280=ORIENTED_EDGE('',*,*,#14865,.F.);
#19281=ORIENTED_EDGE('',*,*,#14866,.T.);
#19282=ORIENTED_EDGE('',*,*,#14867,.T.);
#19283=ORIENTED_EDGE('',*,*,#14868,.F.);
#19284=ORIENTED_EDGE('',*,*,#14862,.T.);
#19285=ORIENTED_EDGE('',*,*,#14861,.F.);
#19286=ORIENTED_EDGE('',*,*,#14869,.T.);
#19287=ORIENTED_EDGE('',*,*,#14870,.T.);
#19288=ORIENTED_EDGE('',*,*,#14871,.T.);
#19289=ORIENTED_EDGE('',*,*,#14865,.T.);
#19290=ORIENTED_EDGE('',*,*,#14872,.T.);
#19291=ORIENTED_EDGE('',*,*,#14873,.T.);
#19292=ORIENTED_EDGE('',*,*,#14874,.T.);
#19293=ORIENTED_EDGE('',*,*,#14875,.T.);
#19294=ORIENTED_EDGE('',*,*,#14863,.T.);
#19295=ORIENTED_EDGE('',*,*,#14868,.T.);
#19296=ORIENTED_EDGE('',*,*,#14858,.F.);
#19297=ORIENTED_EDGE('',*,*,#14864,.T.);
#19298=ORIENTED_EDGE('',*,*,#14875,.F.);
#19299=ORIENTED_EDGE('',*,*,#14876,.F.);
#19300=ORIENTED_EDGE('',*,*,#14877,.T.);
#19301=ORIENTED_EDGE('',*,*,#14878,.T.);
#19302=ORIENTED_EDGE('',*,*,#14874,.F.);
#19303=ORIENTED_EDGE('',*,*,#14879,.T.);
#19304=ORIENTED_EDGE('',*,*,#14880,.F.);
#19305=ORIENTED_EDGE('',*,*,#14881,.F.);
#19306=ORIENTED_EDGE('',*,*,#14882,.T.);
#19307=ORIENTED_EDGE('',*,*,#14876,.T.);
#19308=ORIENTED_EDGE('',*,*,#14873,.F.);
#19309=ORIENTED_EDGE('',*,*,#14883,.F.);
#19310=ORIENTED_EDGE('',*,*,#14884,.F.);
#19311=ORIENTED_EDGE('',*,*,#14879,.F.);
#19312=ORIENTED_EDGE('',*,*,#14885,.T.);
#19313=ORIENTED_EDGE('',*,*,#14886,.T.);
#19314=ORIENTED_EDGE('',*,*,#14887,.T.);
#19315=ORIENTED_EDGE('',*,*,#14888,.T.);
#19316=ORIENTED_EDGE('',*,*,#14889,.T.);
#19317=ORIENTED_EDGE('',*,*,#14890,.T.);
#19318=ORIENTED_EDGE('',*,*,#14891,.T.);
#19319=ORIENTED_EDGE('',*,*,#14892,.T.);
#19320=ORIENTED_EDGE('',*,*,#14893,.T.);
#19321=ORIENTED_EDGE('',*,*,#14894,.T.);
#19322=ORIENTED_EDGE('',*,*,#14895,.T.);
#19323=ORIENTED_EDGE('',*,*,#14896,.T.);
#19324=ORIENTED_EDGE('',*,*,#14897,.T.);
#19325=ORIENTED_EDGE('',*,*,#14898,.T.);
#19326=ORIENTED_EDGE('',*,*,#14899,.T.);
#19327=ORIENTED_EDGE('',*,*,#14900,.T.);
#19328=ORIENTED_EDGE('',*,*,#14901,.T.);
#19329=ORIENTED_EDGE('',*,*,#14902,.T.);
#19330=ORIENTED_EDGE('',*,*,#14903,.T.);
#19331=ORIENTED_EDGE('',*,*,#14904,.T.);
#19332=ORIENTED_EDGE('',*,*,#14905,.T.);
#19333=ORIENTED_EDGE('',*,*,#14906,.T.);
#19334=ORIENTED_EDGE('',*,*,#14907,.T.);
#19335=ORIENTED_EDGE('',*,*,#14908,.T.);
#19336=ORIENTED_EDGE('',*,*,#14909,.T.);
#19337=ORIENTED_EDGE('',*,*,#14910,.T.);
#19338=ORIENTED_EDGE('',*,*,#14911,.T.);
#19339=ORIENTED_EDGE('',*,*,#14912,.T.);
#19340=ORIENTED_EDGE('',*,*,#14913,.T.);
#19341=ORIENTED_EDGE('',*,*,#14914,.T.);
#19342=ORIENTED_EDGE('',*,*,#14915,.T.);
#19343=ORIENTED_EDGE('',*,*,#14916,.T.);
#19344=ORIENTED_EDGE('',*,*,#14917,.T.);
#19345=ORIENTED_EDGE('',*,*,#14918,.T.);
#19346=ORIENTED_EDGE('',*,*,#14919,.T.);
#19347=ORIENTED_EDGE('',*,*,#14920,.T.);
#19348=ORIENTED_EDGE('',*,*,#14921,.T.);
#19349=ORIENTED_EDGE('',*,*,#14922,.T.);
#19350=ORIENTED_EDGE('',*,*,#14923,.T.);
#19351=ORIENTED_EDGE('',*,*,#14924,.T.);
#19352=ORIENTED_EDGE('',*,*,#14925,.T.);
#19353=ORIENTED_EDGE('',*,*,#14926,.T.);
#19354=ORIENTED_EDGE('',*,*,#14927,.T.);
#19355=ORIENTED_EDGE('',*,*,#14928,.T.);
#19356=ORIENTED_EDGE('',*,*,#14929,.T.);
#19357=ORIENTED_EDGE('',*,*,#14930,.T.);
#19358=ORIENTED_EDGE('',*,*,#14931,.T.);
#19359=ORIENTED_EDGE('',*,*,#14932,.T.);
#19360=ORIENTED_EDGE('',*,*,#14933,.T.);
#19361=ORIENTED_EDGE('',*,*,#14934,.T.);
#19362=ORIENTED_EDGE('',*,*,#14935,.T.);
#19363=ORIENTED_EDGE('',*,*,#14936,.T.);
#19364=ORIENTED_EDGE('',*,*,#14937,.T.);
#19365=ORIENTED_EDGE('',*,*,#14938,.T.);
#19366=ORIENTED_EDGE('',*,*,#14939,.T.);
#19367=ORIENTED_EDGE('',*,*,#14940,.T.);
#19368=ORIENTED_EDGE('',*,*,#14941,.T.);
#19369=ORIENTED_EDGE('',*,*,#14942,.T.);
#19370=ORIENTED_EDGE('',*,*,#14943,.T.);
#19371=ORIENTED_EDGE('',*,*,#14944,.T.);
#19372=ORIENTED_EDGE('',*,*,#14945,.T.);
#19373=ORIENTED_EDGE('',*,*,#14946,.T.);
#19374=ORIENTED_EDGE('',*,*,#14947,.T.);
#19375=ORIENTED_EDGE('',*,*,#14948,.T.);
#19376=ORIENTED_EDGE('',*,*,#14949,.T.);
#19377=ORIENTED_EDGE('',*,*,#14950,.T.);
#19378=ORIENTED_EDGE('',*,*,#14951,.T.);
#19379=ORIENTED_EDGE('',*,*,#14952,.T.);
#19380=ORIENTED_EDGE('',*,*,#14953,.T.);
#19381=ORIENTED_EDGE('',*,*,#14954,.T.);
#19382=ORIENTED_EDGE('',*,*,#14955,.T.);
#19383=ORIENTED_EDGE('',*,*,#14956,.T.);
#19384=ORIENTED_EDGE('',*,*,#14957,.T.);
#19385=ORIENTED_EDGE('',*,*,#14958,.T.);
#19386=ORIENTED_EDGE('',*,*,#14959,.T.);
#19387=ORIENTED_EDGE('',*,*,#14960,.T.);
#19388=ORIENTED_EDGE('',*,*,#14961,.T.);
#19389=ORIENTED_EDGE('',*,*,#14962,.T.);
#19390=ORIENTED_EDGE('',*,*,#14963,.T.);
#19391=ORIENTED_EDGE('',*,*,#14964,.T.);
#19392=ORIENTED_EDGE('',*,*,#14965,.T.);
#19393=ORIENTED_EDGE('',*,*,#14966,.T.);
#19394=ORIENTED_EDGE('',*,*,#14967,.T.);
#19395=ORIENTED_EDGE('',*,*,#14968,.T.);
#19396=ORIENTED_EDGE('',*,*,#14969,.T.);
#19397=ORIENTED_EDGE('',*,*,#14970,.T.);
#19398=ORIENTED_EDGE('',*,*,#14971,.T.);
#19399=ORIENTED_EDGE('',*,*,#14972,.T.);
#19400=ORIENTED_EDGE('',*,*,#14973,.T.);
#19401=ORIENTED_EDGE('',*,*,#14974,.T.);
#19402=ORIENTED_EDGE('',*,*,#14975,.T.);
#19403=ORIENTED_EDGE('',*,*,#14976,.T.);
#19404=ORIENTED_EDGE('',*,*,#14977,.T.);
#19405=ORIENTED_EDGE('',*,*,#14978,.T.);
#19406=ORIENTED_EDGE('',*,*,#14979,.T.);
#19407=ORIENTED_EDGE('',*,*,#14980,.T.);
#19408=ORIENTED_EDGE('',*,*,#14981,.T.);
#19409=ORIENTED_EDGE('',*,*,#14982,.T.);
#19410=ORIENTED_EDGE('',*,*,#14983,.T.);
#19411=ORIENTED_EDGE('',*,*,#14984,.T.);
#19412=ORIENTED_EDGE('',*,*,#14985,.T.);
#19413=ORIENTED_EDGE('',*,*,#14986,.T.);
#19414=ORIENTED_EDGE('',*,*,#14987,.T.);
#19415=ORIENTED_EDGE('',*,*,#14988,.T.);
#19416=ORIENTED_EDGE('',*,*,#14989,.T.);
#19417=ORIENTED_EDGE('',*,*,#14990,.T.);
#19418=ORIENTED_EDGE('',*,*,#14991,.T.);
#19419=ORIENTED_EDGE('',*,*,#14992,.T.);
#19420=ORIENTED_EDGE('',*,*,#14993,.T.);
#19421=ORIENTED_EDGE('',*,*,#14994,.T.);
#19422=ORIENTED_EDGE('',*,*,#14995,.T.);
#19423=ORIENTED_EDGE('',*,*,#14996,.T.);
#19424=ORIENTED_EDGE('',*,*,#14997,.T.);
#19425=ORIENTED_EDGE('',*,*,#14998,.T.);
#19426=ORIENTED_EDGE('',*,*,#14999,.T.);
#19427=ORIENTED_EDGE('',*,*,#15000,.T.);
#19428=ORIENTED_EDGE('',*,*,#15001,.T.);
#19429=ORIENTED_EDGE('',*,*,#15002,.T.);
#19430=ORIENTED_EDGE('',*,*,#15003,.T.);
#19431=ORIENTED_EDGE('',*,*,#15004,.T.);
#19432=ORIENTED_EDGE('',*,*,#15005,.T.);
#19433=ORIENTED_EDGE('',*,*,#15006,.T.);
#19434=ORIENTED_EDGE('',*,*,#15007,.T.);
#19435=ORIENTED_EDGE('',*,*,#15008,.T.);
#19436=ORIENTED_EDGE('',*,*,#15009,.T.);
#19437=ORIENTED_EDGE('',*,*,#15010,.T.);
#19438=ORIENTED_EDGE('',*,*,#15011,.T.);
#19439=ORIENTED_EDGE('',*,*,#15012,.T.);
#19440=ORIENTED_EDGE('',*,*,#15013,.T.);
#19441=ORIENTED_EDGE('',*,*,#15014,.T.);
#19442=ORIENTED_EDGE('',*,*,#15015,.T.);
#19443=ORIENTED_EDGE('',*,*,#15016,.T.);
#19444=ORIENTED_EDGE('',*,*,#15017,.T.);
#19445=ORIENTED_EDGE('',*,*,#15018,.T.);
#19446=ORIENTED_EDGE('',*,*,#15019,.T.);
#19447=ORIENTED_EDGE('',*,*,#15020,.T.);
#19448=ORIENTED_EDGE('',*,*,#15021,.T.);
#19449=ORIENTED_EDGE('',*,*,#15022,.T.);
#19450=ORIENTED_EDGE('',*,*,#15023,.T.);
#19451=ORIENTED_EDGE('',*,*,#15024,.T.);
#19452=ORIENTED_EDGE('',*,*,#15025,.T.);
#19453=ORIENTED_EDGE('',*,*,#15026,.T.);
#19454=ORIENTED_EDGE('',*,*,#15027,.T.);
#19455=ORIENTED_EDGE('',*,*,#15028,.T.);
#19456=ORIENTED_EDGE('',*,*,#15029,.T.);
#19457=ORIENTED_EDGE('',*,*,#15030,.T.);
#19458=ORIENTED_EDGE('',*,*,#15031,.T.);
#19459=ORIENTED_EDGE('',*,*,#15032,.T.);
#19460=ORIENTED_EDGE('',*,*,#15033,.T.);
#19461=ORIENTED_EDGE('',*,*,#15034,.T.);
#19462=ORIENTED_EDGE('',*,*,#15035,.T.);
#19463=ORIENTED_EDGE('',*,*,#15036,.T.);
#19464=ORIENTED_EDGE('',*,*,#15037,.T.);
#19465=ORIENTED_EDGE('',*,*,#15038,.T.);
#19466=ORIENTED_EDGE('',*,*,#15039,.T.);
#19467=ORIENTED_EDGE('',*,*,#15040,.T.);
#19468=ORIENTED_EDGE('',*,*,#15041,.T.);
#19469=ORIENTED_EDGE('',*,*,#15042,.T.);
#19470=ORIENTED_EDGE('',*,*,#15043,.T.);
#19471=ORIENTED_EDGE('',*,*,#15044,.T.);
#19472=ORIENTED_EDGE('',*,*,#15045,.T.);
#19473=ORIENTED_EDGE('',*,*,#14880,.T.);
#19474=ORIENTED_EDGE('',*,*,#14884,.T.);
#19475=ORIENTED_EDGE('',*,*,#15046,.T.);
#19476=ORIENTED_EDGE('',*,*,#15045,.F.);
#19477=ORIENTED_EDGE('',*,*,#15047,.T.);
#19478=ORIENTED_EDGE('',*,*,#15048,.T.);
#19479=ORIENTED_EDGE('',*,*,#15049,.T.);
#19480=ORIENTED_EDGE('',*,*,#14881,.T.);
#19481=ORIENTED_EDGE('',*,*,#15050,.T.);
#19482=ORIENTED_EDGE('',*,*,#15051,.T.);
#19483=ORIENTED_EDGE('',*,*,#15052,.T.);
#19484=ORIENTED_EDGE('',*,*,#15051,.F.);
#19485=ORIENTED_EDGE('',*,*,#15053,.F.);
#19486=ORIENTED_EDGE('',*,*,#15054,.F.);
#19487=ORIENTED_EDGE('',*,*,#15055,.F.);
#19488=ORIENTED_EDGE('',*,*,#15056,.T.);
#19489=ORIENTED_EDGE('',*,*,#15057,.F.);
#19490=ORIENTED_EDGE('',*,*,#15050,.F.);
#19491=ORIENTED_EDGE('',*,*,#15052,.F.);
#19492=ORIENTED_EDGE('',*,*,#15058,.T.);
#19493=ORIENTED_EDGE('',*,*,#15059,.T.);
#19494=ORIENTED_EDGE('',*,*,#15058,.F.);
#19495=ORIENTED_EDGE('',*,*,#15057,.T.);
#19496=ORIENTED_EDGE('',*,*,#15060,.T.);
#19497=ORIENTED_EDGE('',*,*,#15061,.T.);
#19498=ORIENTED_EDGE('',*,*,#15060,.F.);
#19499=ORIENTED_EDGE('',*,*,#15061,.F.);
#19500=ORIENTED_EDGE('',*,*,#15062,.T.);
#19501=ORIENTED_EDGE('',*,*,#15063,.T.);
#19502=ORIENTED_EDGE('',*,*,#15062,.F.);
#19503=ORIENTED_EDGE('',*,*,#15064,.T.);
#19504=ORIENTED_EDGE('',*,*,#15065,.T.);
#19505=ORIENTED_EDGE('',*,*,#15066,.T.);
#19506=ORIENTED_EDGE('',*,*,#15065,.F.);
#19507=ORIENTED_EDGE('',*,*,#15064,.F.);
#19508=ORIENTED_EDGE('',*,*,#15067,.T.);
#19509=ORIENTED_EDGE('',*,*,#15068,.F.);
#19510=ORIENTED_EDGE('',*,*,#15067,.F.);
#19511=ORIENTED_EDGE('',*,*,#15069,.F.);
#19512=ORIENTED_EDGE('',*,*,#15066,.F.);
#19513=ORIENTED_EDGE('',*,*,#15070,.T.);
#19514=ORIENTED_EDGE('',*,*,#15071,.T.);
#19515=ORIENTED_EDGE('',*,*,#15072,.T.);
#19516=ORIENTED_EDGE('',*,*,#15071,.F.);
#19517=ORIENTED_EDGE('',*,*,#15070,.F.);
#19518=ORIENTED_EDGE('',*,*,#15073,.T.);
#19519=ORIENTED_EDGE('',*,*,#15074,.F.);
#19520=ORIENTED_EDGE('',*,*,#15073,.F.);
#19521=ORIENTED_EDGE('',*,*,#15075,.F.);
#19522=ORIENTED_EDGE('',*,*,#15072,.F.);
#19523=ORIENTED_EDGE('',*,*,#15076,.T.);
#19524=ORIENTED_EDGE('',*,*,#15077,.T.);
#19525=ORIENTED_EDGE('',*,*,#15078,.T.);
#19526=ORIENTED_EDGE('',*,*,#15077,.F.);
#19527=ORIENTED_EDGE('',*,*,#15076,.F.);
#19528=ORIENTED_EDGE('',*,*,#15079,.T.);
#19529=ORIENTED_EDGE('',*,*,#15080,.F.);
#19530=ORIENTED_EDGE('',*,*,#15079,.F.);
#19531=ORIENTED_EDGE('',*,*,#15081,.F.);
#19532=ORIENTED_EDGE('',*,*,#15078,.F.);
#19533=ORIENTED_EDGE('',*,*,#15082,.T.);
#19534=ORIENTED_EDGE('',*,*,#15083,.T.);
#19535=ORIENTED_EDGE('',*,*,#15084,.T.);
#19536=ORIENTED_EDGE('',*,*,#15083,.F.);
#19537=ORIENTED_EDGE('',*,*,#15082,.F.);
#19538=ORIENTED_EDGE('',*,*,#15085,.T.);
#19539=ORIENTED_EDGE('',*,*,#15086,.F.);
#19540=ORIENTED_EDGE('',*,*,#15085,.F.);
#19541=ORIENTED_EDGE('',*,*,#15087,.F.);
#19542=ORIENTED_EDGE('',*,*,#15084,.F.);
#19543=ORIENTED_EDGE('',*,*,#14872,.F.);
#19544=ORIENTED_EDGE('',*,*,#14867,.F.);
#19545=ORIENTED_EDGE('',*,*,#15088,.T.);
#19546=ORIENTED_EDGE('',*,*,#15089,.T.);
#19547=ORIENTED_EDGE('',*,*,#15046,.F.);
#19548=ORIENTED_EDGE('',*,*,#14883,.T.);
#19549=ORIENTED_EDGE('',*,*,#15043,.F.);
#19550=ORIENTED_EDGE('',*,*,#15089,.F.);
#19551=ORIENTED_EDGE('',*,*,#15090,.T.);
#19552=ORIENTED_EDGE('',*,*,#15091,.T.);
#19553=ORIENTED_EDGE('',*,*,#15092,.T.);
#19554=ORIENTED_EDGE('',*,*,#14870,.F.);
#19555=ORIENTED_EDGE('',*,*,#15093,.F.);
#19556=ORIENTED_EDGE('',*,*,#15094,.F.);
#19557=ORIENTED_EDGE('',*,*,#15095,.F.);
#19558=ORIENTED_EDGE('',*,*,#15096,.F.);
#19559=ORIENTED_EDGE('',*,*,#15097,.F.);
#19560=ORIENTED_EDGE('',*,*,#15098,.F.);
#19561=ORIENTED_EDGE('',*,*,#15099,.F.);
#19562=ORIENTED_EDGE('',*,*,#15100,.F.);
#19563=ORIENTED_EDGE('',*,*,#15101,.F.);
#19564=ORIENTED_EDGE('',*,*,#15102,.F.);
#19565=ORIENTED_EDGE('',*,*,#15103,.F.);
#19566=ORIENTED_EDGE('',*,*,#15102,.T.);
#19567=ORIENTED_EDGE('',*,*,#15104,.T.);
#19568=ORIENTED_EDGE('',*,*,#15100,.T.);
#19569=ORIENTED_EDGE('',*,*,#15105,.T.);
#19570=ORIENTED_EDGE('',*,*,#15055,.T.);
#19571=ORIENTED_EDGE('',*,*,#15103,.T.);
#19572=ORIENTED_EDGE('',*,*,#15106,.T.);
#19573=ORIENTED_EDGE('',*,*,#15048,.F.);
#19574=ORIENTED_EDGE('',*,*,#15096,.T.);
#19575=ORIENTED_EDGE('',*,*,#15107,.T.);
#19576=ORIENTED_EDGE('',*,*,#15101,.T.);
#19577=ORIENTED_EDGE('',*,*,#15054,.T.);
#19578=ORIENTED_EDGE('',*,*,#14859,.F.);
#19579=ORIENTED_EDGE('',*,*,#14878,.F.);
#19580=ORIENTED_EDGE('',*,*,#15108,.T.);
#19581=ORIENTED_EDGE('',*,*,#15099,.T.);
#19582=ORIENTED_EDGE('',*,*,#15109,.T.);
#19583=ORIENTED_EDGE('',*,*,#15093,.T.);
#19584=ORIENTED_EDGE('',*,*,#15110,.T.);
#19585=ORIENTED_EDGE('',*,*,#15098,.T.);
#19586=ORIENTED_EDGE('',*,*,#15111,.T.);
#19587=ORIENTED_EDGE('',*,*,#15112,.T.);
#19588=ORIENTED_EDGE('',*,*,#15097,.T.);
#19589=ORIENTED_EDGE('',*,*,#15053,.T.);
#19590=ORIENTED_EDGE('',*,*,#15091,.F.);
#19591=ORIENTED_EDGE('',*,*,#15095,.T.);
#19592=ORIENTED_EDGE('',*,*,#15113,.T.);
#19593=ORIENTED_EDGE('',*,*,#15094,.T.);
#19594=ORIENTED_EDGE('',*,*,#15114,.T.);
#19595=ORIENTED_EDGE('',*,*,#15044,.F.);
#19596=ORIENTED_EDGE('',*,*,#15092,.F.);
#19597=ORIENTED_EDGE('',*,*,#15056,.F.);
#19598=ORIENTED_EDGE('',*,*,#15047,.F.);
#19599=ORIENTED_EDGE('',*,*,#15088,.F.);
#19600=ORIENTED_EDGE('',*,*,#14866,.F.);
#19601=ORIENTED_EDGE('',*,*,#14871,.F.);
#19602=ORIENTED_EDGE('',*,*,#15113,.F.);
#19603=ORIENTED_EDGE('',*,*,#15112,.F.);
#19604=ORIENTED_EDGE('',*,*,#15090,.F.);
#19605=ORIENTED_EDGE('',*,*,#15115,.F.);
#19606=ORIENTED_EDGE('',*,*,#15116,.F.);
#19607=ORIENTED_EDGE('',*,*,#15117,.F.);
#19608=ORIENTED_EDGE('',*,*,#15118,.F.);
#19609=ORIENTED_EDGE('',*,*,#15119,.F.);
#19610=ORIENTED_EDGE('',*,*,#15120,.F.);
#19611=ORIENTED_EDGE('',*,*,#15121,.F.);
#19612=ORIENTED_EDGE('',*,*,#15122,.F.);
#19613=ORIENTED_EDGE('',*,*,#15123,.T.);
#19614=ORIENTED_EDGE('',*,*,#15124,.F.);
#19615=ORIENTED_EDGE('',*,*,#15125,.F.);
#19616=ORIENTED_EDGE('',*,*,#15126,.F.);
#19617=ORIENTED_EDGE('',*,*,#15127,.F.);
#19618=ORIENTED_EDGE('',*,*,#15128,.F.);
#19619=ORIENTED_EDGE('',*,*,#15129,.F.);
#19620=ORIENTED_EDGE('',*,*,#15130,.F.);
#19621=ORIENTED_EDGE('',*,*,#15131,.F.);
#19622=ORIENTED_EDGE('',*,*,#15104,.F.);
#19623=ORIENTED_EDGE('',*,*,#15107,.F.);
#19624=ORIENTED_EDGE('',*,*,#15114,.F.);
#19625=ORIENTED_EDGE('',*,*,#15111,.F.);
#19626=ORIENTED_EDGE('',*,*,#15049,.F.);
#19627=ORIENTED_EDGE('',*,*,#15106,.F.);
#19628=ORIENTED_EDGE('',*,*,#15105,.F.);
#19629=ORIENTED_EDGE('',*,*,#15108,.F.);
#19630=ORIENTED_EDGE('',*,*,#14877,.F.);
#19631=ORIENTED_EDGE('',*,*,#14882,.F.);
#19632=ORIENTED_EDGE('',*,*,#15132,.F.);
#19633=ORIENTED_EDGE('',*,*,#15133,.F.);
#19634=ORIENTED_EDGE('',*,*,#15134,.F.);
#19635=ORIENTED_EDGE('',*,*,#15135,.F.);
#19636=ORIENTED_EDGE('',*,*,#15136,.F.);
#19637=ORIENTED_EDGE('',*,*,#14885,.F.);
#19638=ORIENTED_EDGE('',*,*,#15137,.T.);
#19639=ORIENTED_EDGE('',*,*,#15138,.T.);
#19640=ORIENTED_EDGE('',*,*,#15139,.F.);
#19641=ORIENTED_EDGE('',*,*,#14896,.F.);
#19642=ORIENTED_EDGE('',*,*,#15140,.T.);
#19643=ORIENTED_EDGE('',*,*,#15141,.T.);
#19644=ORIENTED_EDGE('',*,*,#15137,.F.);
#19645=ORIENTED_EDGE('',*,*,#14895,.F.);
#19646=ORIENTED_EDGE('',*,*,#15142,.T.);
#19647=ORIENTED_EDGE('',*,*,#15143,.T.);
#19648=ORIENTED_EDGE('',*,*,#15140,.F.);
#19649=ORIENTED_EDGE('',*,*,#14894,.F.);
#19650=ORIENTED_EDGE('',*,*,#15144,.T.);
#19651=ORIENTED_EDGE('',*,*,#15145,.T.);
#19652=ORIENTED_EDGE('',*,*,#15142,.F.);
#19653=ORIENTED_EDGE('',*,*,#14893,.F.);
#19654=ORIENTED_EDGE('',*,*,#15146,.T.);
#19655=ORIENTED_EDGE('',*,*,#15147,.T.);
#19656=ORIENTED_EDGE('',*,*,#15144,.F.);
#19657=ORIENTED_EDGE('',*,*,#14892,.F.);
#19658=ORIENTED_EDGE('',*,*,#15148,.T.);
#19659=ORIENTED_EDGE('',*,*,#15149,.T.);
#19660=ORIENTED_EDGE('',*,*,#15146,.F.);
#19661=ORIENTED_EDGE('',*,*,#14891,.F.);
#19662=ORIENTED_EDGE('',*,*,#15150,.T.);
#19663=ORIENTED_EDGE('',*,*,#15151,.T.);
#19664=ORIENTED_EDGE('',*,*,#15148,.F.);
#19665=ORIENTED_EDGE('',*,*,#14890,.F.);
#19666=ORIENTED_EDGE('',*,*,#15152,.T.);
#19667=ORIENTED_EDGE('',*,*,#15153,.T.);
#19668=ORIENTED_EDGE('',*,*,#15150,.F.);
#19669=ORIENTED_EDGE('',*,*,#14889,.F.);
#19670=ORIENTED_EDGE('',*,*,#15154,.T.);
#19671=ORIENTED_EDGE('',*,*,#15155,.T.);
#19672=ORIENTED_EDGE('',*,*,#15152,.F.);
#19673=ORIENTED_EDGE('',*,*,#14888,.F.);
#19674=ORIENTED_EDGE('',*,*,#15156,.T.);
#19675=ORIENTED_EDGE('',*,*,#15157,.T.);
#19676=ORIENTED_EDGE('',*,*,#15154,.F.);
#19677=ORIENTED_EDGE('',*,*,#14887,.F.);
#19678=ORIENTED_EDGE('',*,*,#15158,.T.);
#19679=ORIENTED_EDGE('',*,*,#15159,.T.);
#19680=ORIENTED_EDGE('',*,*,#15156,.F.);
#19681=ORIENTED_EDGE('',*,*,#14886,.F.);
#19682=ORIENTED_EDGE('',*,*,#15139,.T.);
#19683=ORIENTED_EDGE('',*,*,#15160,.T.);
#19684=ORIENTED_EDGE('',*,*,#15158,.F.);
#19685=ORIENTED_EDGE('',*,*,#15160,.F.);
#19686=ORIENTED_EDGE('',*,*,#15138,.F.);
#19687=ORIENTED_EDGE('',*,*,#15141,.F.);
#19688=ORIENTED_EDGE('',*,*,#15143,.F.);
#19689=ORIENTED_EDGE('',*,*,#15145,.F.);
#19690=ORIENTED_EDGE('',*,*,#15147,.F.);
#19691=ORIENTED_EDGE('',*,*,#15149,.F.);
#19692=ORIENTED_EDGE('',*,*,#15151,.F.);
#19693=ORIENTED_EDGE('',*,*,#15153,.F.);
#19694=ORIENTED_EDGE('',*,*,#15155,.F.);
#19695=ORIENTED_EDGE('',*,*,#15157,.F.);
#19696=ORIENTED_EDGE('',*,*,#15159,.F.);
#19697=ORIENTED_EDGE('',*,*,#14897,.F.);
#19698=ORIENTED_EDGE('',*,*,#15161,.T.);
#19699=ORIENTED_EDGE('',*,*,#15162,.T.);
#19700=ORIENTED_EDGE('',*,*,#15163,.F.);
#19701=ORIENTED_EDGE('',*,*,#14915,.F.);
#19702=ORIENTED_EDGE('',*,*,#15164,.T.);
#19703=ORIENTED_EDGE('',*,*,#15165,.T.);
#19704=ORIENTED_EDGE('',*,*,#15161,.F.);
#19705=ORIENTED_EDGE('',*,*,#14914,.F.);
#19706=ORIENTED_EDGE('',*,*,#15166,.T.);
#19707=ORIENTED_EDGE('',*,*,#15167,.T.);
#19708=ORIENTED_EDGE('',*,*,#15164,.F.);
#19709=ORIENTED_EDGE('',*,*,#14913,.F.);
#19710=ORIENTED_EDGE('',*,*,#15168,.T.);
#19711=ORIENTED_EDGE('',*,*,#15169,.T.);
#19712=ORIENTED_EDGE('',*,*,#15166,.F.);
#19713=ORIENTED_EDGE('',*,*,#14912,.F.);
#19714=ORIENTED_EDGE('',*,*,#15170,.T.);
#19715=ORIENTED_EDGE('',*,*,#15171,.T.);
#19716=ORIENTED_EDGE('',*,*,#15168,.F.);
#19717=ORIENTED_EDGE('',*,*,#14911,.F.);
#19718=ORIENTED_EDGE('',*,*,#15172,.T.);
#19719=ORIENTED_EDGE('',*,*,#15173,.T.);
#19720=ORIENTED_EDGE('',*,*,#15170,.F.);
#19721=ORIENTED_EDGE('',*,*,#14910,.F.);
#19722=ORIENTED_EDGE('',*,*,#15174,.T.);
#19723=ORIENTED_EDGE('',*,*,#15175,.T.);
#19724=ORIENTED_EDGE('',*,*,#15172,.F.);
#19725=ORIENTED_EDGE('',*,*,#14909,.F.);
#19726=ORIENTED_EDGE('',*,*,#15176,.T.);
#19727=ORIENTED_EDGE('',*,*,#15177,.T.);
#19728=ORIENTED_EDGE('',*,*,#15174,.F.);
#19729=ORIENTED_EDGE('',*,*,#14908,.F.);
#19730=ORIENTED_EDGE('',*,*,#15178,.T.);
#19731=ORIENTED_EDGE('',*,*,#15179,.T.);
#19732=ORIENTED_EDGE('',*,*,#15176,.F.);
#19733=ORIENTED_EDGE('',*,*,#14907,.F.);
#19734=ORIENTED_EDGE('',*,*,#15180,.T.);
#19735=ORIENTED_EDGE('',*,*,#15181,.T.);
#19736=ORIENTED_EDGE('',*,*,#15178,.F.);
#19737=ORIENTED_EDGE('',*,*,#14906,.F.);
#19738=ORIENTED_EDGE('',*,*,#15182,.T.);
#19739=ORIENTED_EDGE('',*,*,#15183,.T.);
#19740=ORIENTED_EDGE('',*,*,#15180,.F.);
#19741=ORIENTED_EDGE('',*,*,#14905,.F.);
#19742=ORIENTED_EDGE('',*,*,#15184,.T.);
#19743=ORIENTED_EDGE('',*,*,#15185,.T.);
#19744=ORIENTED_EDGE('',*,*,#15182,.F.);
#19745=ORIENTED_EDGE('',*,*,#14904,.F.);
#19746=ORIENTED_EDGE('',*,*,#15186,.T.);
#19747=ORIENTED_EDGE('',*,*,#15187,.T.);
#19748=ORIENTED_EDGE('',*,*,#15184,.F.);
#19749=ORIENTED_EDGE('',*,*,#14903,.F.);
#19750=ORIENTED_EDGE('',*,*,#15188,.T.);
#19751=ORIENTED_EDGE('',*,*,#15189,.T.);
#19752=ORIENTED_EDGE('',*,*,#15186,.F.);
#19753=ORIENTED_EDGE('',*,*,#14902,.F.);
#19754=ORIENTED_EDGE('',*,*,#15190,.T.);
#19755=ORIENTED_EDGE('',*,*,#15191,.T.);
#19756=ORIENTED_EDGE('',*,*,#15188,.F.);
#19757=ORIENTED_EDGE('',*,*,#14901,.F.);
#19758=ORIENTED_EDGE('',*,*,#15192,.T.);
#19759=ORIENTED_EDGE('',*,*,#15193,.T.);
#19760=ORIENTED_EDGE('',*,*,#15190,.F.);
#19761=ORIENTED_EDGE('',*,*,#14900,.F.);
#19762=ORIENTED_EDGE('',*,*,#15194,.T.);
#19763=ORIENTED_EDGE('',*,*,#15195,.T.);
#19764=ORIENTED_EDGE('',*,*,#15192,.F.);
#19765=ORIENTED_EDGE('',*,*,#14899,.F.);
#19766=ORIENTED_EDGE('',*,*,#15196,.T.);
#19767=ORIENTED_EDGE('',*,*,#15197,.T.);
#19768=ORIENTED_EDGE('',*,*,#15194,.F.);
#19769=ORIENTED_EDGE('',*,*,#14898,.F.);
#19770=ORIENTED_EDGE('',*,*,#15163,.T.);
#19771=ORIENTED_EDGE('',*,*,#15198,.T.);
#19772=ORIENTED_EDGE('',*,*,#15196,.F.);
#19773=ORIENTED_EDGE('',*,*,#15198,.F.);
#19774=ORIENTED_EDGE('',*,*,#15162,.F.);
#19775=ORIENTED_EDGE('',*,*,#15165,.F.);
#19776=ORIENTED_EDGE('',*,*,#15167,.F.);
#19777=ORIENTED_EDGE('',*,*,#15169,.F.);
#19778=ORIENTED_EDGE('',*,*,#15171,.F.);
#19779=ORIENTED_EDGE('',*,*,#15173,.F.);
#19780=ORIENTED_EDGE('',*,*,#15175,.F.);
#19781=ORIENTED_EDGE('',*,*,#15177,.F.);
#19782=ORIENTED_EDGE('',*,*,#15179,.F.);
#19783=ORIENTED_EDGE('',*,*,#15181,.F.);
#19784=ORIENTED_EDGE('',*,*,#15183,.F.);
#19785=ORIENTED_EDGE('',*,*,#15185,.F.);
#19786=ORIENTED_EDGE('',*,*,#15187,.F.);
#19787=ORIENTED_EDGE('',*,*,#15189,.F.);
#19788=ORIENTED_EDGE('',*,*,#15191,.F.);
#19789=ORIENTED_EDGE('',*,*,#15193,.F.);
#19790=ORIENTED_EDGE('',*,*,#15195,.F.);
#19791=ORIENTED_EDGE('',*,*,#15197,.F.);
#19792=ORIENTED_EDGE('',*,*,#14916,.F.);
#19793=ORIENTED_EDGE('',*,*,#15199,.T.);
#19794=ORIENTED_EDGE('',*,*,#15200,.T.);
#19795=ORIENTED_EDGE('',*,*,#15201,.F.);
#19796=ORIENTED_EDGE('',*,*,#14927,.F.);
#19797=ORIENTED_EDGE('',*,*,#15202,.T.);
#19798=ORIENTED_EDGE('',*,*,#15203,.T.);
#19799=ORIENTED_EDGE('',*,*,#15199,.F.);
#19800=ORIENTED_EDGE('',*,*,#14926,.F.);
#19801=ORIENTED_EDGE('',*,*,#15204,.T.);
#19802=ORIENTED_EDGE('',*,*,#15205,.T.);
#19803=ORIENTED_EDGE('',*,*,#15202,.F.);
#19804=ORIENTED_EDGE('',*,*,#14925,.F.);
#19805=ORIENTED_EDGE('',*,*,#15206,.T.);
#19806=ORIENTED_EDGE('',*,*,#15207,.T.);
#19807=ORIENTED_EDGE('',*,*,#15204,.F.);
#19808=ORIENTED_EDGE('',*,*,#14924,.F.);
#19809=ORIENTED_EDGE('',*,*,#15208,.T.);
#19810=ORIENTED_EDGE('',*,*,#15209,.T.);
#19811=ORIENTED_EDGE('',*,*,#15206,.F.);
#19812=ORIENTED_EDGE('',*,*,#14923,.F.);
#19813=ORIENTED_EDGE('',*,*,#15210,.T.);
#19814=ORIENTED_EDGE('',*,*,#15211,.T.);
#19815=ORIENTED_EDGE('',*,*,#15208,.F.);
#19816=ORIENTED_EDGE('',*,*,#14922,.F.);
#19817=ORIENTED_EDGE('',*,*,#15212,.T.);
#19818=ORIENTED_EDGE('',*,*,#15213,.T.);
#19819=ORIENTED_EDGE('',*,*,#15210,.F.);
#19820=ORIENTED_EDGE('',*,*,#14921,.F.);
#19821=ORIENTED_EDGE('',*,*,#15214,.T.);
#19822=ORIENTED_EDGE('',*,*,#15215,.T.);
#19823=ORIENTED_EDGE('',*,*,#15212,.F.);
#19824=ORIENTED_EDGE('',*,*,#14920,.F.);
#19825=ORIENTED_EDGE('',*,*,#15216,.T.);
#19826=ORIENTED_EDGE('',*,*,#15217,.T.);
#19827=ORIENTED_EDGE('',*,*,#15214,.F.);
#19828=ORIENTED_EDGE('',*,*,#14919,.F.);
#19829=ORIENTED_EDGE('',*,*,#15218,.T.);
#19830=ORIENTED_EDGE('',*,*,#15219,.T.);
#19831=ORIENTED_EDGE('',*,*,#15216,.F.);
#19832=ORIENTED_EDGE('',*,*,#14918,.F.);
#19833=ORIENTED_EDGE('',*,*,#15220,.T.);
#19834=ORIENTED_EDGE('',*,*,#15221,.T.);
#19835=ORIENTED_EDGE('',*,*,#15218,.F.);
#19836=ORIENTED_EDGE('',*,*,#14917,.F.);
#19837=ORIENTED_EDGE('',*,*,#15201,.T.);
#19838=ORIENTED_EDGE('',*,*,#15222,.T.);
#19839=ORIENTED_EDGE('',*,*,#15220,.F.);
#19840=ORIENTED_EDGE('',*,*,#15222,.F.);
#19841=ORIENTED_EDGE('',*,*,#15200,.F.);
#19842=ORIENTED_EDGE('',*,*,#15203,.F.);
#19843=ORIENTED_EDGE('',*,*,#15205,.F.);
#19844=ORIENTED_EDGE('',*,*,#15207,.F.);
#19845=ORIENTED_EDGE('',*,*,#15209,.F.);
#19846=ORIENTED_EDGE('',*,*,#15211,.F.);
#19847=ORIENTED_EDGE('',*,*,#15213,.F.);
#19848=ORIENTED_EDGE('',*,*,#15215,.F.);
#19849=ORIENTED_EDGE('',*,*,#15217,.F.);
#19850=ORIENTED_EDGE('',*,*,#15219,.F.);
#19851=ORIENTED_EDGE('',*,*,#15221,.F.);
#19852=ORIENTED_EDGE('',*,*,#14928,.F.);
#19853=ORIENTED_EDGE('',*,*,#15223,.T.);
#19854=ORIENTED_EDGE('',*,*,#15224,.T.);
#19855=ORIENTED_EDGE('',*,*,#15225,.F.);
#19856=ORIENTED_EDGE('',*,*,#14938,.F.);
#19857=ORIENTED_EDGE('',*,*,#15226,.T.);
#19858=ORIENTED_EDGE('',*,*,#15227,.T.);
#19859=ORIENTED_EDGE('',*,*,#15223,.F.);
#19860=ORIENTED_EDGE('',*,*,#14937,.F.);
#19861=ORIENTED_EDGE('',*,*,#15228,.T.);
#19862=ORIENTED_EDGE('',*,*,#15229,.T.);
#19863=ORIENTED_EDGE('',*,*,#15226,.F.);
#19864=ORIENTED_EDGE('',*,*,#14936,.F.);
#19865=ORIENTED_EDGE('',*,*,#15230,.T.);
#19866=ORIENTED_EDGE('',*,*,#15231,.T.);
#19867=ORIENTED_EDGE('',*,*,#15228,.F.);
#19868=ORIENTED_EDGE('',*,*,#14935,.F.);
#19869=ORIENTED_EDGE('',*,*,#15232,.T.);
#19870=ORIENTED_EDGE('',*,*,#15233,.T.);
#19871=ORIENTED_EDGE('',*,*,#15230,.F.);
#19872=ORIENTED_EDGE('',*,*,#14934,.F.);
#19873=ORIENTED_EDGE('',*,*,#15234,.T.);
#19874=ORIENTED_EDGE('',*,*,#15235,.T.);
#19875=ORIENTED_EDGE('',*,*,#15232,.F.);
#19876=ORIENTED_EDGE('',*,*,#14933,.F.);
#19877=ORIENTED_EDGE('',*,*,#15236,.T.);
#19878=ORIENTED_EDGE('',*,*,#15237,.T.);
#19879=ORIENTED_EDGE('',*,*,#15234,.F.);
#19880=ORIENTED_EDGE('',*,*,#14932,.F.);
#19881=ORIENTED_EDGE('',*,*,#15238,.T.);
#19882=ORIENTED_EDGE('',*,*,#15239,.T.);
#19883=ORIENTED_EDGE('',*,*,#15236,.F.);
#19884=ORIENTED_EDGE('',*,*,#14931,.F.);
#19885=ORIENTED_EDGE('',*,*,#15240,.T.);
#19886=ORIENTED_EDGE('',*,*,#15241,.T.);
#19887=ORIENTED_EDGE('',*,*,#15238,.F.);
#19888=ORIENTED_EDGE('',*,*,#14930,.F.);
#19889=ORIENTED_EDGE('',*,*,#15242,.T.);
#19890=ORIENTED_EDGE('',*,*,#15243,.T.);
#19891=ORIENTED_EDGE('',*,*,#15240,.F.);
#19892=ORIENTED_EDGE('',*,*,#14929,.F.);
#19893=ORIENTED_EDGE('',*,*,#15225,.T.);
#19894=ORIENTED_EDGE('',*,*,#15244,.T.);
#19895=ORIENTED_EDGE('',*,*,#15242,.F.);
#19896=ORIENTED_EDGE('',*,*,#15244,.F.);
#19897=ORIENTED_EDGE('',*,*,#15224,.F.);
#19898=ORIENTED_EDGE('',*,*,#15227,.F.);
#19899=ORIENTED_EDGE('',*,*,#15229,.F.);
#19900=ORIENTED_EDGE('',*,*,#15231,.F.);
#19901=ORIENTED_EDGE('',*,*,#15233,.F.);
#19902=ORIENTED_EDGE('',*,*,#15235,.F.);
#19903=ORIENTED_EDGE('',*,*,#15237,.F.);
#19904=ORIENTED_EDGE('',*,*,#15239,.F.);
#19905=ORIENTED_EDGE('',*,*,#15241,.F.);
#19906=ORIENTED_EDGE('',*,*,#15243,.F.);
#19907=ORIENTED_EDGE('',*,*,#14939,.F.);
#19908=ORIENTED_EDGE('',*,*,#15245,.T.);
#19909=ORIENTED_EDGE('',*,*,#15246,.T.);
#19910=ORIENTED_EDGE('',*,*,#15247,.F.);
#19911=ORIENTED_EDGE('',*,*,#14973,.F.);
#19912=ORIENTED_EDGE('',*,*,#15248,.T.);
#19913=ORIENTED_EDGE('',*,*,#15249,.T.);
#19914=ORIENTED_EDGE('',*,*,#15245,.F.);
#19915=ORIENTED_EDGE('',*,*,#14972,.F.);
#19916=ORIENTED_EDGE('',*,*,#15250,.T.);
#19917=ORIENTED_EDGE('',*,*,#15251,.T.);
#19918=ORIENTED_EDGE('',*,*,#15248,.F.);
#19919=ORIENTED_EDGE('',*,*,#14971,.F.);
#19920=ORIENTED_EDGE('',*,*,#15252,.T.);
#19921=ORIENTED_EDGE('',*,*,#15253,.T.);
#19922=ORIENTED_EDGE('',*,*,#15250,.F.);
#19923=ORIENTED_EDGE('',*,*,#14970,.F.);
#19924=ORIENTED_EDGE('',*,*,#15254,.T.);
#19925=ORIENTED_EDGE('',*,*,#15255,.T.);
#19926=ORIENTED_EDGE('',*,*,#15252,.F.);
#19927=ORIENTED_EDGE('',*,*,#14969,.F.);
#19928=ORIENTED_EDGE('',*,*,#15256,.T.);
#19929=ORIENTED_EDGE('',*,*,#15257,.T.);
#19930=ORIENTED_EDGE('',*,*,#15254,.F.);
#19931=ORIENTED_EDGE('',*,*,#14968,.F.);
#19932=ORIENTED_EDGE('',*,*,#15258,.T.);
#19933=ORIENTED_EDGE('',*,*,#15259,.T.);
#19934=ORIENTED_EDGE('',*,*,#15256,.F.);
#19935=ORIENTED_EDGE('',*,*,#14967,.F.);
#19936=ORIENTED_EDGE('',*,*,#15260,.T.);
#19937=ORIENTED_EDGE('',*,*,#15261,.T.);
#19938=ORIENTED_EDGE('',*,*,#15258,.F.);
#19939=ORIENTED_EDGE('',*,*,#14966,.F.);
#19940=ORIENTED_EDGE('',*,*,#15262,.T.);
#19941=ORIENTED_EDGE('',*,*,#15263,.T.);
#19942=ORIENTED_EDGE('',*,*,#15260,.F.);
#19943=ORIENTED_EDGE('',*,*,#14965,.F.);
#19944=ORIENTED_EDGE('',*,*,#15264,.T.);
#19945=ORIENTED_EDGE('',*,*,#15265,.T.);
#19946=ORIENTED_EDGE('',*,*,#15262,.F.);
#19947=ORIENTED_EDGE('',*,*,#14964,.F.);
#19948=ORIENTED_EDGE('',*,*,#15266,.T.);
#19949=ORIENTED_EDGE('',*,*,#15267,.T.);
#19950=ORIENTED_EDGE('',*,*,#15264,.F.);
#19951=ORIENTED_EDGE('',*,*,#14963,.F.);
#19952=ORIENTED_EDGE('',*,*,#15268,.T.);
#19953=ORIENTED_EDGE('',*,*,#15269,.T.);
#19954=ORIENTED_EDGE('',*,*,#15266,.F.);
#19955=ORIENTED_EDGE('',*,*,#14962,.F.);
#19956=ORIENTED_EDGE('',*,*,#15270,.T.);
#19957=ORIENTED_EDGE('',*,*,#15271,.T.);
#19958=ORIENTED_EDGE('',*,*,#15268,.F.);
#19959=ORIENTED_EDGE('',*,*,#14961,.F.);
#19960=ORIENTED_EDGE('',*,*,#15272,.T.);
#19961=ORIENTED_EDGE('',*,*,#15273,.T.);
#19962=ORIENTED_EDGE('',*,*,#15270,.F.);
#19963=ORIENTED_EDGE('',*,*,#14960,.F.);
#19964=ORIENTED_EDGE('',*,*,#15274,.T.);
#19965=ORIENTED_EDGE('',*,*,#15275,.T.);
#19966=ORIENTED_EDGE('',*,*,#15272,.F.);
#19967=ORIENTED_EDGE('',*,*,#14959,.F.);
#19968=ORIENTED_EDGE('',*,*,#15276,.T.);
#19969=ORIENTED_EDGE('',*,*,#15277,.T.);
#19970=ORIENTED_EDGE('',*,*,#15274,.F.);
#19971=ORIENTED_EDGE('',*,*,#14958,.F.);
#19972=ORIENTED_EDGE('',*,*,#15278,.T.);
#19973=ORIENTED_EDGE('',*,*,#15279,.T.);
#19974=ORIENTED_EDGE('',*,*,#15276,.F.);
#19975=ORIENTED_EDGE('',*,*,#14957,.F.);
#19976=ORIENTED_EDGE('',*,*,#15280,.T.);
#19977=ORIENTED_EDGE('',*,*,#15281,.T.);
#19978=ORIENTED_EDGE('',*,*,#15278,.F.);
#19979=ORIENTED_EDGE('',*,*,#14956,.F.);
#19980=ORIENTED_EDGE('',*,*,#15282,.T.);
#19981=ORIENTED_EDGE('',*,*,#15283,.T.);
#19982=ORIENTED_EDGE('',*,*,#15280,.F.);
#19983=ORIENTED_EDGE('',*,*,#14955,.F.);
#19984=ORIENTED_EDGE('',*,*,#15284,.T.);
#19985=ORIENTED_EDGE('',*,*,#15285,.T.);
#19986=ORIENTED_EDGE('',*,*,#15282,.F.);
#19987=ORIENTED_EDGE('',*,*,#14954,.F.);
#19988=ORIENTED_EDGE('',*,*,#15286,.T.);
#19989=ORIENTED_EDGE('',*,*,#15287,.T.);
#19990=ORIENTED_EDGE('',*,*,#15284,.F.);
#19991=ORIENTED_EDGE('',*,*,#14953,.F.);
#19992=ORIENTED_EDGE('',*,*,#15288,.T.);
#19993=ORIENTED_EDGE('',*,*,#15289,.T.);
#19994=ORIENTED_EDGE('',*,*,#15286,.F.);
#19995=ORIENTED_EDGE('',*,*,#14952,.F.);
#19996=ORIENTED_EDGE('',*,*,#15290,.T.);
#19997=ORIENTED_EDGE('',*,*,#15291,.T.);
#19998=ORIENTED_EDGE('',*,*,#15288,.F.);
#19999=ORIENTED_EDGE('',*,*,#14951,.F.);
#20000=ORIENTED_EDGE('',*,*,#15292,.T.);
#20001=ORIENTED_EDGE('',*,*,#15293,.T.);
#20002=ORIENTED_EDGE('',*,*,#15290,.F.);
#20003=ORIENTED_EDGE('',*,*,#14950,.F.);
#20004=ORIENTED_EDGE('',*,*,#15294,.T.);
#20005=ORIENTED_EDGE('',*,*,#15295,.T.);
#20006=ORIENTED_EDGE('',*,*,#15292,.F.);
#20007=ORIENTED_EDGE('',*,*,#14949,.F.);
#20008=ORIENTED_EDGE('',*,*,#15296,.T.);
#20009=ORIENTED_EDGE('',*,*,#15297,.T.);
#20010=ORIENTED_EDGE('',*,*,#15294,.F.);
#20011=ORIENTED_EDGE('',*,*,#14948,.F.);
#20012=ORIENTED_EDGE('',*,*,#15298,.T.);
#20013=ORIENTED_EDGE('',*,*,#15299,.T.);
#20014=ORIENTED_EDGE('',*,*,#15296,.F.);
#20015=ORIENTED_EDGE('',*,*,#14947,.F.);
#20016=ORIENTED_EDGE('',*,*,#15300,.T.);
#20017=ORIENTED_EDGE('',*,*,#15301,.T.);
#20018=ORIENTED_EDGE('',*,*,#15298,.F.);
#20019=ORIENTED_EDGE('',*,*,#14946,.F.);
#20020=ORIENTED_EDGE('',*,*,#15302,.T.);
#20021=ORIENTED_EDGE('',*,*,#15303,.T.);
#20022=ORIENTED_EDGE('',*,*,#15300,.F.);
#20023=ORIENTED_EDGE('',*,*,#14945,.F.);
#20024=ORIENTED_EDGE('',*,*,#15304,.T.);
#20025=ORIENTED_EDGE('',*,*,#15305,.T.);
#20026=ORIENTED_EDGE('',*,*,#15302,.F.);
#20027=ORIENTED_EDGE('',*,*,#14944,.F.);
#20028=ORIENTED_EDGE('',*,*,#15306,.T.);
#20029=ORIENTED_EDGE('',*,*,#15307,.T.);
#20030=ORIENTED_EDGE('',*,*,#15304,.F.);
#20031=ORIENTED_EDGE('',*,*,#14943,.F.);
#20032=ORIENTED_EDGE('',*,*,#15308,.T.);
#20033=ORIENTED_EDGE('',*,*,#15309,.T.);
#20034=ORIENTED_EDGE('',*,*,#15306,.F.);
#20035=ORIENTED_EDGE('',*,*,#14942,.F.);
#20036=ORIENTED_EDGE('',*,*,#15310,.T.);
#20037=ORIENTED_EDGE('',*,*,#15311,.T.);
#20038=ORIENTED_EDGE('',*,*,#15308,.F.);
#20039=ORIENTED_EDGE('',*,*,#14941,.F.);
#20040=ORIENTED_EDGE('',*,*,#15312,.T.);
#20041=ORIENTED_EDGE('',*,*,#15313,.T.);
#20042=ORIENTED_EDGE('',*,*,#15310,.F.);
#20043=ORIENTED_EDGE('',*,*,#14940,.F.);
#20044=ORIENTED_EDGE('',*,*,#15247,.T.);
#20045=ORIENTED_EDGE('',*,*,#15314,.T.);
#20046=ORIENTED_EDGE('',*,*,#15312,.F.);
#20047=ORIENTED_EDGE('',*,*,#15314,.F.);
#20048=ORIENTED_EDGE('',*,*,#15246,.F.);
#20049=ORIENTED_EDGE('',*,*,#15249,.F.);
#20050=ORIENTED_EDGE('',*,*,#15251,.F.);
#20051=ORIENTED_EDGE('',*,*,#15253,.F.);
#20052=ORIENTED_EDGE('',*,*,#15255,.F.);
#20053=ORIENTED_EDGE('',*,*,#15257,.F.);
#20054=ORIENTED_EDGE('',*,*,#15259,.F.);
#20055=ORIENTED_EDGE('',*,*,#15261,.F.);
#20056=ORIENTED_EDGE('',*,*,#15263,.F.);
#20057=ORIENTED_EDGE('',*,*,#15265,.F.);
#20058=ORIENTED_EDGE('',*,*,#15267,.F.);
#20059=ORIENTED_EDGE('',*,*,#15269,.F.);
#20060=ORIENTED_EDGE('',*,*,#15271,.F.);
#20061=ORIENTED_EDGE('',*,*,#15273,.F.);
#20062=ORIENTED_EDGE('',*,*,#15275,.F.);
#20063=ORIENTED_EDGE('',*,*,#15277,.F.);
#20064=ORIENTED_EDGE('',*,*,#15279,.F.);
#20065=ORIENTED_EDGE('',*,*,#15281,.F.);
#20066=ORIENTED_EDGE('',*,*,#15283,.F.);
#20067=ORIENTED_EDGE('',*,*,#15285,.F.);
#20068=ORIENTED_EDGE('',*,*,#15287,.F.);
#20069=ORIENTED_EDGE('',*,*,#15289,.F.);
#20070=ORIENTED_EDGE('',*,*,#15291,.F.);
#20071=ORIENTED_EDGE('',*,*,#15293,.F.);
#20072=ORIENTED_EDGE('',*,*,#15295,.F.);
#20073=ORIENTED_EDGE('',*,*,#15297,.F.);
#20074=ORIENTED_EDGE('',*,*,#15299,.F.);
#20075=ORIENTED_EDGE('',*,*,#15301,.F.);
#20076=ORIENTED_EDGE('',*,*,#15303,.F.);
#20077=ORIENTED_EDGE('',*,*,#15305,.F.);
#20078=ORIENTED_EDGE('',*,*,#15307,.F.);
#20079=ORIENTED_EDGE('',*,*,#15309,.F.);
#20080=ORIENTED_EDGE('',*,*,#15311,.F.);
#20081=ORIENTED_EDGE('',*,*,#15313,.F.);
#20082=ORIENTED_EDGE('',*,*,#14974,.F.);
#20083=ORIENTED_EDGE('',*,*,#15315,.T.);
#20084=ORIENTED_EDGE('',*,*,#15316,.T.);
#20085=ORIENTED_EDGE('',*,*,#15317,.F.);
#20086=ORIENTED_EDGE('',*,*,#15003,.F.);
#20087=ORIENTED_EDGE('',*,*,#15318,.T.);
#20088=ORIENTED_EDGE('',*,*,#15319,.T.);
#20089=ORIENTED_EDGE('',*,*,#15315,.F.);
#20090=ORIENTED_EDGE('',*,*,#15002,.F.);
#20091=ORIENTED_EDGE('',*,*,#15320,.T.);
#20092=ORIENTED_EDGE('',*,*,#15321,.T.);
#20093=ORIENTED_EDGE('',*,*,#15318,.F.);
#20094=ORIENTED_EDGE('',*,*,#15001,.F.);
#20095=ORIENTED_EDGE('',*,*,#15322,.T.);
#20096=ORIENTED_EDGE('',*,*,#15323,.T.);
#20097=ORIENTED_EDGE('',*,*,#15320,.F.);
#20098=ORIENTED_EDGE('',*,*,#15000,.F.);
#20099=ORIENTED_EDGE('',*,*,#15324,.T.);
#20100=ORIENTED_EDGE('',*,*,#15325,.T.);
#20101=ORIENTED_EDGE('',*,*,#15322,.F.);
#20102=ORIENTED_EDGE('',*,*,#14999,.F.);
#20103=ORIENTED_EDGE('',*,*,#15326,.T.);
#20104=ORIENTED_EDGE('',*,*,#15327,.T.);
#20105=ORIENTED_EDGE('',*,*,#15324,.F.);
#20106=ORIENTED_EDGE('',*,*,#14998,.F.);
#20107=ORIENTED_EDGE('',*,*,#15328,.T.);
#20108=ORIENTED_EDGE('',*,*,#15329,.T.);
#20109=ORIENTED_EDGE('',*,*,#15326,.F.);
#20110=ORIENTED_EDGE('',*,*,#14997,.F.);
#20111=ORIENTED_EDGE('',*,*,#15330,.T.);
#20112=ORIENTED_EDGE('',*,*,#15331,.T.);
#20113=ORIENTED_EDGE('',*,*,#15328,.F.);
#20114=ORIENTED_EDGE('',*,*,#14996,.F.);
#20115=ORIENTED_EDGE('',*,*,#15332,.T.);
#20116=ORIENTED_EDGE('',*,*,#15333,.T.);
#20117=ORIENTED_EDGE('',*,*,#15330,.F.);
#20118=ORIENTED_EDGE('',*,*,#14995,.F.);
#20119=ORIENTED_EDGE('',*,*,#15334,.T.);
#20120=ORIENTED_EDGE('',*,*,#15335,.T.);
#20121=ORIENTED_EDGE('',*,*,#15332,.F.);
#20122=ORIENTED_EDGE('',*,*,#14994,.F.);
#20123=ORIENTED_EDGE('',*,*,#15336,.T.);
#20124=ORIENTED_EDGE('',*,*,#15337,.T.);
#20125=ORIENTED_EDGE('',*,*,#15334,.F.);
#20126=ORIENTED_EDGE('',*,*,#14993,.F.);
#20127=ORIENTED_EDGE('',*,*,#15338,.T.);
#20128=ORIENTED_EDGE('',*,*,#15339,.T.);
#20129=ORIENTED_EDGE('',*,*,#15336,.F.);
#20130=ORIENTED_EDGE('',*,*,#14992,.F.);
#20131=ORIENTED_EDGE('',*,*,#15340,.T.);
#20132=ORIENTED_EDGE('',*,*,#15341,.T.);
#20133=ORIENTED_EDGE('',*,*,#15338,.F.);
#20134=ORIENTED_EDGE('',*,*,#14991,.F.);
#20135=ORIENTED_EDGE('',*,*,#15342,.T.);
#20136=ORIENTED_EDGE('',*,*,#15343,.T.);
#20137=ORIENTED_EDGE('',*,*,#15340,.F.);
#20138=ORIENTED_EDGE('',*,*,#14990,.F.);
#20139=ORIENTED_EDGE('',*,*,#15344,.T.);
#20140=ORIENTED_EDGE('',*,*,#15345,.T.);
#20141=ORIENTED_EDGE('',*,*,#15342,.F.);
#20142=ORIENTED_EDGE('',*,*,#14989,.F.);
#20143=ORIENTED_EDGE('',*,*,#15346,.T.);
#20144=ORIENTED_EDGE('',*,*,#15347,.T.);
#20145=ORIENTED_EDGE('',*,*,#15344,.F.);
#20146=ORIENTED_EDGE('',*,*,#14988,.F.);
#20147=ORIENTED_EDGE('',*,*,#15348,.T.);
#20148=ORIENTED_EDGE('',*,*,#15349,.T.);
#20149=ORIENTED_EDGE('',*,*,#15346,.F.);
#20150=ORIENTED_EDGE('',*,*,#14987,.F.);
#20151=ORIENTED_EDGE('',*,*,#15350,.T.);
#20152=ORIENTED_EDGE('',*,*,#15351,.T.);
#20153=ORIENTED_EDGE('',*,*,#15348,.F.);
#20154=ORIENTED_EDGE('',*,*,#14986,.F.);
#20155=ORIENTED_EDGE('',*,*,#15352,.T.);
#20156=ORIENTED_EDGE('',*,*,#15353,.T.);
#20157=ORIENTED_EDGE('',*,*,#15350,.F.);
#20158=ORIENTED_EDGE('',*,*,#14985,.F.);
#20159=ORIENTED_EDGE('',*,*,#15354,.T.);
#20160=ORIENTED_EDGE('',*,*,#15355,.T.);
#20161=ORIENTED_EDGE('',*,*,#15352,.F.);
#20162=ORIENTED_EDGE('',*,*,#14984,.F.);
#20163=ORIENTED_EDGE('',*,*,#15356,.T.);
#20164=ORIENTED_EDGE('',*,*,#15357,.T.);
#20165=ORIENTED_EDGE('',*,*,#15354,.F.);
#20166=ORIENTED_EDGE('',*,*,#14983,.F.);
#20167=ORIENTED_EDGE('',*,*,#15358,.T.);
#20168=ORIENTED_EDGE('',*,*,#15359,.T.);
#20169=ORIENTED_EDGE('',*,*,#15356,.F.);
#20170=ORIENTED_EDGE('',*,*,#14982,.F.);
#20171=ORIENTED_EDGE('',*,*,#15360,.T.);
#20172=ORIENTED_EDGE('',*,*,#15361,.T.);
#20173=ORIENTED_EDGE('',*,*,#15358,.F.);
#20174=ORIENTED_EDGE('',*,*,#14981,.F.);
#20175=ORIENTED_EDGE('',*,*,#15362,.T.);
#20176=ORIENTED_EDGE('',*,*,#15363,.T.);
#20177=ORIENTED_EDGE('',*,*,#15360,.F.);
#20178=ORIENTED_EDGE('',*,*,#14980,.F.);
#20179=ORIENTED_EDGE('',*,*,#15364,.T.);
#20180=ORIENTED_EDGE('',*,*,#15365,.T.);
#20181=ORIENTED_EDGE('',*,*,#15362,.F.);
#20182=ORIENTED_EDGE('',*,*,#14979,.F.);
#20183=ORIENTED_EDGE('',*,*,#15366,.T.);
#20184=ORIENTED_EDGE('',*,*,#15367,.T.);
#20185=ORIENTED_EDGE('',*,*,#15364,.F.);
#20186=ORIENTED_EDGE('',*,*,#14978,.F.);
#20187=ORIENTED_EDGE('',*,*,#15368,.T.);
#20188=ORIENTED_EDGE('',*,*,#15369,.T.);
#20189=ORIENTED_EDGE('',*,*,#15366,.F.);
#20190=ORIENTED_EDGE('',*,*,#14977,.F.);
#20191=ORIENTED_EDGE('',*,*,#15370,.T.);
#20192=ORIENTED_EDGE('',*,*,#15371,.T.);
#20193=ORIENTED_EDGE('',*,*,#15368,.F.);
#20194=ORIENTED_EDGE('',*,*,#14976,.F.);
#20195=ORIENTED_EDGE('',*,*,#15372,.T.);
#20196=ORIENTED_EDGE('',*,*,#15373,.T.);
#20197=ORIENTED_EDGE('',*,*,#15370,.F.);
#20198=ORIENTED_EDGE('',*,*,#14975,.F.);
#20199=ORIENTED_EDGE('',*,*,#15317,.T.);
#20200=ORIENTED_EDGE('',*,*,#15374,.T.);
#20201=ORIENTED_EDGE('',*,*,#15372,.F.);
#20202=ORIENTED_EDGE('',*,*,#15374,.F.);
#20203=ORIENTED_EDGE('',*,*,#15316,.F.);
#20204=ORIENTED_EDGE('',*,*,#15319,.F.);
#20205=ORIENTED_EDGE('',*,*,#15321,.F.);
#20206=ORIENTED_EDGE('',*,*,#15323,.F.);
#20207=ORIENTED_EDGE('',*,*,#15325,.F.);
#20208=ORIENTED_EDGE('',*,*,#15327,.F.);
#20209=ORIENTED_EDGE('',*,*,#15329,.F.);
#20210=ORIENTED_EDGE('',*,*,#15331,.F.);
#20211=ORIENTED_EDGE('',*,*,#15333,.F.);
#20212=ORIENTED_EDGE('',*,*,#15335,.F.);
#20213=ORIENTED_EDGE('',*,*,#15337,.F.);
#20214=ORIENTED_EDGE('',*,*,#15339,.F.);
#20215=ORIENTED_EDGE('',*,*,#15341,.F.);
#20216=ORIENTED_EDGE('',*,*,#15343,.F.);
#20217=ORIENTED_EDGE('',*,*,#15345,.F.);
#20218=ORIENTED_EDGE('',*,*,#15347,.F.);
#20219=ORIENTED_EDGE('',*,*,#15349,.F.);
#20220=ORIENTED_EDGE('',*,*,#15351,.F.);
#20221=ORIENTED_EDGE('',*,*,#15353,.F.);
#20222=ORIENTED_EDGE('',*,*,#15355,.F.);
#20223=ORIENTED_EDGE('',*,*,#15357,.F.);
#20224=ORIENTED_EDGE('',*,*,#15359,.F.);
#20225=ORIENTED_EDGE('',*,*,#15361,.F.);
#20226=ORIENTED_EDGE('',*,*,#15363,.F.);
#20227=ORIENTED_EDGE('',*,*,#15365,.F.);
#20228=ORIENTED_EDGE('',*,*,#15367,.F.);
#20229=ORIENTED_EDGE('',*,*,#15369,.F.);
#20230=ORIENTED_EDGE('',*,*,#15371,.F.);
#20231=ORIENTED_EDGE('',*,*,#15373,.F.);
#20232=ORIENTED_EDGE('',*,*,#15004,.F.);
#20233=ORIENTED_EDGE('',*,*,#15375,.T.);
#20234=ORIENTED_EDGE('',*,*,#15376,.T.);
#20235=ORIENTED_EDGE('',*,*,#15377,.F.);
#20236=ORIENTED_EDGE('',*,*,#15007,.F.);
#20237=ORIENTED_EDGE('',*,*,#15378,.T.);
#20238=ORIENTED_EDGE('',*,*,#15379,.T.);
#20239=ORIENTED_EDGE('',*,*,#15375,.F.);
#20240=ORIENTED_EDGE('',*,*,#15006,.F.);
#20241=ORIENTED_EDGE('',*,*,#15380,.T.);
#20242=ORIENTED_EDGE('',*,*,#15381,.T.);
#20243=ORIENTED_EDGE('',*,*,#15378,.F.);
#20244=ORIENTED_EDGE('',*,*,#15005,.F.);
#20245=ORIENTED_EDGE('',*,*,#15377,.T.);
#20246=ORIENTED_EDGE('',*,*,#15382,.T.);
#20247=ORIENTED_EDGE('',*,*,#15380,.F.);
#20248=ORIENTED_EDGE('',*,*,#15382,.F.);
#20249=ORIENTED_EDGE('',*,*,#15376,.F.);
#20250=ORIENTED_EDGE('',*,*,#15379,.F.);
#20251=ORIENTED_EDGE('',*,*,#15381,.F.);
#20252=ORIENTED_EDGE('',*,*,#15008,.F.);
#20253=ORIENTED_EDGE('',*,*,#15383,.T.);
#20254=ORIENTED_EDGE('',*,*,#15384,.T.);
#20255=ORIENTED_EDGE('',*,*,#15385,.F.);
#20256=ORIENTED_EDGE('',*,*,#15042,.F.);
#20257=ORIENTED_EDGE('',*,*,#15386,.T.);
#20258=ORIENTED_EDGE('',*,*,#15387,.T.);
#20259=ORIENTED_EDGE('',*,*,#15383,.F.);
#20260=ORIENTED_EDGE('',*,*,#15041,.F.);
#20261=ORIENTED_EDGE('',*,*,#15388,.T.);
#20262=ORIENTED_EDGE('',*,*,#15389,.T.);
#20263=ORIENTED_EDGE('',*,*,#15386,.F.);
#20264=ORIENTED_EDGE('',*,*,#15040,.F.);
#20265=ORIENTED_EDGE('',*,*,#15390,.T.);
#20266=ORIENTED_EDGE('',*,*,#15391,.T.);
#20267=ORIENTED_EDGE('',*,*,#15388,.F.);
#20268=ORIENTED_EDGE('',*,*,#15039,.F.);
#20269=ORIENTED_EDGE('',*,*,#15392,.T.);
#20270=ORIENTED_EDGE('',*,*,#15393,.T.);
#20271=ORIENTED_EDGE('',*,*,#15390,.F.);
#20272=ORIENTED_EDGE('',*,*,#15038,.F.);
#20273=ORIENTED_EDGE('',*,*,#15394,.T.);
#20274=ORIENTED_EDGE('',*,*,#15395,.T.);
#20275=ORIENTED_EDGE('',*,*,#15392,.F.);
#20276=ORIENTED_EDGE('',*,*,#15037,.F.);
#20277=ORIENTED_EDGE('',*,*,#15396,.T.);
#20278=ORIENTED_EDGE('',*,*,#15397,.T.);
#20279=ORIENTED_EDGE('',*,*,#15394,.F.);
#20280=ORIENTED_EDGE('',*,*,#15036,.F.);
#20281=ORIENTED_EDGE('',*,*,#15398,.T.);
#20282=ORIENTED_EDGE('',*,*,#15399,.T.);
#20283=ORIENTED_EDGE('',*,*,#15396,.F.);
#20284=ORIENTED_EDGE('',*,*,#15035,.F.);
#20285=ORIENTED_EDGE('',*,*,#15400,.T.);
#20286=ORIENTED_EDGE('',*,*,#15401,.T.);
#20287=ORIENTED_EDGE('',*,*,#15398,.F.);
#20288=ORIENTED_EDGE('',*,*,#15034,.F.);
#20289=ORIENTED_EDGE('',*,*,#15402,.T.);
#20290=ORIENTED_EDGE('',*,*,#15403,.T.);
#20291=ORIENTED_EDGE('',*,*,#15400,.F.);
#20292=ORIENTED_EDGE('',*,*,#15033,.F.);
#20293=ORIENTED_EDGE('',*,*,#15404,.T.);
#20294=ORIENTED_EDGE('',*,*,#15405,.T.);
#20295=ORIENTED_EDGE('',*,*,#15402,.F.);
#20296=ORIENTED_EDGE('',*,*,#15032,.F.);
#20297=ORIENTED_EDGE('',*,*,#15406,.T.);
#20298=ORIENTED_EDGE('',*,*,#15407,.T.);
#20299=ORIENTED_EDGE('',*,*,#15404,.F.);
#20300=ORIENTED_EDGE('',*,*,#15031,.F.);
#20301=ORIENTED_EDGE('',*,*,#15408,.T.);
#20302=ORIENTED_EDGE('',*,*,#15409,.T.);
#20303=ORIENTED_EDGE('',*,*,#15406,.F.);
#20304=ORIENTED_EDGE('',*,*,#15030,.F.);
#20305=ORIENTED_EDGE('',*,*,#15410,.T.);
#20306=ORIENTED_EDGE('',*,*,#15411,.T.);
#20307=ORIENTED_EDGE('',*,*,#15408,.F.);
#20308=ORIENTED_EDGE('',*,*,#15029,.F.);
#20309=ORIENTED_EDGE('',*,*,#15412,.T.);
#20310=ORIENTED_EDGE('',*,*,#15413,.T.);
#20311=ORIENTED_EDGE('',*,*,#15410,.F.);
#20312=ORIENTED_EDGE('',*,*,#15028,.F.);
#20313=ORIENTED_EDGE('',*,*,#15414,.T.);
#20314=ORIENTED_EDGE('',*,*,#15415,.T.);
#20315=ORIENTED_EDGE('',*,*,#15412,.F.);
#20316=ORIENTED_EDGE('',*,*,#15027,.F.);
#20317=ORIENTED_EDGE('',*,*,#15416,.T.);
#20318=ORIENTED_EDGE('',*,*,#15417,.T.);
#20319=ORIENTED_EDGE('',*,*,#15414,.F.);
#20320=ORIENTED_EDGE('',*,*,#15026,.F.);
#20321=ORIENTED_EDGE('',*,*,#15418,.T.);
#20322=ORIENTED_EDGE('',*,*,#15419,.T.);
#20323=ORIENTED_EDGE('',*,*,#15416,.F.);
#20324=ORIENTED_EDGE('',*,*,#15025,.F.);
#20325=ORIENTED_EDGE('',*,*,#15420,.T.);
#20326=ORIENTED_EDGE('',*,*,#15421,.T.);
#20327=ORIENTED_EDGE('',*,*,#15418,.F.);
#20328=ORIENTED_EDGE('',*,*,#15024,.F.);
#20329=ORIENTED_EDGE('',*,*,#15422,.T.);
#20330=ORIENTED_EDGE('',*,*,#15423,.T.);
#20331=ORIENTED_EDGE('',*,*,#15420,.F.);
#20332=ORIENTED_EDGE('',*,*,#15023,.F.);
#20333=ORIENTED_EDGE('',*,*,#15424,.T.);
#20334=ORIENTED_EDGE('',*,*,#15425,.T.);
#20335=ORIENTED_EDGE('',*,*,#15422,.F.);
#20336=ORIENTED_EDGE('',*,*,#15022,.F.);
#20337=ORIENTED_EDGE('',*,*,#15426,.T.);
#20338=ORIENTED_EDGE('',*,*,#15427,.T.);
#20339=ORIENTED_EDGE('',*,*,#15424,.F.);
#20340=ORIENTED_EDGE('',*,*,#15021,.F.);
#20341=ORIENTED_EDGE('',*,*,#15428,.T.);
#20342=ORIENTED_EDGE('',*,*,#15429,.T.);
#20343=ORIENTED_EDGE('',*,*,#15426,.F.);
#20344=ORIENTED_EDGE('',*,*,#15020,.F.);
#20345=ORIENTED_EDGE('',*,*,#15430,.T.);
#20346=ORIENTED_EDGE('',*,*,#15431,.T.);
#20347=ORIENTED_EDGE('',*,*,#15428,.F.);
#20348=ORIENTED_EDGE('',*,*,#15019,.F.);
#20349=ORIENTED_EDGE('',*,*,#15432,.T.);
#20350=ORIENTED_EDGE('',*,*,#15433,.T.);
#20351=ORIENTED_EDGE('',*,*,#15430,.F.);
#20352=ORIENTED_EDGE('',*,*,#15018,.F.);
#20353=ORIENTED_EDGE('',*,*,#15434,.T.);
#20354=ORIENTED_EDGE('',*,*,#15435,.T.);
#20355=ORIENTED_EDGE('',*,*,#15432,.F.);
#20356=ORIENTED_EDGE('',*,*,#15017,.F.);
#20357=ORIENTED_EDGE('',*,*,#15436,.T.);
#20358=ORIENTED_EDGE('',*,*,#15437,.T.);
#20359=ORIENTED_EDGE('',*,*,#15434,.F.);
#20360=ORIENTED_EDGE('',*,*,#15016,.F.);
#20361=ORIENTED_EDGE('',*,*,#15438,.T.);
#20362=ORIENTED_EDGE('',*,*,#15439,.T.);
#20363=ORIENTED_EDGE('',*,*,#15436,.F.);
#20364=ORIENTED_EDGE('',*,*,#15015,.F.);
#20365=ORIENTED_EDGE('',*,*,#15440,.T.);
#20366=ORIENTED_EDGE('',*,*,#15441,.T.);
#20367=ORIENTED_EDGE('',*,*,#15438,.F.);
#20368=ORIENTED_EDGE('',*,*,#15014,.F.);
#20369=ORIENTED_EDGE('',*,*,#15442,.T.);
#20370=ORIENTED_EDGE('',*,*,#15443,.T.);
#20371=ORIENTED_EDGE('',*,*,#15440,.F.);
#20372=ORIENTED_EDGE('',*,*,#15013,.F.);
#20373=ORIENTED_EDGE('',*,*,#15444,.T.);
#20374=ORIENTED_EDGE('',*,*,#15445,.T.);
#20375=ORIENTED_EDGE('',*,*,#15442,.F.);
#20376=ORIENTED_EDGE('',*,*,#15012,.F.);
#20377=ORIENTED_EDGE('',*,*,#15446,.T.);
#20378=ORIENTED_EDGE('',*,*,#15447,.T.);
#20379=ORIENTED_EDGE('',*,*,#15444,.F.);
#20380=ORIENTED_EDGE('',*,*,#15011,.F.);
#20381=ORIENTED_EDGE('',*,*,#15448,.T.);
#20382=ORIENTED_EDGE('',*,*,#15449,.T.);
#20383=ORIENTED_EDGE('',*,*,#15446,.F.);
#20384=ORIENTED_EDGE('',*,*,#15010,.F.);
#20385=ORIENTED_EDGE('',*,*,#15450,.T.);
#20386=ORIENTED_EDGE('',*,*,#15451,.T.);
#20387=ORIENTED_EDGE('',*,*,#15448,.F.);
#20388=ORIENTED_EDGE('',*,*,#15009,.F.);
#20389=ORIENTED_EDGE('',*,*,#15385,.T.);
#20390=ORIENTED_EDGE('',*,*,#15452,.T.);
#20391=ORIENTED_EDGE('',*,*,#15450,.F.);
#20392=ORIENTED_EDGE('',*,*,#15452,.F.);
#20393=ORIENTED_EDGE('',*,*,#15384,.F.);
#20394=ORIENTED_EDGE('',*,*,#15387,.F.);
#20395=ORIENTED_EDGE('',*,*,#15389,.F.);
#20396=ORIENTED_EDGE('',*,*,#15391,.F.);
#20397=ORIENTED_EDGE('',*,*,#15393,.F.);
#20398=ORIENTED_EDGE('',*,*,#15395,.F.);
#20399=ORIENTED_EDGE('',*,*,#15397,.F.);
#20400=ORIENTED_EDGE('',*,*,#15399,.F.);
#20401=ORIENTED_EDGE('',*,*,#15401,.F.);
#20402=ORIENTED_EDGE('',*,*,#15403,.F.);
#20403=ORIENTED_EDGE('',*,*,#15405,.F.);
#20404=ORIENTED_EDGE('',*,*,#15407,.F.);
#20405=ORIENTED_EDGE('',*,*,#15409,.F.);
#20406=ORIENTED_EDGE('',*,*,#15411,.F.);
#20407=ORIENTED_EDGE('',*,*,#15413,.F.);
#20408=ORIENTED_EDGE('',*,*,#15415,.F.);
#20409=ORIENTED_EDGE('',*,*,#15417,.F.);
#20410=ORIENTED_EDGE('',*,*,#15419,.F.);
#20411=ORIENTED_EDGE('',*,*,#15421,.F.);
#20412=ORIENTED_EDGE('',*,*,#15423,.F.);
#20413=ORIENTED_EDGE('',*,*,#15425,.F.);
#20414=ORIENTED_EDGE('',*,*,#15427,.F.);
#20415=ORIENTED_EDGE('',*,*,#15429,.F.);
#20416=ORIENTED_EDGE('',*,*,#15431,.F.);
#20417=ORIENTED_EDGE('',*,*,#15433,.F.);
#20418=ORIENTED_EDGE('',*,*,#15435,.F.);
#20419=ORIENTED_EDGE('',*,*,#15437,.F.);
#20420=ORIENTED_EDGE('',*,*,#15439,.F.);
#20421=ORIENTED_EDGE('',*,*,#15441,.F.);
#20422=ORIENTED_EDGE('',*,*,#15443,.F.);
#20423=ORIENTED_EDGE('',*,*,#15445,.F.);
#20424=ORIENTED_EDGE('',*,*,#15447,.F.);
#20425=ORIENTED_EDGE('',*,*,#15449,.F.);
#20426=ORIENTED_EDGE('',*,*,#15451,.F.);
#20427=ORIENTED_EDGE('',*,*,#15132,.T.);
#20428=ORIENTED_EDGE('',*,*,#15453,.T.);
#20429=ORIENTED_EDGE('',*,*,#15454,.T.);
#20430=ORIENTED_EDGE('',*,*,#15453,.F.);
#20431=ORIENTED_EDGE('',*,*,#15455,.T.);
#20432=ORIENTED_EDGE('',*,*,#15456,.T.);
#20433=ORIENTED_EDGE('',*,*,#15454,.F.);
#20434=ORIENTED_EDGE('',*,*,#15456,.F.);
#20435=ORIENTED_EDGE('',*,*,#15115,.T.);
#20436=ORIENTED_EDGE('',*,*,#15457,.T.);
#20437=ORIENTED_EDGE('',*,*,#15458,.T.);
#20438=ORIENTED_EDGE('',*,*,#15457,.F.);
#20439=ORIENTED_EDGE('',*,*,#15458,.F.);
#20440=ORIENTED_EDGE('',*,*,#15459,.T.);
#20441=ORIENTED_EDGE('',*,*,#15460,.T.);
#20442=ORIENTED_EDGE('',*,*,#15459,.F.);
#20443=ORIENTED_EDGE('',*,*,#15131,.T.);
#20444=ORIENTED_EDGE('',*,*,#15461,.T.);
#20445=ORIENTED_EDGE('',*,*,#15462,.T.);
#20446=ORIENTED_EDGE('',*,*,#15461,.F.);
#20447=ORIENTED_EDGE('',*,*,#15462,.F.);
#20448=ORIENTED_EDGE('',*,*,#15463,.T.);
#20449=ORIENTED_EDGE('',*,*,#15464,.T.);
#20450=ORIENTED_EDGE('',*,*,#15463,.F.);
#20451=ORIENTED_EDGE('',*,*,#15116,.T.);
#20452=ORIENTED_EDGE('',*,*,#15465,.T.);
#20453=ORIENTED_EDGE('',*,*,#15466,.T.);
#20454=ORIENTED_EDGE('',*,*,#15465,.F.);
#20455=ORIENTED_EDGE('',*,*,#15466,.F.);
#20456=ORIENTED_EDGE('',*,*,#15467,.T.);
#20457=ORIENTED_EDGE('',*,*,#15468,.T.);
#20458=ORIENTED_EDGE('',*,*,#15467,.F.);
#20459=ORIENTED_EDGE('',*,*,#15130,.T.);
#20460=ORIENTED_EDGE('',*,*,#15469,.T.);
#20461=ORIENTED_EDGE('',*,*,#15470,.T.);
#20462=ORIENTED_EDGE('',*,*,#15469,.F.);
#20463=ORIENTED_EDGE('',*,*,#15470,.F.);
#20464=ORIENTED_EDGE('',*,*,#15471,.T.);
#20465=ORIENTED_EDGE('',*,*,#15472,.T.);
#20466=ORIENTED_EDGE('',*,*,#15471,.F.);
#20467=ORIENTED_EDGE('',*,*,#15117,.T.);
#20468=ORIENTED_EDGE('',*,*,#15473,.T.);
#20469=ORIENTED_EDGE('',*,*,#15474,.T.);
#20470=ORIENTED_EDGE('',*,*,#15473,.F.);
#20471=ORIENTED_EDGE('',*,*,#15474,.F.);
#20472=ORIENTED_EDGE('',*,*,#15475,.T.);
#20473=ORIENTED_EDGE('',*,*,#15476,.T.);
#20474=ORIENTED_EDGE('',*,*,#15475,.F.);
#20475=ORIENTED_EDGE('',*,*,#15129,.T.);
#20476=ORIENTED_EDGE('',*,*,#15477,.T.);
#20477=ORIENTED_EDGE('',*,*,#15478,.T.);
#20478=ORIENTED_EDGE('',*,*,#15477,.F.);
#20479=ORIENTED_EDGE('',*,*,#15478,.F.);
#20480=ORIENTED_EDGE('',*,*,#15479,.T.);
#20481=ORIENTED_EDGE('',*,*,#15480,.T.);
#20482=ORIENTED_EDGE('',*,*,#15479,.F.);
#20483=ORIENTED_EDGE('',*,*,#15118,.T.);
#20484=ORIENTED_EDGE('',*,*,#15481,.T.);
#20485=ORIENTED_EDGE('',*,*,#15482,.T.);
#20486=ORIENTED_EDGE('',*,*,#15481,.F.);
#20487=ORIENTED_EDGE('',*,*,#15482,.F.);
#20488=ORIENTED_EDGE('',*,*,#15483,.T.);
#20489=ORIENTED_EDGE('',*,*,#15484,.T.);
#20490=ORIENTED_EDGE('',*,*,#15483,.F.);
#20491=ORIENTED_EDGE('',*,*,#15128,.T.);
#20492=ORIENTED_EDGE('',*,*,#15485,.T.);
#20493=ORIENTED_EDGE('',*,*,#15486,.T.);
#20494=ORIENTED_EDGE('',*,*,#15485,.F.);
#20495=ORIENTED_EDGE('',*,*,#15486,.F.);
#20496=ORIENTED_EDGE('',*,*,#15487,.T.);
#20497=ORIENTED_EDGE('',*,*,#15488,.T.);
#20498=ORIENTED_EDGE('',*,*,#15487,.F.);
#20499=ORIENTED_EDGE('',*,*,#15119,.T.);
#20500=ORIENTED_EDGE('',*,*,#15489,.T.);
#20501=ORIENTED_EDGE('',*,*,#15490,.T.);
#20502=ORIENTED_EDGE('',*,*,#15489,.F.);
#20503=ORIENTED_EDGE('',*,*,#15490,.F.);
#20504=ORIENTED_EDGE('',*,*,#15491,.T.);
#20505=ORIENTED_EDGE('',*,*,#15492,.T.);
#20506=ORIENTED_EDGE('',*,*,#15491,.F.);
#20507=ORIENTED_EDGE('',*,*,#15127,.T.);
#20508=ORIENTED_EDGE('',*,*,#15493,.T.);
#20509=ORIENTED_EDGE('',*,*,#15494,.T.);
#20510=ORIENTED_EDGE('',*,*,#15493,.F.);
#20511=ORIENTED_EDGE('',*,*,#15494,.F.);
#20512=ORIENTED_EDGE('',*,*,#15495,.T.);
#20513=ORIENTED_EDGE('',*,*,#15496,.T.);
#20514=ORIENTED_EDGE('',*,*,#15495,.F.);
#20515=ORIENTED_EDGE('',*,*,#15120,.T.);
#20516=ORIENTED_EDGE('',*,*,#15497,.T.);
#20517=ORIENTED_EDGE('',*,*,#15498,.T.);
#20518=ORIENTED_EDGE('',*,*,#15497,.F.);
#20519=ORIENTED_EDGE('',*,*,#15498,.F.);
#20520=ORIENTED_EDGE('',*,*,#15499,.T.);
#20521=ORIENTED_EDGE('',*,*,#15500,.T.);
#20522=ORIENTED_EDGE('',*,*,#15499,.F.);
#20523=ORIENTED_EDGE('',*,*,#15126,.T.);
#20524=ORIENTED_EDGE('',*,*,#15501,.T.);
#20525=ORIENTED_EDGE('',*,*,#15502,.T.);
#20526=ORIENTED_EDGE('',*,*,#15501,.F.);
#20527=ORIENTED_EDGE('',*,*,#15502,.F.);
#20528=ORIENTED_EDGE('',*,*,#15503,.T.);
#20529=ORIENTED_EDGE('',*,*,#15504,.T.);
#20530=ORIENTED_EDGE('',*,*,#15503,.F.);
#20531=ORIENTED_EDGE('',*,*,#15121,.T.);
#20532=ORIENTED_EDGE('',*,*,#15505,.T.);
#20533=ORIENTED_EDGE('',*,*,#15506,.T.);
#20534=ORIENTED_EDGE('',*,*,#15505,.F.);
#20535=ORIENTED_EDGE('',*,*,#15506,.F.);
#20536=ORIENTED_EDGE('',*,*,#15507,.T.);
#20537=ORIENTED_EDGE('',*,*,#15087,.T.);
#20538=ORIENTED_EDGE('',*,*,#15507,.F.);
#20539=ORIENTED_EDGE('',*,*,#15125,.T.);
#20540=ORIENTED_EDGE('',*,*,#15508,.T.);
#20541=ORIENTED_EDGE('',*,*,#15509,.T.);
#20542=ORIENTED_EDGE('',*,*,#15508,.F.);
#20543=ORIENTED_EDGE('',*,*,#15509,.F.);
#20544=ORIENTED_EDGE('',*,*,#15510,.T.);
#20545=ORIENTED_EDGE('',*,*,#15081,.T.);
#20546=ORIENTED_EDGE('',*,*,#15510,.F.);
#20547=ORIENTED_EDGE('',*,*,#15122,.T.);
#20548=ORIENTED_EDGE('',*,*,#15511,.T.);
#20549=ORIENTED_EDGE('',*,*,#15512,.T.);
#20550=ORIENTED_EDGE('',*,*,#15511,.F.);
#20551=ORIENTED_EDGE('',*,*,#15512,.F.);
#20552=ORIENTED_EDGE('',*,*,#15513,.T.);
#20553=ORIENTED_EDGE('',*,*,#15075,.T.);
#20554=ORIENTED_EDGE('',*,*,#15513,.F.);
#20555=ORIENTED_EDGE('',*,*,#15124,.T.);
#20556=ORIENTED_EDGE('',*,*,#15514,.T.);
#20557=ORIENTED_EDGE('',*,*,#15515,.T.);
#20558=ORIENTED_EDGE('',*,*,#15514,.F.);
#20559=ORIENTED_EDGE('',*,*,#15515,.F.);
#20560=ORIENTED_EDGE('',*,*,#15516,.T.);
#20561=ORIENTED_EDGE('',*,*,#15069,.T.);
#20562=ORIENTED_EDGE('',*,*,#15516,.F.);
#20563=ORIENTED_EDGE('',*,*,#15136,.T.);
#20564=ORIENTED_EDGE('',*,*,#15517,.T.);
#20565=ORIENTED_EDGE('',*,*,#15086,.T.);
#20566=ORIENTED_EDGE('',*,*,#15517,.F.);
#20567=ORIENTED_EDGE('',*,*,#15133,.T.);
#20568=ORIENTED_EDGE('',*,*,#15518,.T.);
#20569=ORIENTED_EDGE('',*,*,#15080,.T.);
#20570=ORIENTED_EDGE('',*,*,#15518,.F.);
#20571=ORIENTED_EDGE('',*,*,#15135,.T.);
#20572=ORIENTED_EDGE('',*,*,#15519,.T.);
#20573=ORIENTED_EDGE('',*,*,#15074,.T.);
#20574=ORIENTED_EDGE('',*,*,#15519,.F.);
#20575=ORIENTED_EDGE('',*,*,#15134,.T.);
#20576=ORIENTED_EDGE('',*,*,#15520,.T.);
#20577=ORIENTED_EDGE('',*,*,#15068,.T.);
#20578=ORIENTED_EDGE('',*,*,#15520,.F.);
#20579=ORIENTED_EDGE('',*,*,#15063,.F.);
#20580=ORIENTED_EDGE('',*,*,#15059,.F.);
#20581=ORIENTED_EDGE('',*,*,#15504,.F.);
#20582=ORIENTED_EDGE('',*,*,#15500,.F.);
#20583=ORIENTED_EDGE('',*,*,#15496,.F.);
#20584=ORIENTED_EDGE('',*,*,#15492,.F.);
#20585=ORIENTED_EDGE('',*,*,#15488,.F.);
#20586=ORIENTED_EDGE('',*,*,#15484,.F.);
#20587=ORIENTED_EDGE('',*,*,#15480,.F.);
#20588=ORIENTED_EDGE('',*,*,#15476,.F.);
#20589=ORIENTED_EDGE('',*,*,#15472,.F.);
#20590=ORIENTED_EDGE('',*,*,#15468,.F.);
#20591=ORIENTED_EDGE('',*,*,#15464,.F.);
#20592=ORIENTED_EDGE('',*,*,#15460,.F.);
#20593=ORIENTED_EDGE('',*,*,#15123,.F.);
#20594=ORIENTED_EDGE('',*,*,#15521,.T.);
#20595=ORIENTED_EDGE('',*,*,#15522,.T.);
#20596=ORIENTED_EDGE('',*,*,#15521,.F.);
#20597=ORIENTED_EDGE('',*,*,#15522,.F.);
#20598=ORIENTED_EDGE('',*,*,#15455,.F.);
#20599=ORIENTED_EDGE('',*,*,#14860,.F.);
#20600=ORIENTED_EDGE('',*,*,#15109,.F.);
#20601=ORIENTED_EDGE('',*,*,#15110,.F.);
#20602=ORIENTED_EDGE('',*,*,#14869,.F.);
#28095=PLANE('',#30892);
#28096=PLANE('',#30893);
#28097=PLANE('',#30894);
#28098=PLANE('',#30895);
#28099=PLANE('',#30896);
#28100=PLANE('',#30897);
#28101=PLANE('',#30898);
#28102=PLANE('',#30899);
#28103=PLANE('',#30900);
#28104=PLANE('',#30901);
#28105=PLANE('',#30905);
#28106=PLANE('',#30918);
#28107=PLANE('',#30925);
#28108=PLANE('',#30932);
#28109=PLANE('',#30939);
#28110=PLANE('',#30941);
#28111=PLANE('',#30942);
#28112=PLANE('',#30943);
#28113=PLANE('',#30944);
#28114=PLANE('',#30945);
#28115=PLANE('',#30946);
#28116=PLANE('',#30947);
#28117=PLANE('',#30948);
#28118=PLANE('',#30949);
#28119=PLANE('',#30950);
#28120=PLANE('',#30951);
#28121=PLANE('',#30952);
#28122=PLANE('',#30953);
#28123=PLANE('',#30954);
#28124=PLANE('',#30955);
#28125=PLANE('',#30973);
#28126=PLANE('',#30974);
#28127=PLANE('',#30980);
#28128=PLANE('',#30981);
#28129=PLANE('',#30982);
#28130=PLANE('',#30983);
#28131=PLANE('',#30984);
#28132=PLANE('',#30985);
#28133=PLANE('',#30986);
#28134=PLANE('',#30987);
#28135=PLANE('',#30988);
#28136=PLANE('',#30989);
#28137=PLANE('',#30990);
#28138=PLANE('',#30991);
#28139=PLANE('',#30992);
#28140=PLANE('',#30993);
#28141=PLANE('',#30994);
#28142=PLANE('',#30995);
#28143=PLANE('',#30996);
#28144=PLANE('',#30997);
#28145=PLANE('',#30998);
#28146=PLANE('',#30999);
#28147=PLANE('',#31000);
#28148=PLANE('',#31001);
#28149=PLANE('',#31002);
#28150=PLANE('',#31003);
#28151=PLANE('',#31004);
#28152=PLANE('',#31005);
#28153=PLANE('',#31006);
#28154=PLANE('',#31007);
#28155=PLANE('',#31008);
#28156=PLANE('',#31009);
#28157=PLANE('',#31010);
#28158=PLANE('',#31011);
#28159=PLANE('',#31012);
#28160=PLANE('',#31013);
#28161=PLANE('',#31014);
#28162=PLANE('',#31015);
#28163=PLANE('',#31016);
#28164=PLANE('',#31017);
#28165=PLANE('',#31018);
#28166=PLANE('',#31019);
#28167=PLANE('',#31020);
#28168=PLANE('',#31021);
#28169=PLANE('',#31022);
#28170=PLANE('',#31023);
#28171=PLANE('',#31024);
#28172=PLANE('',#31025);
#28173=PLANE('',#31026);
#28174=PLANE('',#31027);
#28175=PLANE('',#31028);
#28176=PLANE('',#31029);
#28177=PLANE('',#31030);
#28178=PLANE('',#31031);
#28179=PLANE('',#31032);
#28180=PLANE('',#31033);
#28181=PLANE('',#31034);
#28182=PLANE('',#31035);
#28183=PLANE('',#31104);
#28184=PLANE('',#31105);
#28185=PLANE('',#31106);
#28186=PLANE('',#31107);
#28187=PLANE('',#31108);
#28188=PLANE('',#31109);
#28189=PLANE('',#31110);
#28190=PLANE('',#31111);
#28191=PLANE('',#31112);
#28192=PLANE('',#31113);
#28193=PLANE('',#31114);
#28194=PLANE('',#31115);
#28195=PLANE('',#31116);
#28196=PLANE('',#31117);
#28197=PLANE('',#31120);
#28198=PLANE('',#31121);
#28905=ADVANCED_FACE('',(#3577),#28095,.T.);
#28906=ADVANCED_FACE('',(#3578),#28096,.T.);
#28907=ADVANCED_FACE('',(#3579),#28097,.T.);
#28908=ADVANCED_FACE('',(#3580),#28098,.T.);
#28909=ADVANCED_FACE('',(#3581),#28099,.T.);
#28910=ADVANCED_FACE('',(#3582),#28100,.T.);
#28911=ADVANCED_FACE('',(#3583),#28101,.T.);
#28912=ADVANCED_FACE('',(#3584,#3284,#3285,#3286,#3287,#3288,#3289,#3290,
#3291),#28102,.T.);
#28913=ADVANCED_FACE('',(#3585),#28103,.T.);
#28914=ADVANCED_FACE('',(#3586),#28104,.T.);
#28915=ADVANCED_FACE('',(#3587),#1872,.F.);
#28916=ADVANCED_FACE('',(#3588,#3292,#3293),#28105,.T.);
#28917=ADVANCED_FACE('',(#3589),#433,.F.);
#28918=ADVANCED_FACE('',(#3590),#1873,.F.);
#28919=ADVANCED_FACE('',(#3591),#434,.F.);
#28920=ADVANCED_FACE('',(#3592),#1874,.F.);
#28921=ADVANCED_FACE('',(#3593),#435,.F.);
#28922=ADVANCED_FACE('',(#3594,#3294),#28106,.T.);
#28923=ADVANCED_FACE('',(#3595),#1875,.F.);
#28924=ADVANCED_FACE('',(#3596),#436,.F.);
#28925=ADVANCED_FACE('',(#3597,#3295),#28107,.T.);
#28926=ADVANCED_FACE('',(#3598),#1876,.F.);
#28927=ADVANCED_FACE('',(#3599),#437,.F.);
#28928=ADVANCED_FACE('',(#3600,#3296),#28108,.T.);
#28929=ADVANCED_FACE('',(#3601),#1877,.F.);
#28930=ADVANCED_FACE('',(#3602),#438,.F.);
#28931=ADVANCED_FACE('',(#3603,#3297),#28109,.T.);
#28932=ADVANCED_FACE('',(#3604),#28110,.T.);
#28933=ADVANCED_FACE('',(#3605),#28111,.T.);
#28934=ADVANCED_FACE('',(#3606),#28112,.T.);
#28935=ADVANCED_FACE('',(#3607),#28113,.T.);
#28936=ADVANCED_FACE('',(#3608),#28114,.T.);
#28937=ADVANCED_FACE('',(#3609),#28115,.T.);
#28938=ADVANCED_FACE('',(#3610),#28116,.T.);
#28939=ADVANCED_FACE('',(#3611),#28117,.T.);
#28940=ADVANCED_FACE('',(#3612),#28118,.T.);
#28941=ADVANCED_FACE('',(#3613),#28119,.T.);
#28942=ADVANCED_FACE('',(#3614),#28120,.T.);
#28943=ADVANCED_FACE('',(#3615),#28121,.T.);
#28944=ADVANCED_FACE('',(#3616),#28122,.T.);
#28945=ADVANCED_FACE('',(#3617),#28123,.T.);
#28946=ADVANCED_FACE('',(#3618,#3298,#3299,#3300,#3301,#3302,#3303,#3304,
#3305,#3306,#3307,#3308,#3309,#3310,#3311,#3312,#3313,#3314),#28124,.T.);
#28947=ADVANCED_FACE('',(#3619),#28125,.T.);
#28948=ADVANCED_FACE('',(#3620,#3315,#3316,#3317,#3318,#3319),#28126,.F.);
#28949=ADVANCED_FACE('',(#3621),#28127,.F.);
#28950=ADVANCED_FACE('',(#3622),#28128,.F.);
#28951=ADVANCED_FACE('',(#3623),#28129,.F.);
#28952=ADVANCED_FACE('',(#3624),#28130,.F.);
#28953=ADVANCED_FACE('',(#3625),#28131,.F.);
#28954=ADVANCED_FACE('',(#3626),#28132,.F.);
#28955=ADVANCED_FACE('',(#3627),#28133,.F.);
#28956=ADVANCED_FACE('',(#3628),#28134,.F.);
#28957=ADVANCED_FACE('',(#3629),#28135,.F.);
#28958=ADVANCED_FACE('',(#3630),#28136,.F.);
#28959=ADVANCED_FACE('',(#3631),#28137,.F.);
#28960=ADVANCED_FACE('',(#3632),#28138,.F.);
#28961=ADVANCED_FACE('',(#3633),#28139,.F.);
#28962=ADVANCED_FACE('',(#3634),#28140,.F.);
#28963=ADVANCED_FACE('',(#3635),#308,.F.);
#28964=ADVANCED_FACE('',(#3636),#309,.F.);
#28965=ADVANCED_FACE('',(#3637),#310,.F.);
#28966=ADVANCED_FACE('',(#3638),#311,.F.);
#28967=ADVANCED_FACE('',(#3639),#28141,.F.);
#28968=ADVANCED_FACE('',(#3640),#28142,.F.);
#28969=ADVANCED_FACE('',(#3641),#28143,.F.);
#28970=ADVANCED_FACE('',(#3642),#312,.F.);
#28971=ADVANCED_FACE('',(#3643),#313,.F.);
#28972=ADVANCED_FACE('',(#3644),#314,.F.);
#28973=ADVANCED_FACE('',(#3645),#315,.F.);
#28974=ADVANCED_FACE('',(#3646),#316,.F.);
#28975=ADVANCED_FACE('',(#3647),#317,.F.);
#28976=ADVANCED_FACE('',(#3648),#318,.F.);
#28977=ADVANCED_FACE('',(#3649),#28144,.F.);
#28978=ADVANCED_FACE('',(#3650),#28145,.F.);
#28979=ADVANCED_FACE('',(#3651),#28146,.F.);
#28980=ADVANCED_FACE('',(#3652),#28147,.F.);
#28981=ADVANCED_FACE('',(#3653),#28148,.T.);
#28982=ADVANCED_FACE('',(#3654),#28149,.F.);
#28983=ADVANCED_FACE('',(#3655),#28150,.F.);
#28984=ADVANCED_FACE('',(#3656),#28151,.F.);
#28985=ADVANCED_FACE('',(#3657),#28152,.F.);
#28986=ADVANCED_FACE('',(#3658),#28153,.F.);
#28987=ADVANCED_FACE('',(#3659),#28154,.F.);
#28988=ADVANCED_FACE('',(#3660),#28155,.F.);
#28989=ADVANCED_FACE('',(#3661),#28156,.F.);
#28990=ADVANCED_FACE('',(#3662),#28157,.F.);
#28991=ADVANCED_FACE('',(#3663),#28158,.F.);
#28992=ADVANCED_FACE('',(#3664),#28159,.F.);
#28993=ADVANCED_FACE('',(#3665),#28160,.F.);
#28994=ADVANCED_FACE('',(#3666),#28161,.F.);
#28995=ADVANCED_FACE('',(#3667),#319,.F.);
#28996=ADVANCED_FACE('',(#3668),#320,.F.);
#28997=ADVANCED_FACE('',(#3669),#28162,.F.);
#28998=ADVANCED_FACE('',(#3670),#321,.F.);
#28999=ADVANCED_FACE('',(#3671),#322,.F.);
#29000=ADVANCED_FACE('',(#3672),#323,.F.);
#29001=ADVANCED_FACE('',(#3673),#28163,.F.);
#29002=ADVANCED_FACE('',(#3674),#28164,.F.);
#29003=ADVANCED_FACE('',(#3675),#28165,.F.);
#29004=ADVANCED_FACE('',(#3676),#28166,.F.);
#29005=ADVANCED_FACE('',(#3677),#324,.F.);
#29006=ADVANCED_FACE('',(#3678),#28167,.T.);
#29007=ADVANCED_FACE('',(#3679),#325,.F.);
#29008=ADVANCED_FACE('',(#3680),#326,.F.);
#29009=ADVANCED_FACE('',(#3681),#327,.F.);
#29010=ADVANCED_FACE('',(#3682),#328,.F.);
#29011=ADVANCED_FACE('',(#3683),#329,.F.);
#29012=ADVANCED_FACE('',(#3684),#330,.F.);
#29013=ADVANCED_FACE('',(#3685),#331,.F.);
#29014=ADVANCED_FACE('',(#3686),#332,.F.);
#29015=ADVANCED_FACE('',(#3687),#333,.F.);
#29016=ADVANCED_FACE('',(#3688),#334,.F.);
#29017=ADVANCED_FACE('',(#3689),#335,.F.);
#29018=ADVANCED_FACE('',(#3690),#336,.F.);
#29019=ADVANCED_FACE('',(#3691),#337,.F.);
#29020=ADVANCED_FACE('',(#3692),#28168,.F.);
#29021=ADVANCED_FACE('',(#3693),#338,.F.);
#29022=ADVANCED_FACE('',(#3694),#339,.F.);
#29023=ADVANCED_FACE('',(#3695),#340,.F.);
#29024=ADVANCED_FACE('',(#3696),#341,.F.);
#29025=ADVANCED_FACE('',(#3697),#342,.F.);
#29026=ADVANCED_FACE('',(#3698),#343,.F.);
#29027=ADVANCED_FACE('',(#3699),#344,.F.);
#29028=ADVANCED_FACE('',(#3700),#345,.F.);
#29029=ADVANCED_FACE('',(#3701),#346,.F.);
#29030=ADVANCED_FACE('',(#3702),#347,.F.);
#29031=ADVANCED_FACE('',(#3703),#348,.F.);
#29032=ADVANCED_FACE('',(#3704),#349,.F.);
#29033=ADVANCED_FACE('',(#3705),#350,.F.);
#29034=ADVANCED_FACE('',(#3706),#351,.F.);
#29035=ADVANCED_FACE('',(#3707),#352,.F.);
#29036=ADVANCED_FACE('',(#3708),#353,.F.);
#29037=ADVANCED_FACE('',(#3709),#354,.F.);
#29038=ADVANCED_FACE('',(#3710),#355,.F.);
#29039=ADVANCED_FACE('',(#3711),#28169,.F.);
#29040=ADVANCED_FACE('',(#3712),#356,.F.);
#29041=ADVANCED_FACE('',(#3713),#357,.F.);
#29042=ADVANCED_FACE('',(#3714),#28170,.T.);
#29043=ADVANCED_FACE('',(#3715),#358,.F.);
#29044=ADVANCED_FACE('',(#3716),#359,.F.);
#29045=ADVANCED_FACE('',(#3717),#360,.F.);
#29046=ADVANCED_FACE('',(#3718),#361,.F.);
#29047=ADVANCED_FACE('',(#3719),#362,.F.);
#29048=ADVANCED_FACE('',(#3720),#363,.F.);
#29049=ADVANCED_FACE('',(#3721),#364,.F.);
#29050=ADVANCED_FACE('',(#3722),#365,.F.);
#29051=ADVANCED_FACE('',(#3723),#366,.F.);
#29052=ADVANCED_FACE('',(#3724),#367,.F.);
#29053=ADVANCED_FACE('',(#3725),#368,.F.);
#29054=ADVANCED_FACE('',(#3726),#28171,.F.);
#29055=ADVANCED_FACE('',(#3727),#369,.F.);
#29056=ADVANCED_FACE('',(#3728),#370,.F.);
#29057=ADVANCED_FACE('',(#3729),#371,.F.);
#29058=ADVANCED_FACE('',(#3730),#372,.F.);
#29059=ADVANCED_FACE('',(#3731),#373,.F.);
#29060=ADVANCED_FACE('',(#3732),#374,.F.);
#29061=ADVANCED_FACE('',(#3733),#375,.F.);
#29062=ADVANCED_FACE('',(#3734),#28172,.F.);
#29063=ADVANCED_FACE('',(#3735),#376,.F.);
#29064=ADVANCED_FACE('',(#3736),#377,.F.);
#29065=ADVANCED_FACE('',(#3737),#378,.F.);
#29066=ADVANCED_FACE('',(#3738),#379,.F.);
#29067=ADVANCED_FACE('',(#3739),#380,.F.);
#29068=ADVANCED_FACE('',(#3740),#381,.F.);
#29069=ADVANCED_FACE('',(#3741),#382,.F.);
#29070=ADVANCED_FACE('',(#3742),#28173,.F.);
#29071=ADVANCED_FACE('',(#3743),#383,.F.);
#29072=ADVANCED_FACE('',(#3744),#384,.F.);
#29073=ADVANCED_FACE('',(#3745),#28174,.T.);
#29074=ADVANCED_FACE('',(#3746),#28175,.F.);
#29075=ADVANCED_FACE('',(#3747),#28176,.F.);
#29076=ADVANCED_FACE('',(#3748),#28177,.F.);
#29077=ADVANCED_FACE('',(#3749),#28178,.F.);
#29078=ADVANCED_FACE('',(#3750),#28179,.F.);
#29079=ADVANCED_FACE('',(#3751),#385,.F.);
#29080=ADVANCED_FACE('',(#3752),#386,.F.);
#29081=ADVANCED_FACE('',(#3753),#387,.F.);
#29082=ADVANCED_FACE('',(#3754),#388,.F.);
#29083=ADVANCED_FACE('',(#3755),#389,.F.);
#29084=ADVANCED_FACE('',(#3756),#390,.F.);
#29085=ADVANCED_FACE('',(#3757),#391,.F.);
#29086=ADVANCED_FACE('',(#3758),#392,.F.);
#29087=ADVANCED_FACE('',(#3759),#393,.F.);
#29088=ADVANCED_FACE('',(#3760),#394,.F.);
#29089=ADVANCED_FACE('',(#3761),#395,.F.);
#29090=ADVANCED_FACE('',(#3762),#396,.F.);
#29091=ADVANCED_FACE('',(#3763),#397,.F.);
#29092=ADVANCED_FACE('',(#3764),#28180,.F.);
#29093=ADVANCED_FACE('',(#3765),#398,.F.);
#29094=ADVANCED_FACE('',(#3766),#399,.F.);
#29095=ADVANCED_FACE('',(#3767),#400,.F.);
#29096=ADVANCED_FACE('',(#3768),#401,.F.);
#29097=ADVANCED_FACE('',(#3769),#402,.F.);
#29098=ADVANCED_FACE('',(#3770),#403,.F.);
#29099=ADVANCED_FACE('',(#3771),#404,.F.);
#29100=ADVANCED_FACE('',(#3772),#405,.F.);
#29101=ADVANCED_FACE('',(#3773),#406,.F.);
#29102=ADVANCED_FACE('',(#3774),#407,.F.);
#29103=ADVANCED_FACE('',(#3775),#408,.F.);
#29104=ADVANCED_FACE('',(#3776),#409,.F.);
#29105=ADVANCED_FACE('',(#3777),#410,.F.);
#29106=ADVANCED_FACE('',(#3778),#411,.F.);
#29107=ADVANCED_FACE('',(#3779),#412,.F.);
#29108=ADVANCED_FACE('',(#3780),#413,.F.);
#29109=ADVANCED_FACE('',(#3781),#414,.F.);
#29110=ADVANCED_FACE('',(#3782),#415,.F.);
#29111=ADVANCED_FACE('',(#3783),#28181,.F.);
#29112=ADVANCED_FACE('',(#3784),#416,.F.);
#29113=ADVANCED_FACE('',(#3785),#417,.F.);
#29114=ADVANCED_FACE('',(#3786),#28182,.T.);
#29115=ADVANCED_FACE('',(#3787),#1878,.F.);
#29116=ADVANCED_FACE('',(#3788),#439,.F.);
#29117=ADVANCED_FACE('',(#3789),#1879,.F.);
#29118=ADVANCED_FACE('',(#3790),#440,.F.);
#29119=ADVANCED_FACE('',(#3791),#1880,.F.);
#29120=ADVANCED_FACE('',(#3792),#441,.F.);
#29121=ADVANCED_FACE('',(#3793),#1881,.F.);
#29122=ADVANCED_FACE('',(#3794),#442,.F.);
#29123=ADVANCED_FACE('',(#3795),#1882,.F.);
#29124=ADVANCED_FACE('',(#3796),#443,.F.);
#29125=ADVANCED_FACE('',(#3797),#1883,.F.);
#29126=ADVANCED_FACE('',(#3798),#444,.F.);
#29127=ADVANCED_FACE('',(#3799),#1884,.F.);
#29128=ADVANCED_FACE('',(#3800),#445,.F.);
#29129=ADVANCED_FACE('',(#3801),#1885,.F.);
#29130=ADVANCED_FACE('',(#3802),#446,.F.);
#29131=ADVANCED_FACE('',(#3803),#1886,.F.);
#29132=ADVANCED_FACE('',(#3804),#447,.F.);
#29133=ADVANCED_FACE('',(#3805),#1887,.F.);
#29134=ADVANCED_FACE('',(#3806),#448,.F.);
#29135=ADVANCED_FACE('',(#3807),#1888,.F.);
#29136=ADVANCED_FACE('',(#3808),#449,.F.);
#29137=ADVANCED_FACE('',(#3809),#1889,.F.);
#29138=ADVANCED_FACE('',(#3810),#450,.F.);
#29139=ADVANCED_FACE('',(#3811),#1890,.F.);
#29140=ADVANCED_FACE('',(#3812),#451,.F.);
#29141=ADVANCED_FACE('',(#3813),#1891,.F.);
#29142=ADVANCED_FACE('',(#3814),#452,.F.);
#29143=ADVANCED_FACE('',(#3815),#1892,.F.);
#29144=ADVANCED_FACE('',(#3816),#453,.F.);
#29145=ADVANCED_FACE('',(#3817),#1893,.F.);
#29146=ADVANCED_FACE('',(#3818),#454,.F.);
#29147=ADVANCED_FACE('',(#3819),#1894,.F.);
#29148=ADVANCED_FACE('',(#3820),#455,.F.);
#29149=ADVANCED_FACE('',(#3821),#1895,.F.);
#29150=ADVANCED_FACE('',(#3822),#1896,.F.);
#29151=ADVANCED_FACE('',(#3823),#1897,.F.);
#29152=ADVANCED_FACE('',(#3824),#1898,.F.);
#29153=ADVANCED_FACE('',(#3825),#28183,.F.);
#29154=ADVANCED_FACE('',(#3826),#28184,.F.);
#29155=ADVANCED_FACE('',(#3827),#28185,.T.);
#29156=ADVANCED_FACE('',(#3828),#28186,.T.);
#29157=ADVANCED_FACE('',(#3829),#28187,.T.);
#29158=ADVANCED_FACE('',(#3830),#28188,.T.);
#29159=ADVANCED_FACE('',(#3831),#28189,.T.);
#29160=ADVANCED_FACE('',(#3832),#28190,.T.);
#29161=ADVANCED_FACE('',(#3833),#28191,.T.);
#29162=ADVANCED_FACE('',(#3834),#28192,.T.);
#29163=ADVANCED_FACE('',(#3835),#28193,.T.);
#29164=ADVANCED_FACE('',(#3836),#28194,.T.);
#29165=ADVANCED_FACE('',(#3837),#28195,.T.);
#29166=ADVANCED_FACE('',(#3838),#28196,.T.);
#29167=ADVANCED_FACE('',(#3839),#456,.F.);
#29168=ADVANCED_FACE('',(#3840,#3320),#28197,.T.);
#29169=ADVANCED_FACE('',(#3841),#28198,.T.);
#30661=CLOSED_SHELL('',(#28905,#28906,#28907,#28908,#28909,#28910,#28911,
#28912,#28913,#28914,#28915,#28916,#28917,#28918,#28919,#28920,#28921,#28922,
#28923,#28924,#28925,#28926,#28927,#28928,#28929,#28930,#28931,#28932,#28933,
#28934,#28935,#28936,#28937,#28938,#28939,#28940,#28941,#28942,#28943,#28944,
#28945,#28946,#28947,#28948,#28949,#28950,#28951,#28952,#28953,#28954,#28955,
#28956,#28957,#28958,#28959,#28960,#28961,#28962,#28963,#28964,#28965,#28966,
#28967,#28968,#28969,#28970,#28971,#28972,#28973,#28974,#28975,#28976,#28977,
#28978,#28979,#28980,#28981,#28982,#28983,#28984,#28985,#28986,#28987,#28988,
#28989,#28990,#28991,#28992,#28993,#28994,#28995,#28996,#28997,#28998,#28999,
#29000,#29001,#29002,#29003,#29004,#29005,#29006,#29007,#29008,#29009,#29010,
#29011,#29012,#29013,#29014,#29015,#29016,#29017,#29018,#29019,#29020,#29021,
#29022,#29023,#29024,#29025,#29026,#29027,#29028,#29029,#29030,#29031,#29032,
#29033,#29034,#29035,#29036,#29037,#29038,#29039,#29040,#29041,#29042,#29043,
#29044,#29045,#29046,#29047,#29048,#29049,#29050,#29051,#29052,#29053,#29054,
#29055,#29056,#29057,#29058,#29059,#29060,#29061,#29062,#29063,#29064,#29065,
#29066,#29067,#29068,#29069,#29070,#29071,#29072,#29073,#29074,#29075,#29076,
#29077,#29078,#29079,#29080,#29081,#29082,#29083,#29084,#29085,#29086,#29087,
#29088,#29089,#29090,#29091,#29092,#29093,#29094,#29095,#29096,#29097,#29098,
#29099,#29100,#29101,#29102,#29103,#29104,#29105,#29106,#29107,#29108,#29109,
#29110,#29111,#29112,#29113,#29114,#29115,#29116,#29117,#29118,#29119,#29120,
#29121,#29122,#29123,#29124,#29125,#29126,#29127,#29128,#29129,#29130,#29131,
#29132,#29133,#29134,#29135,#29136,#29137,#29138,#29139,#29140,#29141,#29142,
#29143,#29144,#29145,#29146,#29147,#29148,#29149,#29150,#29151,#29152,#29153,
#29154,#29155,#29156,#29157,#29158,#29159,#29160,#29161,#29162,#29163,#29164,
#29165,#29166,#29167,#29168,#29169));
#30891=AXIS2_PLACEMENT_3D('',#40766,#33415,#33416);
#30892=AXIS2_PLACEMENT_3D('',#40767,#33417,#33418);
#30893=AXIS2_PLACEMENT_3D('',#40780,#33425,#33426);
#30894=AXIS2_PLACEMENT_3D('',#40786,#33430,#33431);
#30895=AXIS2_PLACEMENT_3D('',#40794,#33436,#33437);
#30896=AXIS2_PLACEMENT_3D('',#40800,#33441,#33442);
#30897=AXIS2_PLACEMENT_3D('',#40808,#33447,#33448);
#30898=AXIS2_PLACEMENT_3D('',#40814,#33452,#33453);
#30899=AXIS2_PLACEMENT_3D('',#40822,#33458,#33459);
#30900=AXIS2_PLACEMENT_3D('',#41362,#33510,#33511);
#30901=AXIS2_PLACEMENT_3D('',#41370,#33516,#33517);
#30902=AXIS2_PLACEMENT_3D('',#41376,#33521,#33522);
#30903=AXIS2_PLACEMENT_3D('',#41378,#33523,#33524);
#30904=AXIS2_PLACEMENT_3D('',#41381,#33526,#33527);
#30905=AXIS2_PLACEMENT_3D('',#41382,#33528,#33529);
#30906=AXIS2_PLACEMENT_3D('',#41391,#33534,#33535);
#30907=AXIS2_PLACEMENT_3D('',#41392,#33536,#33537);
#30908=AXIS2_PLACEMENT_3D('',#41395,#33539,#33540);
#30909=AXIS2_PLACEMENT_3D('',#41396,#33541,#33542);
#30910=AXIS2_PLACEMENT_3D('',#41399,#33544,#33545);
#30911=AXIS2_PLACEMENT_3D('',#41400,#33546,#33547);
#30912=AXIS2_PLACEMENT_3D('',#41403,#33549,#33550);
#30913=AXIS2_PLACEMENT_3D('',#41404,#33551,#33552);
#30914=AXIS2_PLACEMENT_3D('',#41406,#33553,#33554);
#30915=AXIS2_PLACEMENT_3D('',#41409,#33556,#33557);
#30916=AXIS2_PLACEMENT_3D('',#41410,#33558,#33559);
#30917=AXIS2_PLACEMENT_3D('',#41413,#33561,#33562);
#30918=AXIS2_PLACEMENT_3D('',#41414,#33563,#33564);
#30919=AXIS2_PLACEMENT_3D('',#41416,#33565,#33566);
#30920=AXIS2_PLACEMENT_3D('',#41417,#33567,#33568);
#30921=AXIS2_PLACEMENT_3D('',#41419,#33569,#33570);
#30922=AXIS2_PLACEMENT_3D('',#41422,#33572,#33573);
#30923=AXIS2_PLACEMENT_3D('',#41423,#33574,#33575);
#30924=AXIS2_PLACEMENT_3D('',#41426,#33577,#33578);
#30925=AXIS2_PLACEMENT_3D('',#41427,#33579,#33580);
#30926=AXIS2_PLACEMENT_3D('',#41429,#33581,#33582);
#30927=AXIS2_PLACEMENT_3D('',#41430,#33583,#33584);
#30928=AXIS2_PLACEMENT_3D('',#41432,#33585,#33586);
#30929=AXIS2_PLACEMENT_3D('',#41435,#33588,#33589);
#30930=AXIS2_PLACEMENT_3D('',#41436,#33590,#33591);
#30931=AXIS2_PLACEMENT_3D('',#41439,#33593,#33594);
#30932=AXIS2_PLACEMENT_3D('',#41440,#33595,#33596);
#30933=AXIS2_PLACEMENT_3D('',#41442,#33597,#33598);
#30934=AXIS2_PLACEMENT_3D('',#41443,#33599,#33600);
#30935=AXIS2_PLACEMENT_3D('',#41445,#33601,#33602);
#30936=AXIS2_PLACEMENT_3D('',#41448,#33604,#33605);
#30937=AXIS2_PLACEMENT_3D('',#41449,#33606,#33607);
#30938=AXIS2_PLACEMENT_3D('',#41452,#33609,#33610);
#30939=AXIS2_PLACEMENT_3D('',#41453,#33611,#33612);
#30940=AXIS2_PLACEMENT_3D('',#41455,#33613,#33614);
#30941=AXIS2_PLACEMENT_3D('',#41456,#33615,#33616);
#30942=AXIS2_PLACEMENT_3D('',#41460,#33619,#33620);
#30943=AXIS2_PLACEMENT_3D('',#41465,#33624,#33625);
#30944=AXIS2_PLACEMENT_3D('',#41469,#33628,#33629);
#30945=AXIS2_PLACEMENT_3D('',#41475,#33633,#33634);
#30946=AXIS2_PLACEMENT_3D('',#41482,#33638,#33639);
#30947=AXIS2_PLACEMENT_3D('',#41488,#33643,#33644);
#30948=AXIS2_PLACEMENT_3D('',#41491,#33647,#33648);
#30949=AXIS2_PLACEMENT_3D('',#41493,#33650,#33651);
#30950=AXIS2_PLACEMENT_3D('',#41495,#33653,#33654);
#30951=AXIS2_PLACEMENT_3D('',#41498,#33657,#33658);
#30952=AXIS2_PLACEMENT_3D('',#41501,#33661,#33662);
#30953=AXIS2_PLACEMENT_3D('',#41503,#33664,#33665);
#30954=AXIS2_PLACEMENT_3D('',#41506,#33668,#33669);
#30955=AXIS2_PLACEMENT_3D('',#41507,#33670,#33671);
#30956=AXIS2_PLACEMENT_3D('',#41509,#33672,#33673);
#30957=AXIS2_PLACEMENT_3D('',#41511,#33674,#33675);
#30958=AXIS2_PLACEMENT_3D('',#41513,#33676,#33677);
#30959=AXIS2_PLACEMENT_3D('',#41515,#33678,#33679);
#30960=AXIS2_PLACEMENT_3D('',#41517,#33680,#33681);
#30961=AXIS2_PLACEMENT_3D('',#41519,#33682,#33683);
#30962=AXIS2_PLACEMENT_3D('',#41521,#33684,#33685);
#30963=AXIS2_PLACEMENT_3D('',#41523,#33686,#33687);
#30964=AXIS2_PLACEMENT_3D('',#41525,#33688,#33689);
#30965=AXIS2_PLACEMENT_3D('',#41527,#33690,#33691);
#30966=AXIS2_PLACEMENT_3D('',#41529,#33692,#33693);
#30967=AXIS2_PLACEMENT_3D('',#41531,#33694,#33695);
#30968=AXIS2_PLACEMENT_3D('',#41533,#33696,#33697);
#30969=AXIS2_PLACEMENT_3D('',#41535,#33698,#33699);
#30970=AXIS2_PLACEMENT_3D('',#41537,#33700,#33701);
#30971=AXIS2_PLACEMENT_3D('',#41539,#33702,#33703);
#30972=AXIS2_PLACEMENT_3D('',#41541,#33704,#33705);
#30973=AXIS2_PLACEMENT_3D('',#41542,#33706,#33707);
#30974=AXIS2_PLACEMENT_3D('',#41543,#33708,#33709);
#30975=AXIS2_PLACEMENT_3D('',#41545,#33710,#33711);
#30976=AXIS2_PLACEMENT_3D('',#41547,#33712,#33713);
#30977=AXIS2_PLACEMENT_3D('',#41549,#33714,#33715);
#30978=AXIS2_PLACEMENT_3D('',#41551,#33716,#33717);
#30979=AXIS2_PLACEMENT_3D('',#41553,#33718,#33719);
#30980=AXIS2_PLACEMENT_3D('',#41554,#33720,#33721);
#30981=AXIS2_PLACEMENT_3D('',#41560,#33725,#33726);
#30982=AXIS2_PLACEMENT_3D('',#41564,#33729,#33730);
#30983=AXIS2_PLACEMENT_3D('',#41568,#33733,#33734);
#30984=AXIS2_PLACEMENT_3D('',#41572,#33737,#33738);
#30985=AXIS2_PLACEMENT_3D('',#41576,#33741,#33742);
#30986=AXIS2_PLACEMENT_3D('',#41580,#33745,#33746);
#30987=AXIS2_PLACEMENT_3D('',#41584,#33749,#33750);
#30988=AXIS2_PLACEMENT_3D('',#41588,#33753,#33754);
#30989=AXIS2_PLACEMENT_3D('',#41592,#33757,#33758);
#30990=AXIS2_PLACEMENT_3D('',#41596,#33761,#33762);
#30991=AXIS2_PLACEMENT_3D('',#41600,#33765,#33766);
#30992=AXIS2_PLACEMENT_3D('',#41602,#33768,#33769);
#30993=AXIS2_PLACEMENT_3D('',#41603,#33770,#33771);
#30994=AXIS2_PLACEMENT_3D('',#41653,#33779,#33780);
#30995=AXIS2_PLACEMENT_3D('',#41657,#33783,#33784);
#30996=AXIS2_PLACEMENT_3D('',#41661,#33787,#33788);
#30997=AXIS2_PLACEMENT_3D('',#41742,#33798,#33799);
#30998=AXIS2_PLACEMENT_3D('',#41746,#33802,#33803);
#30999=AXIS2_PLACEMENT_3D('',#41750,#33806,#33807);
#31000=AXIS2_PLACEMENT_3D('',#41754,#33810,#33811);
#31001=AXIS2_PLACEMENT_3D('',#41756,#33813,#33814);
#31002=AXIS2_PLACEMENT_3D('',#41757,#33815,#33816);
#31003=AXIS2_PLACEMENT_3D('',#41763,#33820,#33821);
#31004=AXIS2_PLACEMENT_3D('',#41767,#33824,#33825);
#31005=AXIS2_PLACEMENT_3D('',#41771,#33828,#33829);
#31006=AXIS2_PLACEMENT_3D('',#41775,#33832,#33833);
#31007=AXIS2_PLACEMENT_3D('',#41779,#33836,#33837);
#31008=AXIS2_PLACEMENT_3D('',#41783,#33840,#33841);
#31009=AXIS2_PLACEMENT_3D('',#41787,#33844,#33845);
#31010=AXIS2_PLACEMENT_3D('',#41791,#33848,#33849);
#31011=AXIS2_PLACEMENT_3D('',#41795,#33852,#33853);
#31012=AXIS2_PLACEMENT_3D('',#41799,#33856,#33857);
#31013=AXIS2_PLACEMENT_3D('',#41803,#33860,#33861);
#31014=AXIS2_PLACEMENT_3D('',#41805,#33863,#33864);
#31015=AXIS2_PLACEMENT_3D('',#41830,#33868,#33869);
#31016=AXIS2_PLACEMENT_3D('',#41867,#33875,#33876);
#31017=AXIS2_PLACEMENT_3D('',#41871,#33879,#33880);
#31018=AXIS2_PLACEMENT_3D('',#41875,#33883,#33884);
#31019=AXIS2_PLACEMENT_3D('',#41879,#33887,#33888);
#31020=AXIS2_PLACEMENT_3D('',#41892,#33891,#33892);
#31021=AXIS2_PLACEMENT_3D('',#42038,#33907,#33908);
#31022=AXIS2_PLACEMENT_3D('',#42240,#33929,#33930);
#31023=AXIS2_PLACEMENT_3D('',#42264,#33934,#33935);
#31024=AXIS2_PLACEMENT_3D('',#42388,#33948,#33949);
#31025=AXIS2_PLACEMENT_3D('',#42469,#33959,#33960);
#31026=AXIS2_PLACEMENT_3D('',#42550,#33970,#33971);
#31027=AXIS2_PLACEMENT_3D('',#42574,#33975,#33976);
#31028=AXIS2_PLACEMENT_3D('',#42575,#33977,#33978);
#31029=AXIS2_PLACEMENT_3D('',#42581,#33982,#33983);
#31030=AXIS2_PLACEMENT_3D('',#42585,#33986,#33987);
#31031=AXIS2_PLACEMENT_3D('',#42589,#33990,#33991);
#31032=AXIS2_PLACEMENT_3D('',#42591,#33993,#33994);
#31033=AXIS2_PLACEMENT_3D('',#42737,#34009,#34010);
#31034=AXIS2_PLACEMENT_3D('',#42939,#34031,#34032);
#31035=AXIS2_PLACEMENT_3D('',#42963,#34036,#34037);
#31036=AXIS2_PLACEMENT_3D('',#42964,#34038,#34039);
#31037=AXIS2_PLACEMENT_3D('',#42967,#34041,#34042);
#31038=AXIS2_PLACEMENT_3D('',#42968,#34043,#34044);
#31039=AXIS2_PLACEMENT_3D('',#42970,#34045,#34046);
#31040=AXIS2_PLACEMENT_3D('',#42972,#34048,#34049);
#31041=AXIS2_PLACEMENT_3D('',#42975,#34051,#34052);
#31042=AXIS2_PLACEMENT_3D('',#42976,#34053,#34054);
#31043=AXIS2_PLACEMENT_3D('',#42979,#34056,#34057);
#31044=AXIS2_PLACEMENT_3D('',#42980,#34058,#34059);
#31045=AXIS2_PLACEMENT_3D('',#42983,#34061,#34062);
#31046=AXIS2_PLACEMENT_3D('',#42984,#34063,#34064);
#31047=AXIS2_PLACEMENT_3D('',#42987,#34066,#34067);
#31048=AXIS2_PLACEMENT_3D('',#42988,#34068,#34069);
#31049=AXIS2_PLACEMENT_3D('',#42991,#34071,#34072);
#31050=AXIS2_PLACEMENT_3D('',#42992,#34073,#34074);
#31051=AXIS2_PLACEMENT_3D('',#42995,#34076,#34077);
#31052=AXIS2_PLACEMENT_3D('',#42996,#34078,#34079);
#31053=AXIS2_PLACEMENT_3D('',#42999,#34081,#34082);
#31054=AXIS2_PLACEMENT_3D('',#43000,#34083,#34084);
#31055=AXIS2_PLACEMENT_3D('',#43003,#34086,#34087);
#31056=AXIS2_PLACEMENT_3D('',#43004,#34088,#34089);
#31057=AXIS2_PLACEMENT_3D('',#43007,#34091,#34092);
#31058=AXIS2_PLACEMENT_3D('',#43008,#34093,#34094);
#31059=AXIS2_PLACEMENT_3D('',#43011,#34096,#34097);
#31060=AXIS2_PLACEMENT_3D('',#43012,#34098,#34099);
#31061=AXIS2_PLACEMENT_3D('',#43015,#34101,#34102);
#31062=AXIS2_PLACEMENT_3D('',#43016,#34103,#34104);
#31063=AXIS2_PLACEMENT_3D('',#43019,#34106,#34107);
#31064=AXIS2_PLACEMENT_3D('',#43020,#34108,#34109);
#31065=AXIS2_PLACEMENT_3D('',#43023,#34111,#34112);
#31066=AXIS2_PLACEMENT_3D('',#43024,#34113,#34114);
#31067=AXIS2_PLACEMENT_3D('',#43027,#34116,#34117);
#31068=AXIS2_PLACEMENT_3D('',#43028,#34118,#34119);
#31069=AXIS2_PLACEMENT_3D('',#43031,#34121,#34122);
#31070=AXIS2_PLACEMENT_3D('',#43032,#34123,#34124);
#31071=AXIS2_PLACEMENT_3D('',#43035,#34126,#34127);
#31072=AXIS2_PLACEMENT_3D('',#43036,#34128,#34129);
#31073=AXIS2_PLACEMENT_3D('',#43039,#34131,#34132);
#31074=AXIS2_PLACEMENT_3D('',#43040,#34133,#34134);
#31075=AXIS2_PLACEMENT_3D('',#43043,#34136,#34137);
#31076=AXIS2_PLACEMENT_3D('',#43044,#34138,#34139);
#31077=AXIS2_PLACEMENT_3D('',#43047,#34141,#34142);
#31078=AXIS2_PLACEMENT_3D('',#43048,#34143,#34144);
#31079=AXIS2_PLACEMENT_3D('',#43051,#34146,#34147);
#31080=AXIS2_PLACEMENT_3D('',#43052,#34148,#34149);
#31081=AXIS2_PLACEMENT_3D('',#43055,#34151,#34152);
#31082=AXIS2_PLACEMENT_3D('',#43056,#34153,#34154);
#31083=AXIS2_PLACEMENT_3D('',#43059,#34156,#34157);
#31084=AXIS2_PLACEMENT_3D('',#43060,#34158,#34159);
#31085=AXIS2_PLACEMENT_3D('',#43063,#34161,#34162);
#31086=AXIS2_PLACEMENT_3D('',#43064,#34163,#34164);
#31087=AXIS2_PLACEMENT_3D('',#43067,#34166,#34167);
#31088=AXIS2_PLACEMENT_3D('',#43068,#34168,#34169);
#31089=AXIS2_PLACEMENT_3D('',#43071,#34171,#34172);
#31090=AXIS2_PLACEMENT_3D('',#43072,#34173,#34174);
#31091=AXIS2_PLACEMENT_3D('',#43074,#34176,#34177);
#31092=AXIS2_PLACEMENT_3D('',#43077,#34179,#34180);
#31093=AXIS2_PLACEMENT_3D('',#43078,#34181,#34182);
#31094=AXIS2_PLACEMENT_3D('',#43080,#34184,#34185);
#31095=AXIS2_PLACEMENT_3D('',#43083,#34187,#34188);
#31096=AXIS2_PLACEMENT_3D('',#43084,#34189,#34190);
#31097=AXIS2_PLACEMENT_3D('',#43086,#34192,#34193);
#31098=AXIS2_PLACEMENT_3D('',#43089,#34195,#34196);
#31099=AXIS2_PLACEMENT_3D('',#43090,#34197,#34198);
#31100=AXIS2_PLACEMENT_3D('',#43092,#34200,#34201);
#31101=AXIS2_PLACEMENT_3D('',#43094,#34203,#34204);
#31102=AXIS2_PLACEMENT_3D('',#43096,#34206,#34207);
#31103=AXIS2_PLACEMENT_3D('',#43098,#34209,#34210);
#31104=AXIS2_PLACEMENT_3D('',#43100,#34212,#34213);
#31105=AXIS2_PLACEMENT_3D('',#43101,#34214,#34215);
#31106=AXIS2_PLACEMENT_3D('',#43102,#34216,#34217);
#31107=AXIS2_PLACEMENT_3D('',#43103,#34218,#34219);
#31108=AXIS2_PLACEMENT_3D('',#43104,#34220,#34221);
#31109=AXIS2_PLACEMENT_3D('',#43105,#34222,#34223);
#31110=AXIS2_PLACEMENT_3D('',#43106,#34224,#34225);
#31111=AXIS2_PLACEMENT_3D('',#43107,#34226,#34227);
#31112=AXIS2_PLACEMENT_3D('',#43108,#34228,#34229);
#31113=AXIS2_PLACEMENT_3D('',#43109,#34230,#34231);
#31114=AXIS2_PLACEMENT_3D('',#43110,#34232,#34233);
#31115=AXIS2_PLACEMENT_3D('',#43111,#34234,#34235);
#31116=AXIS2_PLACEMENT_3D('',#43112,#34236,#34237);
#31117=AXIS2_PLACEMENT_3D('',#43113,#34238,#34239);
#31118=AXIS2_PLACEMENT_3D('',#43114,#34240,#34241);
#31119=AXIS2_PLACEMENT_3D('',#43117,#34243,#34244);
#31120=AXIS2_PLACEMENT_3D('',#43118,#34245,#34246);
#31121=AXIS2_PLACEMENT_3D('',#43119,#34247,#34248);
#33415=DIRECTION('axis',(0.,0.,1.));
#33416=DIRECTION('refdir',(1.,0.,0.));
#33417=DIRECTION('center_axis',(0.707106781186548,0.707106781186548,0.));
#33418=DIRECTION('ref_axis',(0.,0.,-1.));
#33419=DIRECTION('',(0.577350269189628,-0.577350269189628,-0.577350269189621));
#33420=DIRECTION('',(0.,0.,-1.));
#33421=DIRECTION('',(-0.577350269189629,0.577350269189629,-0.57735026918962));
#33422=DIRECTION('',(-0.577350269189629,0.577350269189629,0.57735026918962));
#33423=DIRECTION('',(0.,0.,1.));
#33424=DIRECTION('',(0.577350269189628,-0.577350269189628,0.577350269189621));
#33425=DIRECTION('center_axis',(1.,0.,0.));
#33426=DIRECTION('ref_axis',(0.,1.,0.));
#33427=DIRECTION('',(0.,1.,0.));
#33428=DIRECTION('',(0.,0.,1.));
#33429=DIRECTION('',(0.,-1.,0.));
#33430=DIRECTION('center_axis',(0.707106781186543,0.,0.707106781186552));
#33431=DIRECTION('ref_axis',(0.707106781186552,0.,-0.707106781186543));
#33432=DIRECTION('',(0.577350269189635,0.577350269189615,-0.577350269189628));
#33433=DIRECTION('',(0.,-1.,0.));
#33434=DIRECTION('',(0.577350269189628,-0.577350269189628,-0.577350269189621));
#33435=DIRECTION('',(-0.577350269189628,-0.577350269189628,0.577350269189621));
#33436=DIRECTION('center_axis',(0.,0.707106781186543,0.707106781186552));
#33437=DIRECTION('ref_axis',(1.,0.,0.));
#33438=DIRECTION('',(-1.,0.,0.));
#33439=DIRECTION('',(0.,-0.707106781186552,0.707106781186543));
#33440=DIRECTION('',(1.,0.,0.));
#33441=DIRECTION('center_axis',(0.707106781186548,-0.707106781186548,0.));
#33442=DIRECTION('ref_axis',(0.,0.,-1.));
#33443=DIRECTION('',(-0.577350269189628,-0.577350269189628,-0.577350269189621));
#33444=DIRECTION('',(0.,0.,-1.));
#33445=DIRECTION('',(0.577350269189629,0.577350269189629,-0.57735026918962));
#33446=DIRECTION('',(0.577350269189629,0.577350269189629,0.57735026918962));
#33447=DIRECTION('center_axis',(0.707106781186543,0.,-0.707106781186553));
#33448=DIRECTION('ref_axis',(-0.707106781186553,0.,-0.707106781186543));
#33449=DIRECTION('',(0.577350269189629,-0.577350269189629,0.57735026918962));
#33450=DIRECTION('',(0.,1.,0.));
#33451=DIRECTION('',(0.577350269189629,0.577350269189629,0.57735026918962));
#33452=DIRECTION('center_axis',(0.,-0.707106781186543,-0.707106781186553));
#33453=DIRECTION('ref_axis',(-1.,0.,0.));
#33454=DIRECTION('',(-1.,0.,0.));
#33455=DIRECTION('',(0.577350269189629,-0.577350269189629,0.57735026918962));
#33456=DIRECTION('',(-0.577350269189622,-0.577350269189632,0.577350269189624));
#33457=DIRECTION('',(1.,0.,0.));
#33458=DIRECTION('center_axis',(0.,-1.,0.));
#33459=DIRECTION('ref_axis',(1.,0.,0.));
#33460=DIRECTION('',(1.,0.,0.));
#33461=DIRECTION('',(0.,0.,1.));
#33462=DIRECTION('',(1.,0.,0.));
#33463=DIRECTION('',(0.,0.,-1.));
#33464=DIRECTION('',(-1.,0.,0.));
#33465=DIRECTION('',(0.,0.,1.));
#33466=DIRECTION('',(1.,0.,0.));
#33467=DIRECTION('',(0.,0.,-1.));
#33468=DIRECTION('',(-1.,0.,0.));
#33469=DIRECTION('',(0.,0.,-1.));
#33470=DIRECTION('',(1.,0.,0.));
#33471=DIRECTION('',(0.,0.,-1.));
#33472=DIRECTION('',(-1.,0.,0.));
#33473=DIRECTION('',(0.,0.,-1.));
#33474=DIRECTION('',(-1.,0.,0.));
#33475=DIRECTION('',(0.,0.,-1.));
#33476=DIRECTION('',(-1.,0.,0.));
#33477=DIRECTION('',(0.,0.,1.));
#33478=DIRECTION('',(1.,0.,0.));
#33479=DIRECTION('',(0.538514489852619,0.,-0.842616249676431));
#33480=DIRECTION('',(-1.,0.,0.));
#33481=DIRECTION('',(-0.536696608221845,0.,0.843775296345637));
#33482=DIRECTION('',(1.,0.,0.));
#33483=DIRECTION('',(0.,0.,-1.));
#33484=DIRECTION('',(-1.,0.,0.));
#33485=DIRECTION('',(0.,0.,1.));
#33486=DIRECTION('',(1.,0.,0.));
#33487=DIRECTION('',(0.,0.,-1.));
#33488=DIRECTION('',(-1.,0.,0.));
#33489=DIRECTION('',(0.,0.,-1.));
#33490=DIRECTION('',(1.,0.,0.));
#33491=DIRECTION('',(0.,0.,-1.));
#33492=DIRECTION('',(-1.,0.,0.));
#33493=DIRECTION('',(0.,0.,-1.));
#33494=DIRECTION('',(-1.,0.,0.));
#33495=DIRECTION('',(0.,0.,1.));
#33496=DIRECTION('',(1.,0.,0.));
#33497=DIRECTION('',(0.,0.,-1.));
#33498=DIRECTION('',(-1.,0.,0.));
#33499=DIRECTION('',(0.996199647084823,0.,0.0870991569883124));
#33500=DIRECTION('',(-0.997179320834183,0.,-0.0750559931030013));
#33501=DIRECTION('',(0.991227966055039,0.,0.132163229797056));
#33502=DIRECTION('',(0.125580368698037,0.,0.992083449613824));
#33503=DIRECTION('',(-0.984562438638901,0.,0.175033723668955));
#33504=DIRECTION('',(1.,0.,0.));
#33505=DIRECTION('',(0.,0.,-1.));
#33506=DIRECTION('',(-1.,0.,0.));
#33507=DIRECTION('',(0.,0.,1.));
#33508=DIRECTION('',(0.996199663122956,0.,0.0870989735514131));
#33509=DIRECTION('',(-0.997179320834183,0.,-0.0750559931030013));
#33510=DIRECTION('center_axis',(-0.707106781186548,-0.707106781186548,0.));
#33511=DIRECTION('ref_axis',(0.,0.,1.));
#33512=DIRECTION('',(-0.577350269189625,0.577350269189625,-0.577350269189627));
#33513=DIRECTION('',(0.,0.,-1.));
#33514=DIRECTION('',(0.577350269189625,-0.577350269189625,-0.577350269189627));
#33515=DIRECTION('',(-0.577350269189628,0.577350269189628,0.577350269189621));
#33516=DIRECTION('center_axis',(-0.707106781186549,0.,-0.707106781186546));
#33517=DIRECTION('ref_axis',(-0.707106781186546,0.,0.707106781186549));
#33518=DIRECTION('',(0.,1.,0.));
#33519=DIRECTION('',(0.577350269189625,0.577350269189625,-0.577350269189627));
#33520=DIRECTION('',(0.,-1.,0.));
#33521=DIRECTION('center_axis',(0.,-1.,0.));
#33522=DIRECTION('ref_axis',(1.,0.,0.));
#33523=DIRECTION('center_axis',(0.,-1.,0.));
#33524=DIRECTION('ref_axis',(1.,0.,0.));
#33525=DIRECTION('',(0.707106781186547,0.707106781186547,8.65956056235493E-17));
#33526=DIRECTION('center_axis',(0.,1.,0.));
#33527=DIRECTION('ref_axis',(1.,0.,0.));
#33528=DIRECTION('center_axis',(0.,-1.,0.));
#33529=DIRECTION('ref_axis',(1.,0.,0.));
#33530=DIRECTION('',(1.,0.,0.));
#33531=DIRECTION('',(0.,0.,1.));
#33532=DIRECTION('',(-1.,0.,0.));
#33533=DIRECTION('',(0.,0.,1.));
#33534=DIRECTION('center_axis',(0.,-1.,0.));
#33535=DIRECTION('ref_axis',(1.,0.,0.));
#33536=DIRECTION('center_axis',(0.,1.,0.));
#33537=DIRECTION('ref_axis',(1.,0.,0.));
#33538=DIRECTION('',(0.,1.,0.));
#33539=DIRECTION('center_axis',(0.,1.,0.));
#33540=DIRECTION('ref_axis',(1.,0.,0.));
#33541=DIRECTION('center_axis',(0.,-1.,0.));
#33542=DIRECTION('ref_axis',(1.,0.,0.));
#33543=DIRECTION('',(0.707106781186547,0.707106781186547,8.65956056235493E-17));
#33544=DIRECTION('center_axis',(0.,1.,0.));
#33545=DIRECTION('ref_axis',(1.,0.,0.));
#33546=DIRECTION('center_axis',(0.,1.,0.));
#33547=DIRECTION('ref_axis',(1.,0.,0.));
#33548=DIRECTION('',(0.,1.,0.));
#33549=DIRECTION('center_axis',(0.,1.,0.));
#33550=DIRECTION('ref_axis',(1.,0.,0.));
#33551=DIRECTION('center_axis',(0.,0.,1.));
#33552=DIRECTION('ref_axis',(1.,0.,0.));
#33553=DIRECTION('center_axis',(0.,0.,-1.));
#33554=DIRECTION('ref_axis',(1.,0.,0.));
#33555=DIRECTION('',(-0.707106781186547,8.65956056235493E-17,0.707106781186548));
#33556=DIRECTION('center_axis',(0.,0.,1.));
#33557=DIRECTION('ref_axis',(1.,0.,0.));
#33558=DIRECTION('center_axis',(0.,0.,-1.));
#33559=DIRECTION('ref_axis',(1.,0.,0.));
#33560=DIRECTION('',(0.,0.,-1.));
#33561=DIRECTION('center_axis',(0.,0.,1.));
#33562=DIRECTION('ref_axis',(1.,0.,0.));
#33563=DIRECTION('center_axis',(0.,0.,1.));
#33564=DIRECTION('ref_axis',(1.,0.,0.));
#33565=DIRECTION('center_axis',(0.,0.,-1.));
#33566=DIRECTION('ref_axis',(1.,0.,0.));
#33567=DIRECTION('center_axis',(0.,0.,1.));
#33568=DIRECTION('ref_axis',(1.,0.,0.));
#33569=DIRECTION('center_axis',(0.,0.,-1.));
#33570=DIRECTION('ref_axis',(1.,0.,0.));
#33571=DIRECTION('',(-0.707106781186546,8.65956056235491E-17,0.707106781186549));
#33572=DIRECTION('center_axis',(0.,0.,1.));
#33573=DIRECTION('ref_axis',(1.,0.,0.));
#33574=DIRECTION('center_axis',(0.,0.,-1.));
#33575=DIRECTION('ref_axis',(1.,0.,0.));
#33576=DIRECTION('',(0.,0.,-1.));
#33577=DIRECTION('center_axis',(0.,0.,1.));
#33578=DIRECTION('ref_axis',(1.,0.,0.));
#33579=DIRECTION('center_axis',(0.,0.,1.));
#33580=DIRECTION('ref_axis',(1.,0.,0.));
#33581=DIRECTION('center_axis',(0.,0.,-1.));
#33582=DIRECTION('ref_axis',(1.,0.,0.));
#33583=DIRECTION('center_axis',(0.,0.,1.));
#33584=DIRECTION('ref_axis',(1.,0.,0.));
#33585=DIRECTION('center_axis',(0.,0.,-1.));
#33586=DIRECTION('ref_axis',(1.,0.,0.));
#33587=DIRECTION('',(-0.707106781186546,8.65956056235491E-17,0.707106781186549));
#33588=DIRECTION('center_axis',(0.,0.,1.));
#33589=DIRECTION('ref_axis',(1.,0.,0.));
#33590=DIRECTION('center_axis',(0.,0.,-1.));
#33591=DIRECTION('ref_axis',(1.,0.,0.));
#33592=DIRECTION('',(0.,0.,-1.));
#33593=DIRECTION('center_axis',(0.,0.,1.));
#33594=DIRECTION('ref_axis',(1.,0.,0.));
#33595=DIRECTION('center_axis',(0.,0.,1.));
#33596=DIRECTION('ref_axis',(1.,0.,0.));
#33597=DIRECTION('center_axis',(0.,0.,-1.));
#33598=DIRECTION('ref_axis',(1.,0.,0.));
#33599=DIRECTION('center_axis',(0.,0.,1.));
#33600=DIRECTION('ref_axis',(1.,0.,0.));
#33601=DIRECTION('center_axis',(0.,0.,-1.));
#33602=DIRECTION('ref_axis',(1.,0.,0.));
#33603=DIRECTION('',(-0.707106781186547,8.65956056235493E-17,0.707106781186548));
#33604=DIRECTION('center_axis',(0.,0.,1.));
#33605=DIRECTION('ref_axis',(1.,0.,0.));
#33606=DIRECTION('center_axis',(0.,0.,-1.));
#33607=DIRECTION('ref_axis',(1.,0.,0.));
#33608=DIRECTION('',(0.,0.,-1.));
#33609=DIRECTION('center_axis',(0.,0.,1.));
#33610=DIRECTION('ref_axis',(1.,0.,0.));
#33611=DIRECTION('center_axis',(0.,0.,1.));
#33612=DIRECTION('ref_axis',(1.,0.,0.));
#33613=DIRECTION('center_axis',(0.,0.,-1.));
#33614=DIRECTION('ref_axis',(1.,0.,0.));
#33615=DIRECTION('center_axis',(0.,-0.707106781186543,0.707106781186552));
#33616=DIRECTION('ref_axis',(1.,0.,0.));
#33617=DIRECTION('',(-1.,0.,0.));
#33618=DIRECTION('',(-0.577350269189622,-0.577350269189632,-0.577350269189624));
#33619=DIRECTION('center_axis',(-0.707106781186549,0.,0.707106781186546));
#33620=DIRECTION('ref_axis',(0.707106781186546,0.,0.707106781186549));
#33621=DIRECTION('',(0.,1.,0.));
#33622=DIRECTION('',(-0.577350269189625,-0.577350269189625,-0.577350269189628));
#33623=DIRECTION('',(0.,-1.,0.));
#33624=DIRECTION('center_axis',(-0.577350269189623,0.577350269189623,0.577350269189631));
#33625=DIRECTION('ref_axis',(0.707106781186552,0.,0.707106781186543));
#33626=DIRECTION('',(0.707106781186547,0.707106781186547,0.));
#33627=DIRECTION('',(-0.707106781186552,0.,-0.707106781186543));
#33628=DIRECTION('center_axis',(-0.57735026918962,-0.57735026918963,0.577350269189628));
#33629=DIRECTION('ref_axis',(0.707106781186552,0.,0.707106781186543));
#33630=DIRECTION('',(0.707106781186552,0.,0.707106781186543));
#33631=DIRECTION('',(-0.707106781186554,0.707106781186541,0.));
#33632=DIRECTION('',(0.,-0.707106781186546,-0.707106781186549));
#33633=DIRECTION('center_axis',(-0.577350269189623,0.577350269189623,-0.577350269189631));
#33634=DIRECTION('ref_axis',(-0.707106781186553,0.,0.707106781186543));
#33635=DIRECTION('',(-0.707106781186547,-0.707106781186547,0.));
#33636=DIRECTION('',(0.,0.707106781186552,0.707106781186542));
#33637=DIRECTION('',(0.707106781186552,0.,-0.707106781186542));
#33638=DIRECTION('center_axis',(-0.57735026918962,-0.57735026918963,-0.577350269189628));
#33639=DIRECTION('ref_axis',(-0.707106781186553,0.,0.707106781186543));
#33640=DIRECTION('',(0.707106781186554,-0.707106781186541,0.));
#33641=DIRECTION('',(-0.707106781186552,0.,0.707106781186542));
#33642=DIRECTION('',(0.,0.707106781186546,-0.707106781186549));
#33643=DIRECTION('center_axis',(-0.707106781186543,0.,-0.707106781186553));
#33644=DIRECTION('ref_axis',(-0.707106781186553,0.,0.707106781186543));
#33645=DIRECTION('',(0.,1.,0.));
#33646=DIRECTION('',(0.,-1.,0.));
#33647=DIRECTION('center_axis',(0.,-0.707106781186549,-0.707106781186546));
#33648=DIRECTION('ref_axis',(-1.,0.,0.));
#33649=DIRECTION('',(1.,0.,0.));
#33650=DIRECTION('center_axis',(-0.707106781186541,-0.707106781186554,0.));
#33651=DIRECTION('ref_axis',(0.,0.,1.));
#33652=DIRECTION('',(0.,0.,-1.));
#33653=DIRECTION('center_axis',(0.,0.707106781186543,-0.707106781186553));
#33654=DIRECTION('ref_axis',(-1.,0.,0.));
#33655=DIRECTION('',(-1.,0.,0.));
#33656=DIRECTION('',(1.,0.,0.));
#33657=DIRECTION('center_axis',(-0.707106781186548,0.707106781186548,0.));
#33658=DIRECTION('ref_axis',(0.,0.,1.));
#33659=DIRECTION('',(0.,0.,-1.));
#33660=DIRECTION('',(0.,0.,1.));
#33661=DIRECTION('center_axis',(0.,-0.707106781186549,0.707106781186546));
#33662=DIRECTION('ref_axis',(1.,0.,0.));
#33663=DIRECTION('',(-1.,0.,0.));
#33664=DIRECTION('center_axis',(-0.707106781186543,0.,0.707106781186552));
#33665=DIRECTION('ref_axis',(0.707106781186552,0.,0.707106781186543));
#33666=DIRECTION('',(0.,1.,0.));
#33667=DIRECTION('',(0.,-1.,0.));
#33668=DIRECTION('center_axis',(-1.,0.,0.));
#33669=DIRECTION('ref_axis',(0.,-1.,0.));
#33670=DIRECTION('center_axis',(0.,0.,1.));
#33671=DIRECTION('ref_axis',(1.,0.,0.));
#33672=DIRECTION('center_axis',(0.,0.,1.));
#33673=DIRECTION('ref_axis',(1.,0.,0.));
#33674=DIRECTION('center_axis',(0.,0.,1.));
#33675=DIRECTION('ref_axis',(1.,0.,0.));
#33676=DIRECTION('center_axis',(0.,0.,1.));
#33677=DIRECTION('ref_axis',(1.,0.,0.));
#33678=DIRECTION('center_axis',(0.,0.,1.));
#33679=DIRECTION('ref_axis',(1.,0.,0.));
#33680=DIRECTION('center_axis',(0.,0.,1.));
#33681=DIRECTION('ref_axis',(1.,0.,0.));
#33682=DIRECTION('center_axis',(0.,0.,1.));
#33683=DIRECTION('ref_axis',(1.,0.,0.));
#33684=DIRECTION('center_axis',(0.,0.,1.));
#33685=DIRECTION('ref_axis',(1.,0.,0.));
#33686=DIRECTION('center_axis',(0.,0.,1.));
#33687=DIRECTION('ref_axis',(1.,0.,0.));
#33688=DIRECTION('center_axis',(0.,0.,-1.));
#33689=DIRECTION('ref_axis',(1.,0.,0.));
#33690=DIRECTION('center_axis',(0.,0.,1.));
#33691=DIRECTION('ref_axis',(1.,0.,0.));
#33692=DIRECTION('center_axis',(0.,0.,1.));
#33693=DIRECTION('ref_axis',(1.,0.,0.));
#33694=DIRECTION('center_axis',(0.,0.,1.));
#33695=DIRECTION('ref_axis',(1.,0.,0.));
#33696=DIRECTION('center_axis',(0.,0.,1.));
#33697=DIRECTION('ref_axis',(1.,0.,0.));
#33698=DIRECTION('center_axis',(0.,0.,1.));
#33699=DIRECTION('ref_axis',(1.,0.,0.));
#33700=DIRECTION('center_axis',(0.,0.,1.));
#33701=DIRECTION('ref_axis',(1.,0.,0.));
#33702=DIRECTION('center_axis',(0.,0.,1.));
#33703=DIRECTION('ref_axis',(1.,0.,0.));
#33704=DIRECTION('center_axis',(0.,0.,1.));
#33705=DIRECTION('ref_axis',(1.,0.,0.));
#33706=DIRECTION('center_axis',(-1.,0.,0.));
#33707=DIRECTION('ref_axis',(0.,-1.,0.));
#33708=DIRECTION('center_axis',(0.,0.,1.));
#33709=DIRECTION('ref_axis',(1.,0.,0.));
#33710=DIRECTION('center_axis',(0.,0.,-1.));
#33711=DIRECTION('ref_axis',(1.,0.,0.));
#33712=DIRECTION('center_axis',(0.,0.,-1.));
#33713=DIRECTION('ref_axis',(1.,0.,0.));
#33714=DIRECTION('center_axis',(0.,0.,-1.));
#33715=DIRECTION('ref_axis',(1.,0.,0.));
#33716=DIRECTION('center_axis',(0.,0.,-1.));
#33717=DIRECTION('ref_axis',(1.,0.,0.));
#33718=DIRECTION('center_axis',(0.,0.,-1.));
#33719=DIRECTION('ref_axis',(1.,0.,0.));
#33720=DIRECTION('center_axis',(0.,0.,1.));
#33721=DIRECTION('ref_axis',(1.,0.,0.));
#33722=DIRECTION('',(0.,1.,0.));
#33723=DIRECTION('',(1.,0.,0.));
#33724=DIRECTION('',(0.,1.,0.));
#33725=DIRECTION('center_axis',(1.,0.,0.));
#33726=DIRECTION('ref_axis',(0.,0.,-1.));
#33727=DIRECTION('',(0.,1.,0.));
#33728=DIRECTION('',(0.,0.,-1.));
#33729=DIRECTION('center_axis',(0.,0.,-1.));
#33730=DIRECTION('ref_axis',(-1.,0.,0.));
#33731=DIRECTION('',(0.,1.,0.));
#33732=DIRECTION('',(-1.,0.,0.));
#33733=DIRECTION('center_axis',(1.,0.,0.));
#33734=DIRECTION('ref_axis',(0.,0.,-1.));
#33735=DIRECTION('',(0.,1.,0.));
#33736=DIRECTION('',(0.,0.,-1.));
#33737=DIRECTION('center_axis',(0.,0.,1.));
#33738=DIRECTION('ref_axis',(1.,0.,0.));
#33739=DIRECTION('',(0.,1.,0.));
#33740=DIRECTION('',(1.,0.,0.));
#33741=DIRECTION('center_axis',(1.,0.,0.));
#33742=DIRECTION('ref_axis',(0.,0.,-1.));
#33743=DIRECTION('',(0.,1.,0.));
#33744=DIRECTION('',(0.,0.,-1.));
#33745=DIRECTION('center_axis',(0.,0.,-1.));
#33746=DIRECTION('ref_axis',(-1.,0.,0.));
#33747=DIRECTION('',(0.,1.,0.));
#33748=DIRECTION('',(-1.,0.,0.));
#33749=DIRECTION('center_axis',(1.,0.,0.));
#33750=DIRECTION('ref_axis',(0.,0.,-1.));
#33751=DIRECTION('',(0.,1.,0.));
#33752=DIRECTION('',(0.,0.,-1.));
#33753=DIRECTION('center_axis',(0.,0.,1.));
#33754=DIRECTION('ref_axis',(1.,0.,0.));
#33755=DIRECTION('',(0.,1.,0.));
#33756=DIRECTION('',(1.,0.,0.));
#33757=DIRECTION('center_axis',(-1.,0.,0.));
#33758=DIRECTION('ref_axis',(0.,0.,1.));
#33759=DIRECTION('',(0.,1.,0.));
#33760=DIRECTION('',(0.,0.,1.));
#33761=DIRECTION('center_axis',(0.,0.,-1.));
#33762=DIRECTION('ref_axis',(-1.,0.,0.));
#33763=DIRECTION('',(0.,1.,0.));
#33764=DIRECTION('',(-1.,0.,0.));
#33765=DIRECTION('center_axis',(1.,0.,0.));
#33766=DIRECTION('ref_axis',(0.,0.,-1.));
#33767=DIRECTION('',(0.,0.,-1.));
#33768=DIRECTION('center_axis',(0.,1.,0.));
#33769=DIRECTION('ref_axis',(0.,0.,1.));
#33770=DIRECTION('center_axis',(0.,0.,-1.));
#33771=DIRECTION('ref_axis',(-1.,0.,0.));
#33772=DIRECTION('',(0.,1.,0.));
#33773=DIRECTION('',(-1.,0.,0.));
#33774=DIRECTION('',(0.,1.,0.));
#33775=DIRECTION('',(0.,1.,0.));
#33776=DIRECTION('',(0.,1.,0.));
#33777=DIRECTION('',(0.,1.,0.));
#33778=DIRECTION('',(0.,1.,0.));
#33779=DIRECTION('center_axis',(-0.843775296345637,0.,-0.536696608221845));
#33780=DIRECTION('ref_axis',(-0.536696608221845,0.,0.843775296345637));
#33781=DIRECTION('',(0.,1.,0.));
#33782=DIRECTION('',(-0.536696608221845,0.,0.843775296345637));
#33783=DIRECTION('center_axis',(0.,0.,-1.));
#33784=DIRECTION('ref_axis',(-1.,0.,0.));
#33785=DIRECTION('',(0.,1.,0.));
#33786=DIRECTION('',(-1.,0.,0.));
#33787=DIRECTION('center_axis',(0.842616249676431,0.,0.538514489852619));
#33788=DIRECTION('ref_axis',(0.538514489852619,0.,-0.842616249676431));
#33789=DIRECTION('',(0.,1.,0.));
#33790=DIRECTION('',(0.538514489852619,0.,-0.842616249676431));
#33791=DIRECTION('',(0.,1.,0.));
#33792=DIRECTION('',(0.,1.,0.));
#33793=DIRECTION('',(0.,1.,0.));
#33794=DIRECTION('',(0.,1.,0.));
#33795=DIRECTION('',(0.,1.,0.));
#33796=DIRECTION('',(0.,1.,0.));
#33797=DIRECTION('',(0.,1.,0.));
#33798=DIRECTION('center_axis',(0.,0.,1.));
#33799=DIRECTION('ref_axis',(1.,0.,0.));
#33800=DIRECTION('',(0.,1.,0.));
#33801=DIRECTION('',(1.,0.,0.));
#33802=DIRECTION('center_axis',(-1.,0.,0.));
#33803=DIRECTION('ref_axis',(0.,0.,1.));
#33804=DIRECTION('',(0.,1.,0.));
#33805=DIRECTION('',(0.,0.,1.));
#33806=DIRECTION('center_axis',(0.,0.,-1.));
#33807=DIRECTION('ref_axis',(-1.,0.,0.));
#33808=DIRECTION('',(0.,1.,0.));
#33809=DIRECTION('',(-1.,0.,0.));
#33810=DIRECTION('center_axis',(1.,0.,0.));
#33811=DIRECTION('ref_axis',(0.,0.,-1.));
#33812=DIRECTION('',(0.,0.,-1.));
#33813=DIRECTION('center_axis',(0.,-1.,0.));
#33814=DIRECTION('ref_axis',(1.,0.,0.));
#33815=DIRECTION('center_axis',(0.,0.,1.));
#33816=DIRECTION('ref_axis',(1.,0.,0.));
#33817=DIRECTION('',(0.,1.,0.));
#33818=DIRECTION('',(1.,0.,0.));
#33819=DIRECTION('',(0.,1.,0.));
#33820=DIRECTION('center_axis',(1.,0.,0.));
#33821=DIRECTION('ref_axis',(0.,0.,-1.));
#33822=DIRECTION('',(0.,1.,0.));
#33823=DIRECTION('',(0.,0.,-1.));
#33824=DIRECTION('center_axis',(0.,0.,-1.));
#33825=DIRECTION('ref_axis',(-1.,0.,0.));
#33826=DIRECTION('',(0.,1.,0.));
#33827=DIRECTION('',(-1.,0.,0.));
#33828=DIRECTION('center_axis',(1.,0.,0.));
#33829=DIRECTION('ref_axis',(0.,0.,-1.));
#33830=DIRECTION('',(0.,1.,0.));
#33831=DIRECTION('',(0.,0.,-1.));
#33832=DIRECTION('center_axis',(0.,0.,1.));
#33833=DIRECTION('ref_axis',(1.,0.,0.));
#33834=DIRECTION('',(0.,1.,0.));
#33835=DIRECTION('',(1.,0.,0.));
#33836=DIRECTION('center_axis',(1.,0.,0.));
#33837=DIRECTION('ref_axis',(0.,0.,-1.));
#33838=DIRECTION('',(0.,1.,0.));
#33839=DIRECTION('',(0.,0.,-1.));
#33840=DIRECTION('center_axis',(0.,0.,-1.));
#33841=DIRECTION('ref_axis',(-1.,0.,0.));
#33842=DIRECTION('',(0.,1.,0.));
#33843=DIRECTION('',(-1.,0.,0.));
#33844=DIRECTION('center_axis',(1.,0.,0.));
#33845=DIRECTION('ref_axis',(0.,0.,-1.));
#33846=DIRECTION('',(0.,1.,0.));
#33847=DIRECTION('',(0.,0.,-1.));
#33848=DIRECTION('center_axis',(0.,0.,1.));
#33849=DIRECTION('ref_axis',(1.,0.,0.));
#33850=DIRECTION('',(0.,1.,0.));
#33851=DIRECTION('',(1.,0.,0.));
#33852=DIRECTION('center_axis',(-1.,0.,0.));
#33853=DIRECTION('ref_axis',(0.,0.,1.));
#33854=DIRECTION('',(0.,1.,0.));
#33855=DIRECTION('',(0.,0.,1.));
#33856=DIRECTION('center_axis',(0.,0.,-1.));
#33857=DIRECTION('ref_axis',(-1.,0.,0.));
#33858=DIRECTION('',(0.,1.,0.));
#33859=DIRECTION('',(-1.,0.,0.));
#33860=DIRECTION('center_axis',(1.,0.,0.));
#33861=DIRECTION('ref_axis',(0.,0.,-1.));
#33862=DIRECTION('',(0.,0.,-1.));
#33863=DIRECTION('center_axis',(0.,1.,0.));
#33864=DIRECTION('ref_axis',(0.,0.,1.));
#33865=DIRECTION('',(0.,1.,0.));
#33866=DIRECTION('',(0.,1.,0.));
#33867=DIRECTION('',(0.,1.,0.));
#33868=DIRECTION('center_axis',(0.,0.,-1.));
#33869=DIRECTION('ref_axis',(-1.,0.,0.));
#33870=DIRECTION('',(0.,1.,0.));
#33871=DIRECTION('',(-1.,0.,0.));
#33872=DIRECTION('',(0.,1.,0.));
#33873=DIRECTION('',(0.,1.,0.));
#33874=DIRECTION('',(0.,1.,0.));
#33875=DIRECTION('center_axis',(1.,0.,0.));
#33876=DIRECTION('ref_axis',(0.,0.,-1.));
#33877=DIRECTION('',(0.,1.,0.));
#33878=DIRECTION('',(0.,0.,-1.));
#33879=DIRECTION('center_axis',(0.,0.,1.));
#33880=DIRECTION('ref_axis',(1.,0.,0.));
#33881=DIRECTION('',(0.,1.,0.));
#33882=DIRECTION('',(1.,0.,0.));
#33883=DIRECTION('center_axis',(-1.,0.,0.));
#33884=DIRECTION('ref_axis',(0.,0.,1.));
#33885=DIRECTION('',(0.,1.,0.));
#33886=DIRECTION('',(0.,0.,1.));
#33887=DIRECTION('center_axis',(0.,0.,-1.));
#33888=DIRECTION('ref_axis',(-1.,0.,0.));
#33889=DIRECTION('',(0.,1.,0.));
#33890=DIRECTION('',(-1.,0.,0.));
#33891=DIRECTION('center_axis',(0.,-1.,0.));
#33892=DIRECTION('ref_axis',(1.,0.,0.));
#33893=DIRECTION('',(0.,1.,0.));
#33894=DIRECTION('',(0.,1.,0.));
#33895=DIRECTION('',(0.,1.,0.));
#33896=DIRECTION('',(0.,1.,0.));
#33897=DIRECTION('',(0.,1.,0.));
#33898=DIRECTION('',(0.,1.,0.));
#33899=DIRECTION('',(0.,1.,0.));
#33900=DIRECTION('',(0.,1.,0.));
#33901=DIRECTION('',(0.,1.,0.));
#33902=DIRECTION('',(0.,1.,0.));
#33903=DIRECTION('',(0.,1.,0.));
#33904=DIRECTION('',(0.,1.,0.));
#33905=DIRECTION('',(0.,1.,0.));
#33906=DIRECTION('',(0.,1.,0.));
#33907=DIRECTION('center_axis',(0.0750559931030013,0.,-0.997179320834183));
#33908=DIRECTION('ref_axis',(-0.997179320834183,0.,-0.0750559931030013));
#33909=DIRECTION('',(0.,1.,0.));
#33910=DIRECTION('',(-0.997179320834183,0.,-0.0750559931030013));
#33911=DIRECTION('',(0.,1.,0.));
#33912=DIRECTION('',(0.,1.,0.));
#33913=DIRECTION('',(0.,1.,0.));
#33914=DIRECTION('',(0.,1.,0.));
#33915=DIRECTION('',(0.,1.,0.));
#33916=DIRECTION('',(0.,1.,0.));
#33917=DIRECTION('',(0.,1.,0.));
#33918=DIRECTION('',(0.,1.,0.));
#33919=DIRECTION('',(0.,1.,0.));
#33920=DIRECTION('',(0.,1.,0.));
#33921=DIRECTION('',(0.,1.,0.));
#33922=DIRECTION('',(0.,1.,0.));
#33923=DIRECTION('',(0.,1.,0.));
#33924=DIRECTION('',(0.,1.,0.));
#33925=DIRECTION('',(0.,1.,0.));
#33926=DIRECTION('',(0.,1.,0.));
#33927=DIRECTION('',(0.,1.,0.));
#33928=DIRECTION('',(0.,1.,0.));
#33929=DIRECTION('center_axis',(-0.0870991569883124,0.,0.996199647084823));
#33930=DIRECTION('ref_axis',(0.996199647084823,0.,0.0870991569883124));
#33931=DIRECTION('',(0.,1.,0.));
#33932=DIRECTION('',(0.996199647084823,0.,0.0870991569883124));
#33933=DIRECTION('',(0.,1.,0.));
#33934=DIRECTION('center_axis',(0.,-1.,0.));
#33935=DIRECTION('ref_axis',(1.,0.,0.));
#33936=DIRECTION('',(0.,1.,0.));
#33937=DIRECTION('',(0.,1.,0.));
#33938=DIRECTION('',(0.,1.,0.));
#33939=DIRECTION('',(0.,1.,0.));
#33940=DIRECTION('',(0.,1.,0.));
#33941=DIRECTION('',(0.,1.,0.));
#33942=DIRECTION('',(0.,1.,0.));
#33943=DIRECTION('',(0.,1.,0.));
#33944=DIRECTION('',(0.,1.,0.));
#33945=DIRECTION('',(0.,1.,0.));
#33946=DIRECTION('',(0.,1.,0.));
#33947=DIRECTION('',(0.,1.,0.));
#33948=DIRECTION('center_axis',(-0.175033723668955,0.,-0.984562438638901));
#33949=DIRECTION('ref_axis',(-0.984562438638901,0.,0.175033723668955));
#33950=DIRECTION('',(0.,1.,0.));
#33951=DIRECTION('',(-0.984562438638901,0.,0.175033723668955));
#33952=DIRECTION('',(0.,1.,0.));
#33953=DIRECTION('',(0.,1.,0.));
#33954=DIRECTION('',(0.,1.,0.));
#33955=DIRECTION('',(0.,1.,0.));
#33956=DIRECTION('',(0.,1.,0.));
#33957=DIRECTION('',(0.,1.,0.));
#33958=DIRECTION('',(0.,1.,0.));
#33959=DIRECTION('center_axis',(-0.992083449613824,0.,0.125580368698037));
#33960=DIRECTION('ref_axis',(0.125580368698037,0.,0.992083449613824));
#33961=DIRECTION('',(0.,1.,0.));
#33962=DIRECTION('',(0.125580368698037,0.,0.992083449613824));
#33963=DIRECTION('',(0.,1.,0.));
#33964=DIRECTION('',(0.,1.,0.));
#33965=DIRECTION('',(0.,1.,0.));
#33966=DIRECTION('',(0.,1.,0.));
#33967=DIRECTION('',(0.,1.,0.));
#33968=DIRECTION('',(0.,1.,0.));
#33969=DIRECTION('',(0.,1.,0.));
#33970=DIRECTION('center_axis',(-0.132163229797056,0.,0.99122796605504));
#33971=DIRECTION('ref_axis',(0.991227966055039,0.,0.132163229797056));
#33972=DIRECTION('',(0.,1.,0.));
#33973=DIRECTION('',(0.991227966055039,0.,0.132163229797056));
#33974=DIRECTION('',(0.,1.,0.));
#33975=DIRECTION('center_axis',(0.,-1.,0.));
#33976=DIRECTION('ref_axis',(1.,0.,0.));
#33977=DIRECTION('center_axis',(0.,0.,1.));
#33978=DIRECTION('ref_axis',(1.,0.,0.));
#33979=DIRECTION('',(0.,1.,0.));
#33980=DIRECTION('',(1.,0.,0.));
#33981=DIRECTION('',(0.,1.,0.));
#33982=DIRECTION('center_axis',(-1.,0.,0.));
#33983=DIRECTION('ref_axis',(0.,0.,1.));
#33984=DIRECTION('',(0.,1.,0.));
#33985=DIRECTION('',(0.,0.,1.));
#33986=DIRECTION('center_axis',(0.,0.,-1.));
#33987=DIRECTION('ref_axis',(-1.,0.,0.));
#33988=DIRECTION('',(0.,1.,0.));
#33989=DIRECTION('',(-1.,0.,0.));
#33990=DIRECTION('center_axis',(1.,0.,0.));
#33991=DIRECTION('ref_axis',(0.,0.,-1.));
#33992=DIRECTION('',(0.,0.,-1.));
#33993=DIRECTION('center_axis',(0.,1.,0.));
#33994=DIRECTION('ref_axis',(0.,0.,1.));
#33995=DIRECTION('',(0.,1.,0.));
#33996=DIRECTION('',(0.,1.,0.));
#33997=DIRECTION('',(0.,1.,0.));
#33998=DIRECTION('',(0.,1.,0.));
#33999=DIRECTION('',(0.,1.,0.));
#34000=DIRECTION('',(0.,1.,0.));
#34001=DIRECTION('',(0.,1.,0.));
#34002=DIRECTION('',(0.,1.,0.));
#34003=DIRECTION('',(0.,1.,0.));
#34004=DIRECTION('',(0.,1.,0.));
#34005=DIRECTION('',(0.,1.,0.));
#34006=DIRECTION('',(0.,1.,0.));
#34007=DIRECTION('',(0.,1.,0.));
#34008=DIRECTION('',(0.,1.,0.));
#34009=DIRECTION('center_axis',(0.0750559931030013,0.,-0.997179320834183));
#34010=DIRECTION('ref_axis',(-0.997179320834183,0.,-0.0750559931030013));
#34011=DIRECTION('',(0.,1.,0.));
#34012=DIRECTION('',(-0.997179320834183,0.,-0.0750559931030013));
#34013=DIRECTION('',(0.,1.,0.));
#34014=DIRECTION('',(0.,1.,0.));
#34015=DIRECTION('',(0.,1.,0.));
#34016=DIRECTION('',(0.,1.,0.));
#34017=DIRECTION('',(0.,1.,0.));
#34018=DIRECTION('',(0.,1.,0.));
#34019=DIRECTION('',(0.,1.,0.));
#34020=DIRECTION('',(0.,1.,0.));
#34021=DIRECTION('',(0.,1.,0.));
#34022=DIRECTION('',(0.,1.,0.));
#34023=DIRECTION('',(0.,1.,0.));
#34024=DIRECTION('',(0.,1.,0.));
#34025=DIRECTION('',(0.,1.,0.));
#34026=DIRECTION('',(0.,1.,0.));
#34027=DIRECTION('',(0.,1.,0.));
#34028=DIRECTION('',(0.,1.,0.));
#34029=DIRECTION('',(0.,1.,0.));
#34030=DIRECTION('',(0.,1.,0.));
#34031=DIRECTION('center_axis',(-0.0870989735514131,0.,0.996199663122956));
#34032=DIRECTION('ref_axis',(0.996199663122956,0.,0.0870989735514131));
#34033=DIRECTION('',(0.,1.,0.));
#34034=DIRECTION('',(0.996199663122956,0.,0.0870989735514131));
#34035=DIRECTION('',(0.,1.,0.));
#34036=DIRECTION('center_axis',(0.,-1.,0.));
#34037=DIRECTION('ref_axis',(1.,0.,0.));
#34038=DIRECTION('center_axis',(0.,0.,-1.));
#34039=DIRECTION('ref_axis',(1.,0.,0.));
#34040=DIRECTION('',(0.707106781186547,-8.65956056235493E-17,0.707106781186548));
#34041=DIRECTION('center_axis',(0.,0.,1.));
#34042=DIRECTION('ref_axis',(1.,0.,0.));
#34043=DIRECTION('center_axis',(0.,0.,-1.));
#34044=DIRECTION('ref_axis',(1.,0.,0.));
#34045=DIRECTION('center_axis',(0.,0.,1.));
#34046=DIRECTION('ref_axis',(1.,0.,0.));
#34047=DIRECTION('',(0.,0.,-1.));
#34048=DIRECTION('center_axis',(0.,0.,1.));
#34049=DIRECTION('ref_axis',(1.,0.,0.));
#34050=DIRECTION('',(0.707106781186548,8.65956056235493E-17,-0.707106781186548));
#34051=DIRECTION('center_axis',(0.,0.,-1.));
#34052=DIRECTION('ref_axis',(1.,0.,0.));
#34053=DIRECTION('center_axis',(0.,0.,-1.));
#34054=DIRECTION('ref_axis',(1.,0.,0.));
#34055=DIRECTION('',(0.,0.,-1.));
#34056=DIRECTION('center_axis',(0.,0.,-1.));
#34057=DIRECTION('ref_axis',(1.,0.,0.));
#34058=DIRECTION('center_axis',(0.,0.,1.));
#34059=DIRECTION('ref_axis',(1.,0.,0.));
#34060=DIRECTION('',(0.707106781186548,8.65956056235493E-17,-0.707106781186548));
#34061=DIRECTION('center_axis',(0.,0.,-1.));
#34062=DIRECTION('ref_axis',(1.,0.,0.));
#34063=DIRECTION('center_axis',(0.,0.,-1.));
#34064=DIRECTION('ref_axis',(1.,0.,0.));
#34065=DIRECTION('',(0.,0.,-1.));
#34066=DIRECTION('center_axis',(0.,0.,-1.));
#34067=DIRECTION('ref_axis',(1.,0.,0.));
#34068=DIRECTION('center_axis',(0.,0.,1.));
#34069=DIRECTION('ref_axis',(1.,0.,0.));
#34070=DIRECTION('',(0.707106781186548,8.65956056235493E-17,-0.707106781186548));
#34071=DIRECTION('center_axis',(0.,0.,-1.));
#34072=DIRECTION('ref_axis',(1.,0.,0.));
#34073=DIRECTION('center_axis',(0.,0.,-1.));
#34074=DIRECTION('ref_axis',(1.,0.,0.));
#34075=DIRECTION('',(0.,0.,-1.));
#34076=DIRECTION('center_axis',(0.,0.,-1.));
#34077=DIRECTION('ref_axis',(1.,0.,0.));
#34078=DIRECTION('center_axis',(0.,0.,1.));
#34079=DIRECTION('ref_axis',(1.,0.,0.));
#34080=DIRECTION('',(0.70710678118654,8.65956056235484E-17,-0.707106781186555));
#34081=DIRECTION('center_axis',(0.,0.,-1.));
#34082=DIRECTION('ref_axis',(1.,0.,0.));
#34083=DIRECTION('center_axis',(0.,0.,-1.));
#34084=DIRECTION('ref_axis',(1.,0.,0.));
#34085=DIRECTION('',(0.,0.,-1.));
#34086=DIRECTION('center_axis',(0.,0.,-1.));
#34087=DIRECTION('ref_axis',(1.,0.,0.));
#34088=DIRECTION('center_axis',(0.,0.,1.));
#34089=DIRECTION('ref_axis',(1.,0.,0.));
#34090=DIRECTION('',(0.707106781186547,8.65956056235493E-17,-0.707106781186547));
#34091=DIRECTION('center_axis',(0.,0.,-1.));
#34092=DIRECTION('ref_axis',(1.,0.,0.));
#34093=DIRECTION('center_axis',(0.,0.,-1.));
#34094=DIRECTION('ref_axis',(1.,0.,0.));
#34095=DIRECTION('',(0.,0.,-1.));
#34096=DIRECTION('center_axis',(0.,0.,-1.));
#34097=DIRECTION('ref_axis',(1.,0.,0.));
#34098=DIRECTION('center_axis',(0.,0.,1.));
#34099=DIRECTION('ref_axis',(1.,0.,0.));
#34100=DIRECTION('',(0.70710678118654,8.65956056235484E-17,-0.707106781186555));
#34101=DIRECTION('center_axis',(0.,0.,-1.));
#34102=DIRECTION('ref_axis',(1.,0.,0.));
#34103=DIRECTION('center_axis',(0.,0.,-1.));
#34104=DIRECTION('ref_axis',(1.,0.,0.));
#34105=DIRECTION('',(0.,0.,-1.));
#34106=DIRECTION('center_axis',(0.,0.,-1.));
#34107=DIRECTION('ref_axis',(1.,0.,0.));
#34108=DIRECTION('center_axis',(0.,0.,1.));
#34109=DIRECTION('ref_axis',(1.,0.,0.));
#34110=DIRECTION('',(0.707106781186548,8.65956056235493E-17,-0.707106781186548));
#34111=DIRECTION('center_axis',(0.,0.,-1.));
#34112=DIRECTION('ref_axis',(1.,0.,0.));
#34113=DIRECTION('center_axis',(0.,0.,-1.));
#34114=DIRECTION('ref_axis',(1.,0.,0.));
#34115=DIRECTION('',(0.,0.,-1.));
#34116=DIRECTION('center_axis',(0.,0.,-1.));
#34117=DIRECTION('ref_axis',(1.,0.,0.));
#34118=DIRECTION('center_axis',(0.,0.,1.));
#34119=DIRECTION('ref_axis',(1.,0.,0.));
#34120=DIRECTION('',(0.707106781186548,8.65956056235493E-17,-0.707106781186548));
#34121=DIRECTION('center_axis',(0.,0.,-1.));
#34122=DIRECTION('ref_axis',(1.,0.,0.));
#34123=DIRECTION('center_axis',(0.,0.,-1.));
#34124=DIRECTION('ref_axis',(1.,0.,0.));
#34125=DIRECTION('',(0.,0.,-1.));
#34126=DIRECTION('center_axis',(0.,0.,-1.));
#34127=DIRECTION('ref_axis',(1.,0.,0.));
#34128=DIRECTION('center_axis',(0.,0.,1.));
#34129=DIRECTION('ref_axis',(1.,0.,0.));
#34130=DIRECTION('',(0.70710678118654,8.65956056235484E-17,-0.707106781186555));
#34131=DIRECTION('center_axis',(0.,0.,-1.));
#34132=DIRECTION('ref_axis',(1.,0.,0.));
#34133=DIRECTION('center_axis',(0.,0.,-1.));
#34134=DIRECTION('ref_axis',(1.,0.,0.));
#34135=DIRECTION('',(0.,0.,-1.));
#34136=DIRECTION('center_axis',(0.,0.,-1.));
#34137=DIRECTION('ref_axis',(1.,0.,0.));
#34138=DIRECTION('center_axis',(0.,0.,1.));
#34139=DIRECTION('ref_axis',(1.,0.,0.));
#34140=DIRECTION('',(0.707106781186548,8.65956056235493E-17,-0.707106781186548));
#34141=DIRECTION('center_axis',(0.,0.,-1.));
#34142=DIRECTION('ref_axis',(1.,0.,0.));
#34143=DIRECTION('center_axis',(0.,0.,-1.));
#34144=DIRECTION('ref_axis',(1.,0.,0.));
#34145=DIRECTION('',(0.,0.,-1.));
#34146=DIRECTION('center_axis',(0.,0.,-1.));
#34147=DIRECTION('ref_axis',(1.,0.,0.));
#34148=DIRECTION('center_axis',(0.,0.,1.));
#34149=DIRECTION('ref_axis',(1.,0.,0.));
#34150=DIRECTION('',(0.70710678118654,8.65956056235484E-17,-0.707106781186555));
#34151=DIRECTION('center_axis',(0.,0.,-1.));
#34152=DIRECTION('ref_axis',(1.,0.,0.));
#34153=DIRECTION('center_axis',(0.,0.,-1.));
#34154=DIRECTION('ref_axis',(1.,0.,0.));
#34155=DIRECTION('',(0.,0.,-1.));
#34156=DIRECTION('center_axis',(0.,0.,-1.));
#34157=DIRECTION('ref_axis',(1.,0.,0.));
#34158=DIRECTION('center_axis',(0.,0.,1.));
#34159=DIRECTION('ref_axis',(1.,0.,0.));
#34160=DIRECTION('',(0.707106781186548,8.65956056235493E-17,-0.707106781186548));
#34161=DIRECTION('center_axis',(0.,0.,-1.));
#34162=DIRECTION('ref_axis',(1.,0.,0.));
#34163=DIRECTION('center_axis',(0.,0.,-1.));
#34164=DIRECTION('ref_axis',(1.,0.,0.));
#34165=DIRECTION('',(0.,0.,-1.));
#34166=DIRECTION('center_axis',(0.,0.,-1.));
#34167=DIRECTION('ref_axis',(1.,0.,0.));
#34168=DIRECTION('center_axis',(0.,0.,1.));
#34169=DIRECTION('ref_axis',(1.,0.,0.));
#34170=DIRECTION('',(0.707106781186547,8.65956056235493E-17,-0.707106781186547));
#34171=DIRECTION('center_axis',(0.,0.,-1.));
#34172=DIRECTION('ref_axis',(1.,0.,0.));
#34173=DIRECTION('center_axis',(0.,0.,-1.));
#34174=DIRECTION('ref_axis',(1.,0.,0.));
#34175=DIRECTION('',(0.,0.,-1.));
#34176=DIRECTION('center_axis',(0.,0.,1.));
#34177=DIRECTION('ref_axis',(1.,0.,0.));
#34178=DIRECTION('',(0.707106781186548,8.65956056235493E-17,-0.707106781186548));
#34179=DIRECTION('center_axis',(0.,0.,-1.));
#34180=DIRECTION('ref_axis',(1.,0.,0.));
#34181=DIRECTION('center_axis',(0.,0.,-1.));
#34182=DIRECTION('ref_axis',(1.,0.,0.));
#34183=DIRECTION('',(0.,0.,-1.));
#34184=DIRECTION('center_axis',(0.,0.,1.));
#34185=DIRECTION('ref_axis',(1.,0.,0.));
#34186=DIRECTION('',(0.707106781186548,8.65956056235493E-17,-0.707106781186548));
#34187=DIRECTION('center_axis',(0.,0.,-1.));
#34188=DIRECTION('ref_axis',(1.,0.,0.));
#34189=DIRECTION('center_axis',(0.,0.,-1.));
#34190=DIRECTION('ref_axis',(1.,0.,0.));
#34191=DIRECTION('',(0.,0.,-1.));
#34192=DIRECTION('center_axis',(0.,0.,1.));
#34193=DIRECTION('ref_axis',(1.,0.,0.));
#34194=DIRECTION('',(0.707106781186547,8.65956056235493E-17,-0.707106781186547));
#34195=DIRECTION('center_axis',(0.,0.,-1.));
#34196=DIRECTION('ref_axis',(1.,0.,0.));
#34197=DIRECTION('center_axis',(0.,0.,-1.));
#34198=DIRECTION('ref_axis',(1.,0.,0.));
#34199=DIRECTION('',(0.,0.,-1.));
#34200=DIRECTION('center_axis',(0.,0.,-1.));
#34201=DIRECTION('ref_axis',(1.,0.,0.));
#34202=DIRECTION('',(0.707106781186547,-8.65956056235493E-17,0.707106781186548));
#34203=DIRECTION('center_axis',(0.,0.,-1.));
#34204=DIRECTION('ref_axis',(1.,0.,0.));
#34205=DIRECTION('',(0.707106781186548,-8.65956056235493E-17,0.707106781186548));
#34206=DIRECTION('center_axis',(0.,0.,-1.));
#34207=DIRECTION('ref_axis',(1.,0.,0.));
#34208=DIRECTION('',(0.707106781186548,-8.65956056235493E-17,0.707106781186548));
#34209=DIRECTION('center_axis',(0.,0.,-1.));
#34210=DIRECTION('ref_axis',(1.,0.,0.));
#34211=DIRECTION('',(0.707106781186547,-8.65956056235493E-17,0.707106781186548));
#34212=DIRECTION('center_axis',(0.,1.,0.));
#34213=DIRECTION('ref_axis',(1.,0.,0.));
#34214=DIRECTION('center_axis',(0.,1.,0.));
#34215=DIRECTION('ref_axis',(1.,0.,0.));
#34216=DIRECTION('center_axis',(0.,0.,1.));
#34217=DIRECTION('ref_axis',(1.,0.,0.));
#34218=DIRECTION('center_axis',(0.,0.,1.));
#34219=DIRECTION('ref_axis',(1.,0.,0.));
#34220=DIRECTION('center_axis',(0.,0.,1.));
#34221=DIRECTION('ref_axis',(1.,0.,0.));
#34222=DIRECTION('center_axis',(0.,0.,1.));
#34223=DIRECTION('ref_axis',(1.,0.,0.));
#34224=DIRECTION('center_axis',(0.,0.,1.));
#34225=DIRECTION('ref_axis',(1.,0.,0.));
#34226=DIRECTION('center_axis',(0.,0.,1.));
#34227=DIRECTION('ref_axis',(1.,0.,0.));
#34228=DIRECTION('center_axis',(0.,0.,1.));
#34229=DIRECTION('ref_axis',(1.,0.,0.));
#34230=DIRECTION('center_axis',(0.,0.,1.));
#34231=DIRECTION('ref_axis',(1.,0.,0.));
#34232=DIRECTION('center_axis',(0.,0.,1.));
#34233=DIRECTION('ref_axis',(1.,0.,0.));
#34234=DIRECTION('center_axis',(0.,0.,1.));
#34235=DIRECTION('ref_axis',(1.,0.,0.));
#34236=DIRECTION('center_axis',(0.,0.,1.));
#34237=DIRECTION('ref_axis',(1.,0.,0.));
#34238=DIRECTION('center_axis',(0.,0.,1.));
#34239=DIRECTION('ref_axis',(1.,0.,0.));
#34240=DIRECTION('center_axis',(0.,0.,-1.));
#34241=DIRECTION('ref_axis',(1.,0.,0.));
#34242=DIRECTION('',(0.,0.,-1.));
#34243=DIRECTION('center_axis',(0.,0.,-1.));
#34244=DIRECTION('ref_axis',(1.,0.,0.));
#34245=DIRECTION('center_axis',(0.,0.,1.));
#34246=DIRECTION('ref_axis',(1.,0.,0.));
#34247=DIRECTION('center_axis',(0.,1.,0.));
#34248=DIRECTION('ref_axis',(-1.,0.,0.));
#40766=CARTESIAN_POINT('',(0.,0.,0.));
#40767=CARTESIAN_POINT('Origin',(85.475,85.475,0.));
#40768=CARTESIAN_POINT('',(85.475,85.475,18.8));
#40769=CARTESIAN_POINT('',(85.725,85.225,18.55));
#40770=CARTESIAN_POINT('',(109.997916666667,60.9520833333331,-5.7229166666665));
#40771=CARTESIAN_POINT('',(85.725,85.225,0.5));
#40772=CARTESIAN_POINT('',(85.725,85.225,0.));
#40773=CARTESIAN_POINT('',(85.475,85.475,0.25));
#40774=CARTESIAN_POINT('',(106.822916666667,64.1270833333331,21.5979166666666));
#40775=CARTESIAN_POINT('',(85.225,85.725,0.5));
#40776=CARTESIAN_POINT('',(78.4145833333332,92.5354166666667,7.31041666666663));
#40777=CARTESIAN_POINT('',(85.225,85.725,18.55));
#40778=CARTESIAN_POINT('',(85.225,85.725,0.));
#40779=CARTESIAN_POINT('',(75.2395833333333,95.7104166666667,8.56458333333343));
#40780=CARTESIAN_POINT('Origin',(85.725,-85.725,0.));
#40781=CARTESIAN_POINT('',(85.725,-85.225,18.55));
#40782=CARTESIAN_POINT('',(85.725,-42.8625,18.55));
#40783=CARTESIAN_POINT('',(85.725,-85.225,0.5));
#40784=CARTESIAN_POINT('',(85.725,-85.225,0.));
#40785=CARTESIAN_POINT('',(85.725,-42.8625,0.5));
#40786=CARTESIAN_POINT('Origin',(85.475,-42.8625,18.8));
#40787=CARTESIAN_POINT('',(85.225,85.225,19.05));
#40788=CARTESIAN_POINT('',(85.225,85.225,19.05));
#40789=CARTESIAN_POINT('',(85.225,-85.225,19.05));
#40790=CARTESIAN_POINT('',(85.225,-42.8625,19.05));
#40791=CARTESIAN_POINT('',(85.475,-85.475,18.8));
#40792=CARTESIAN_POINT('',(85.225,-85.225,19.05));
#40793=CARTESIAN_POINT('',(95.7104166666667,-75.2395833333333,8.56458333333343));
#40794=CARTESIAN_POINT('Origin',(42.8625,85.475,18.8));
#40795=CARTESIAN_POINT('',(-85.225,85.725,18.55));
#40796=CARTESIAN_POINT('',(42.8625,85.725,18.55));
#40797=CARTESIAN_POINT('',(-85.225,85.225,19.05));
#40798=CARTESIAN_POINT('',(-85.225,85.725,18.55));
#40799=CARTESIAN_POINT('',(42.8625,85.225,19.05));
#40800=CARTESIAN_POINT('Origin',(85.475,-85.475,0.));
#40801=CARTESIAN_POINT('',(85.225,-85.725,18.55));
#40802=CARTESIAN_POINT('',(71.4291666666666,-99.5208333333334,4.75416666666677));
#40803=CARTESIAN_POINT('',(85.225,-85.725,0.5));
#40804=CARTESIAN_POINT('',(85.225,-85.725,0.));
#40805=CARTESIAN_POINT('',(85.475,-85.475,0.25));
#40806=CARTESIAN_POINT('',(74.6041666666666,-96.3458333333334,11.1208333333333));
#40807=CARTESIAN_POINT('',(92.5354166666667,-78.4145833333332,7.31041666666663));
#40808=CARTESIAN_POINT('Origin',(85.475,-42.8625,0.25));
#40809=CARTESIAN_POINT('',(85.225,-85.225,0.));
#40810=CARTESIAN_POINT('',(85.225,-85.225,0.));
#40811=CARTESIAN_POINT('',(85.225,85.225,0.));
#40812=CARTESIAN_POINT('',(85.225,-42.8625,0.));
#40813=CARTESIAN_POINT('',(85.225,85.225,0.));
#40814=CARTESIAN_POINT('Origin',(20.,-85.475,0.25));
#40815=CARTESIAN_POINT('',(40.5,-85.725,0.5));
#40816=CARTESIAN_POINT('',(20.,-85.725,0.5));
#40817=CARTESIAN_POINT('',(40.25,-85.475,0.249999999999998));
#40818=CARTESIAN_POINT('',(36.8333333333333,-82.0583333333333,-3.16666666666665));
#40819=CARTESIAN_POINT('',(40.5,-85.225,0.));
#40820=CARTESIAN_POINT('',(40.5,-85.225,0.));
#40821=CARTESIAN_POINT('',(20.,-85.225,0.));
#40822=CARTESIAN_POINT('Origin',(40.,-85.725,0.));
#40823=CARTESIAN_POINT('',(40.5,-85.725,18.55));
#40824=CARTESIAN_POINT('',(20.,-85.725,18.55));
#40825=CARTESIAN_POINT('',(40.5,-85.725,0.));
#40826=CARTESIAN_POINT('',(71.5002890825272,-85.725,7.28103721141815));
#40827=CARTESIAN_POINT('',(74.2629071474075,-85.725,7.28103721141815));
#40828=CARTESIAN_POINT('',(55.7501445412636,-85.725,7.28103721141815));
#40829=CARTESIAN_POINT('',(74.2629071474075,-85.725,6.75000035762787));
#40830=CARTESIAN_POINT('',(74.2629071474075,-85.725,3.64051860570908));
#40831=CARTESIAN_POINT('',(70.9047909975052,-85.725,6.75000035762787));
#40832=CARTESIAN_POINT('',(57.1314535737038,-85.725,6.75000035762787));
#40833=CARTESIAN_POINT('',(70.9047909975052,-85.725,11.2500002384186));
#40834=CARTESIAN_POINT('',(70.9047909975052,-85.725,3.37500017881393));
#40835=CARTESIAN_POINT('',(74.1585417985916,-85.725,11.2500002384186));
#40836=CARTESIAN_POINT('',(55.4523954987526,-85.725,11.2500002384186));
#40837=CARTESIAN_POINT('',(74.1585417985916,-85.725,10.7189633846283));
#40838=CARTESIAN_POINT('',(74.1585417985916,-85.725,5.62500011920929));
#40839=CARTESIAN_POINT('',(71.5002890825272,-85.725,10.7189633846283));
#40840=CARTESIAN_POINT('',(57.0792708992958,-85.725,10.7189633846283));
#40841=CARTESIAN_POINT('',(71.5002890825272,-85.725,9.3407233953476));
#40842=CARTESIAN_POINT('',(71.5002890825272,-85.725,5.35948169231415));
#40843=CARTESIAN_POINT('',(73.989715218544,-85.725,9.3407233953476));
#40844=CARTESIAN_POINT('',(55.7501445412636,-85.725,9.3407233953476));
#40845=CARTESIAN_POINT('',(73.989715218544,-85.725,8.81275618076324));
#40846=CARTESIAN_POINT('',(73.989715218544,-85.725,4.6703616976738));
#40847=CARTESIAN_POINT('',(71.5002890825272,-85.725,8.81275618076324));
#40848=CARTESIAN_POINT('',(56.994857609272,-85.725,8.81275618076324));
#40849=CARTESIAN_POINT('',(71.5002890825272,-85.725,4.40637809038162));
#40850=CARTESIAN_POINT('',(65.901381611824,-85.725,8.74829494953156));
#40851=CARTESIAN_POINT('',(65.210725903511,-85.725,8.74829494953156));
#40852=CARTESIAN_POINT('',(52.950690805912,-85.725,8.74829494953156));
#40853=CARTESIAN_POINT('',(65.210725903511,-85.725,6.75000035762787));
#40854=CARTESIAN_POINT('',(65.210725903511,-85.725,4.37414747476578));
#40855=CARTESIAN_POINT('',(64.6152278184891,-85.725,6.75000035762787));
#40856=CARTESIAN_POINT('',(52.6053629517555,-85.725,6.75000035762787));
#40857=CARTESIAN_POINT('',(64.6152278184891,-85.725,11.2500002384186));
#40858=CARTESIAN_POINT('',(64.6152278184891,-85.725,3.37500017881393));
#40859=CARTESIAN_POINT('',(66.6104527711868,-85.725,11.2500002384186));
#40860=CARTESIAN_POINT('',(52.3076139092445,-85.725,11.2500002384186));
#40861=CARTESIAN_POINT('',(67.5251885652542,-85.725,11.12875187397));
#40862=CARTESIAN_POINT('Ctrl Pts',(66.6104527711868,-85.725,11.2500002384186));
#40863=CARTESIAN_POINT('Ctrl Pts',(67.2120901346207,-85.725,11.2500002384186));
#40864=CARTESIAN_POINT('Ctrl Pts',(67.5251885652542,-85.725,11.12875187397));
#40865=CARTESIAN_POINT('',(68.0255290269852,-85.725,10.7005458474159));
#40866=CARTESIAN_POINT('Ctrl Pts',(67.5251885652542,-85.725,11.12875187397));
#40867=CARTESIAN_POINT('Ctrl Pts',(67.838284611702,-85.725,11.0075035095215));
#40868=CARTESIAN_POINT('Ctrl Pts',(68.0255290269852,-85.725,10.7005458474159));
#40869=CARTESIAN_POINT('',(68.2127734422684,-85.725,10.0221689939499));
#40870=CARTESIAN_POINT('Ctrl Pts',(68.0255290269852,-85.725,10.7005458474159));
#40871=CARTESIAN_POINT('Ctrl Pts',(68.2127734422684,-85.725,10.3935881853104));
#40872=CARTESIAN_POINT('Ctrl Pts',(68.2127734422684,-85.725,10.0221689939499));
#40873=CARTESIAN_POINT('',(67.9027458429337,-85.725,9.21487057209015));
#40874=CARTESIAN_POINT('Ctrl Pts',(68.2127734422684,-85.725,10.0221689939499));
#40875=CARTESIAN_POINT('Ctrl Pts',(68.2127734422684,-85.725,9.54331541061401));
#40876=CARTESIAN_POINT('Ctrl Pts',(67.9027458429337,-85.725,9.21487057209015));
#40877=CARTESIAN_POINT('',(66.945037484169,-85.725,8.79740798473358));
#40878=CARTESIAN_POINT('Ctrl Pts',(67.9027458429337,-85.725,9.21487057209015));
#40879=CARTESIAN_POINT('Ctrl Pts',(67.5927182435989,-85.725,8.88642573356628));
#40880=CARTESIAN_POINT('Ctrl Pts',(66.945037484169,-85.725,8.79740798473358));
#40881=CARTESIAN_POINT('',(67.3041793107986,-85.725,8.57332909107208));
#40882=CARTESIAN_POINT('Ctrl Pts',(66.945037484169,-85.725,8.79740798473358));
#40883=CARTESIAN_POINT('Ctrl Pts',(67.1813961267471,-85.725,8.68383371829987));
#40884=CARTESIAN_POINT('Ctrl Pts',(67.3041793107986,-85.725,8.57332909107208));
#40885=CARTESIAN_POINT('',(67.7983804941177,-85.725,7.97476136684418));
#40886=CARTESIAN_POINT('Ctrl Pts',(67.3041793107986,-85.725,8.57332909107208));
#40887=CARTESIAN_POINT('Ctrl Pts',(67.5650926828384,-85.725,8.33390200138092));
#40888=CARTESIAN_POINT('Ctrl Pts',(67.7983804941177,-85.725,7.97476136684418));
#40889=CARTESIAN_POINT('',(68.5811229944229,-85.725,6.75000035762787));
#40890=CARTESIAN_POINT('',(65.5769632102546,-85.725,11.450623829166));
#40891=CARTESIAN_POINT('',(67.8321453332901,-85.725,6.75000035762787));
#40892=CARTESIAN_POINT('',(54.2905614972115,-85.725,6.75000035762787));
#40893=CARTESIAN_POINT('',(67.2366472482681,-85.725,7.68622124195099));
#40894=CARTESIAN_POINT('',(65.3520878975123,-85.725,10.6490583463875));
#40895=CARTESIAN_POINT('',(66.8069072961807,-85.725,8.30627584457397));
#40896=CARTESIAN_POINT('Ctrl Pts',(67.2366472482681,-85.725,7.68622124195099));
#40897=CARTESIAN_POINT('Ctrl Pts',(66.9757338762283,-85.725,8.09140527248383));
#40898=CARTESIAN_POINT('Ctrl Pts',(66.8069072961807,-85.725,8.30627584457397));
#40899=CARTESIAN_POINT('',(66.5045520067215,-85.725,8.60709452629089));
#40900=CARTESIAN_POINT('Ctrl Pts',(66.8069072961807,-85.725,8.30627584457397));
#40901=CARTESIAN_POINT('Ctrl Pts',(66.6380807161331,-85.725,8.52114641666412));
#40902=CARTESIAN_POINT('Ctrl Pts',(66.5045520067215,-85.725,8.60709452629089));
#40903=CARTESIAN_POINT('',(66.2328954935074,-85.725,8.72680807113647));
#40904=CARTESIAN_POINT('Ctrl Pts',(66.5045520067215,-85.725,8.60709452629089));
#40905=CARTESIAN_POINT('Ctrl Pts',(66.3710280656815,-85.725,8.69304263591766));
#40906=CARTESIAN_POINT('Ctrl Pts',(66.2328954935074,-85.725,8.72680807113647));
#40907=CARTESIAN_POINT('Ctrl Pts',(66.2328954935074,-85.725,8.72680807113647));
#40908=CARTESIAN_POINT('Ctrl Pts',(66.1315985918045,-85.725,8.74829494953156));
#40909=CARTESIAN_POINT('Ctrl Pts',(65.901381611824,-85.725,8.74829494953156));
#40910=CARTESIAN_POINT('',(61.0207542181015,-85.725,7.28103721141815));
#40911=CARTESIAN_POINT('',(63.7833734750748,-85.725,7.28103721141815));
#40912=CARTESIAN_POINT('',(50.5103771090508,-85.725,7.28103721141815));
#40913=CARTESIAN_POINT('',(63.7833734750748,-85.725,6.75000035762787));
#40914=CARTESIAN_POINT('',(63.7833734750748,-85.725,3.64051860570908));
#40915=CARTESIAN_POINT('',(60.4252561330795,-85.725,6.75000035762787));
#40916=CARTESIAN_POINT('',(51.8916867375374,-85.725,6.75000035762787));
#40917=CARTESIAN_POINT('',(60.4252561330795,-85.725,11.2500002384186));
#40918=CARTESIAN_POINT('',(60.4252561330795,-85.725,3.37500017881393));
#40919=CARTESIAN_POINT('',(63.6790081262589,-85.725,11.2500002384186));
#40920=CARTESIAN_POINT('',(50.2126280665398,-85.725,11.2500002384186));
#40921=CARTESIAN_POINT('',(63.6790081262589,-85.725,10.7189633846283));
#40922=CARTESIAN_POINT('',(63.6790081262589,-85.725,5.62500011920929));
#40923=CARTESIAN_POINT('',(61.0207542181015,-85.725,10.7189633846283));
#40924=CARTESIAN_POINT('',(51.8395040631294,-85.725,10.7189633846283));
#40925=CARTESIAN_POINT('',(61.0207542181015,-85.725,9.3407233953476));
#40926=CARTESIAN_POINT('',(61.0207542181015,-85.725,5.35948169231415));
#40927=CARTESIAN_POINT('',(63.5101815462112,-85.725,9.3407233953476));
#40928=CARTESIAN_POINT('',(50.5103771090508,-85.725,9.3407233953476));
#40929=CARTESIAN_POINT('',(63.5101815462112,-85.725,8.81275618076324));
#40930=CARTESIAN_POINT('',(63.5101815462112,-85.725,4.6703616976738));
#40931=CARTESIAN_POINT('',(61.0207542181015,-85.725,8.81275618076324));
#40932=CARTESIAN_POINT('',(51.7550907731056,-85.725,8.81275618076324));
#40933=CARTESIAN_POINT('',(61.0207542181015,-85.725,4.40637809038162));
#40934=CARTESIAN_POINT('',(51.6278477907181,-85.725,8.033083319664));
#40935=CARTESIAN_POINT('',(52.200324177742,-85.725,9.48345863819122));
#40936=CARTESIAN_POINT('Ctrl Pts',(51.6278477907181,-85.725,8.033083319664));
#40937=CARTESIAN_POINT('Ctrl Pts',(51.827370762825,-85.725,8.7851300239563));
#40938=CARTESIAN_POINT('Ctrl Pts',(52.200324177742,-85.725,9.48345863819122));
#40939=CARTESIAN_POINT('',(52.9938098192215,-85.725,10.6606414318085));
#40940=CARTESIAN_POINT('Ctrl Pts',(52.200324177742,-85.725,9.48345863819122));
#40941=CARTESIAN_POINT('Ctrl Pts',(52.573277592659,-85.725,10.1817872524261));
#40942=CARTESIAN_POINT('Ctrl Pts',(52.9938098192215,-85.725,10.6606414318085));
#40943=CARTESIAN_POINT('',(50.7898535728455,-85.725,10.6606414318085));
#40944=CARTESIAN_POINT('',(46.4969049096107,-85.725,10.6606414318085));
#40945=CARTESIAN_POINT('',(50.7898535728455,-85.725,11.1916782855988));
#40946=CARTESIAN_POINT('',(50.7898535728455,-85.725,5.33032071590424));
#40947=CARTESIAN_POINT('',(53.7028821706772,-85.725,11.1916782855988));
#40948=CARTESIAN_POINT('',(45.3949267864227,-85.725,11.1916782855988));
#40949=CARTESIAN_POINT('',(53.7028821706772,-85.725,10.7619374394417));
#40950=CARTESIAN_POINT('',(53.7028821706772,-85.725,5.59583914279938));
#40951=CARTESIAN_POINT('',(52.8510745763779,-85.725,9.54638504981995));
#40952=CARTESIAN_POINT('Ctrl Pts',(53.7028821706772,-85.725,10.7619374394417));
#40953=CARTESIAN_POINT('Ctrl Pts',(53.2731410264969,-85.725,10.3045704364777));
#40954=CARTESIAN_POINT('Ctrl Pts',(52.8510745763779,-85.725,9.54638504981995));
#40955=CARTESIAN_POINT('',(52.198789358139,-85.725,7.98703992366791));
#40956=CARTESIAN_POINT('Ctrl Pts',(52.8510745763779,-85.725,9.54638504981995));
#40957=CARTESIAN_POINT('Ctrl Pts',(52.4290075302124,-85.725,8.78819906711578));
#40958=CARTESIAN_POINT('Ctrl Pts',(52.198789358139,-85.725,7.98703992366791));
#40959=CARTESIAN_POINT('',(51.9869884252548,-85.725,6.75000035762787));
#40960=CARTESIAN_POINT('Ctrl Pts',(52.198789358139,-85.725,7.98703992366791));
#40961=CARTESIAN_POINT('Ctrl Pts',(52.0330324172974,-85.725,7.42223763465881));
#40962=CARTESIAN_POINT('Ctrl Pts',(51.9869884252548,-85.725,6.75000035762787));
#40963=CARTESIAN_POINT('',(51.4191170930862,-85.725,6.75000035762787));
#40964=CARTESIAN_POINT('',(45.9934942126274,-85.725,6.75000035762787));
#40965=CARTESIAN_POINT('Ctrl Pts',(51.4191170930862,-85.725,6.75000035762787));
#40966=CARTESIAN_POINT('Ctrl Pts',(51.4283254146576,-85.725,7.28103721141815));
#40967=CARTESIAN_POINT('Ctrl Pts',(51.6278477907181,-85.725,8.033083319664));
#40968=CARTESIAN_POINT('',(57.9358288049698,-85.725,6.6732611656189));
#40969=CARTESIAN_POINT('',(56.9121249914169,-85.725,6.8512966632843));
#40970=CARTESIAN_POINT('Ctrl Pts',(57.9358288049698,-85.725,6.6732611656189));
#40971=CARTESIAN_POINT('Ctrl Pts',(57.3249825239182,-85.725,6.6732611656189));
#40972=CARTESIAN_POINT('Ctrl Pts',(56.9121249914169,-85.725,6.8512966632843));
#40973=CARTESIAN_POINT('',(56.264444231987,-85.725,7.38693737983704));
#40974=CARTESIAN_POINT('Ctrl Pts',(56.9121249914169,-85.725,6.8512966632843));
#40975=CARTESIAN_POINT('Ctrl Pts',(56.4992662668228,-85.725,7.02933156490326));
#40976=CARTESIAN_POINT('Ctrl Pts',(56.264444231987,-85.725,7.38693737983704));
#40977=CARTESIAN_POINT('',(56.0173436403275,-85.725,8.19577121734619));
#40978=CARTESIAN_POINT('Ctrl Pts',(56.264444231987,-85.725,7.38693737983704));
#40979=CARTESIAN_POINT('Ctrl Pts',(56.0296221971512,-85.725,7.74454319477081));
#40980=CARTESIAN_POINT('Ctrl Pts',(56.0173436403275,-85.725,8.19577121734619));
#40981=CARTESIAN_POINT('',(56.5790756940842,-85.725,8.24488425254822));
#40982=CARTESIAN_POINT('',(47.7138617611228,-85.725,7.46978594535495));
#40983=CARTESIAN_POINT('',(56.764784693718,-85.725,7.69082570075989));
#40984=CARTESIAN_POINT('Ctrl Pts',(56.5790756940842,-85.725,8.24488425254822));
#40985=CARTESIAN_POINT('Ctrl Pts',(56.6189798116684,-85.725,7.907231092453));
#40986=CARTESIAN_POINT('Ctrl Pts',(56.764784693718,-85.725,7.69082570075989));
#40987=CARTESIAN_POINT('',(57.2175475358963,-85.725,7.34089398384094));
#40988=CARTESIAN_POINT('Ctrl Pts',(56.764784693718,-85.725,7.69082570075989));
#40989=CARTESIAN_POINT('Ctrl Pts',(56.9105907678604,-85.725,7.47442030906677));
#40990=CARTESIAN_POINT('Ctrl Pts',(57.2175475358963,-85.725,7.34089398384094));
#40991=CARTESIAN_POINT('',(57.9082020521164,-85.725,7.20736706256866));
#40992=CARTESIAN_POINT('Ctrl Pts',(57.2175475358963,-85.725,7.34089398384094));
#40993=CARTESIAN_POINT('Ctrl Pts',(57.5245054960251,-85.725,7.20736706256866));
#40994=CARTESIAN_POINT('Ctrl Pts',(57.9082020521164,-85.725,7.20736706256866));
#40995=CARTESIAN_POINT('',(58.5098394155502,-85.725,7.3086633682251));
#40996=CARTESIAN_POINT('Ctrl Pts',(57.9082020521164,-85.725,7.20736706256866));
#40997=CARTESIAN_POINT('Ctrl Pts',(58.2489248514175,-85.725,7.20736706256866));
#40998=CARTESIAN_POINT('Ctrl Pts',(58.5098394155502,-85.725,7.3086633682251));
#40999=CARTESIAN_POINT('',(58.8981410264969,-85.725,7.58645975589752));
#41000=CARTESIAN_POINT('Ctrl Pts',(58.5098394155502,-85.725,7.3086633682251));
#41001=CARTESIAN_POINT('Ctrl Pts',(58.7707539796829,-85.725,7.40995967388153));
#41002=CARTESIAN_POINT('Ctrl Pts',(58.8981410264969,-85.725,7.58645975589752));
#41003=CARTESIAN_POINT('',(59.0255280733109,-85.725,7.97169172763824));
#41004=CARTESIAN_POINT('Ctrl Pts',(58.8981410264969,-85.725,7.58645975589752));
#41005=CARTESIAN_POINT('Ctrl Pts',(59.0255280733109,-85.725,7.76296103000641));
#41006=CARTESIAN_POINT('Ctrl Pts',(59.0255280733109,-85.725,7.97169172763824));
#41007=CARTESIAN_POINT('',(58.9027448892593,-85.725,8.34157609939575));
#41008=CARTESIAN_POINT('Ctrl Pts',(59.0255280733109,-85.725,7.97169172763824));
#41009=CARTESIAN_POINT('Ctrl Pts',(59.0255280733109,-85.725,8.18349266052246));
#41010=CARTESIAN_POINT('Ctrl Pts',(58.9027448892593,-85.725,8.34157609939575));
#41011=CARTESIAN_POINT('',(58.4975608587265,-85.725,8.60709452629089));
#41012=CARTESIAN_POINT('Ctrl Pts',(58.9027448892593,-85.725,8.34157609939575));
#41013=CARTESIAN_POINT('Ctrl Pts',(58.7799617052078,-85.725,8.4996589422226));
#41014=CARTESIAN_POINT('Ctrl Pts',(58.4975608587265,-85.725,8.60709452629089));
#41015=CARTESIAN_POINT('',(57.6964017152786,-85.725,8.82656896114349));
#41016=CARTESIAN_POINT('Ctrl Pts',(58.4975608587265,-85.725,8.60709452629089));
#41017=CARTESIAN_POINT('Ctrl Pts',(58.3164557218552,-85.725,8.677694439888));
#41018=CARTESIAN_POINT('Ctrl Pts',(57.6964017152786,-85.725,8.82656896114349));
#41019=CARTESIAN_POINT('',(56.8277117013931,-85.725,9.1074355840683));
#41020=CARTESIAN_POINT('Ctrl Pts',(57.6964017152786,-85.725,8.82656896114349));
#41021=CARTESIAN_POINT('Ctrl Pts',(57.0763465166092,-85.725,8.97544348239899));
#41022=CARTESIAN_POINT('Ctrl Pts',(56.8277117013931,-85.725,9.1074355840683));
#41023=CARTESIAN_POINT('',(56.3473221063614,-85.725,9.52643239498138));
#41024=CARTESIAN_POINT('Ctrl Pts',(56.8277117013931,-85.725,9.1074355840683));
#41025=CARTESIAN_POINT('Ctrl Pts',(56.5054055452347,-85.725,9.27626216411591));
#41026=CARTESIAN_POINT('Ctrl Pts',(56.3473221063614,-85.725,9.52643239498138));
#41027=CARTESIAN_POINT('',(56.1892386674881,-85.725,10.0866302251816));
#41028=CARTESIAN_POINT('Ctrl Pts',(56.3473221063614,-85.725,9.52643239498138));
#41029=CARTESIAN_POINT('Ctrl Pts',(56.1892386674881,-85.725,9.77660322189331));
#41030=CARTESIAN_POINT('Ctrl Pts',(56.1892386674881,-85.725,10.0866302251816));
#41031=CARTESIAN_POINT('',(56.3826223611832,-85.725,10.723567545414));
#41032=CARTESIAN_POINT('Ctrl Pts',(56.1892386674881,-85.725,10.0866302251816));
#41033=CARTESIAN_POINT('Ctrl Pts',(56.1892386674881,-85.725,10.427353322506));
#41034=CARTESIAN_POINT('Ctrl Pts',(56.3826223611832,-85.725,10.723567545414));
#41035=CARTESIAN_POINT('',(56.9474240541458,-85.725,11.1732607483864));
#41036=CARTESIAN_POINT('Ctrl Pts',(56.3826223611832,-85.725,10.723567545414));
#41037=CARTESIAN_POINT('Ctrl Pts',(56.5760060548782,-85.725,11.019781768322));
#41038=CARTESIAN_POINT('Ctrl Pts',(56.9474240541458,-85.725,11.1732607483864));
#41039=CARTESIAN_POINT('',(57.773141503334,-85.725,11.3267394304276));
#41040=CARTESIAN_POINT('Ctrl Pts',(56.9474240541458,-85.725,11.1732607483864));
#41041=CARTESIAN_POINT('Ctrl Pts',(57.3188432455063,-85.725,11.3267394304276));
#41042=CARTESIAN_POINT('Ctrl Pts',(57.773141503334,-85.725,11.3267394304276));
#41043=CARTESIAN_POINT('',(58.6556442975998,-85.725,11.1655866503716));
#41044=CARTESIAN_POINT('Ctrl Pts',(57.773141503334,-85.725,11.3267394304276));
#41045=CARTESIAN_POINT('Ctrl Pts',(58.273481965065,-85.725,11.3267394304276));
#41046=CARTESIAN_POINT('Ctrl Pts',(58.6556442975998,-85.725,11.1655866503716));
#41047=CARTESIAN_POINT('',(59.2434688806534,-85.725,10.6913369297981));
#41048=CARTESIAN_POINT('Ctrl Pts',(58.6556442975998,-85.725,11.1655866503716));
#41049=CARTESIAN_POINT('Ctrl Pts',(59.0378066301346,-85.725,11.0044338703156));
#41050=CARTESIAN_POINT('Ctrl Pts',(59.2434688806534,-85.725,10.6913369297981));
#41051=CARTESIAN_POINT('',(59.4644781351089,-85.725,9.98226487636566));
#41052=CARTESIAN_POINT('Ctrl Pts',(59.2434688806534,-85.725,10.6913369297981));
#41053=CARTESIAN_POINT('Ctrl Pts',(59.4491299390793,-85.725,10.3782402873039));
#41054=CARTESIAN_POINT('Ctrl Pts',(59.4644781351089,-85.725,9.98226487636566));
#41055=CARTESIAN_POINT('',(58.8935371637344,-85.725,9.9392911195755));
#41056=CARTESIAN_POINT('',(49.4135069487441,-85.725,9.22574535346662));
#41057=CARTESIAN_POINT('',(58.5819741487503,-85.725,10.5839019417763));
#41058=CARTESIAN_POINT('Ctrl Pts',(58.8935371637344,-85.725,9.9392911195755));
#41059=CARTESIAN_POINT('Ctrl Pts',(58.8474925756454,-85.725,10.3659620285034));
#41060=CARTESIAN_POINT('Ctrl Pts',(58.5819741487503,-85.725,10.5839019417763));
#41061=CARTESIAN_POINT('',(57.7976974248886,-85.725,10.8018418550491));
#41062=CARTESIAN_POINT('Ctrl Pts',(58.5819741487503,-85.725,10.5839019417763));
#41063=CARTESIAN_POINT('Ctrl Pts',(58.3164557218552,-85.725,10.8018418550491));
#41064=CARTESIAN_POINT('Ctrl Pts',(57.7976974248886,-85.725,10.8018418550491));
#41065=CARTESIAN_POINT('',(57.010351061821,-85.725,10.6038540005684));
#41066=CARTESIAN_POINT('Ctrl Pts',(57.7976974248886,-85.725,10.8018418550491));
#41067=CARTESIAN_POINT('Ctrl Pts',(57.2574516534805,-85.725,10.8018418550491));
#41068=CARTESIAN_POINT('Ctrl Pts',(57.010351061821,-85.725,10.6038540005684));
#41069=CARTESIAN_POINT('',(56.7632504701614,-85.725,10.1265349388123));
#41070=CARTESIAN_POINT('Ctrl Pts',(57.010351061821,-85.725,10.6038540005684));
#41071=CARTESIAN_POINT('Ctrl Pts',(56.7632504701614,-85.725,10.4058664441109));
#41072=CARTESIAN_POINT('Ctrl Pts',(56.7632504701614,-85.725,10.1265349388123));
#41073=CARTESIAN_POINT('',(56.9382163286209,-85.725,9.72748959064484));
#41074=CARTESIAN_POINT('Ctrl Pts',(56.7632504701614,-85.725,10.1265349388123));
#41075=CARTESIAN_POINT('Ctrl Pts',(56.7632504701614,-85.725,9.88403820991516));
#41076=CARTESIAN_POINT('Ctrl Pts',(56.9382163286209,-85.725,9.72748959064484));
#41077=CARTESIAN_POINT('',(57.8360673189163,-85.725,9.4067188501358));
#41078=CARTESIAN_POINT('Ctrl Pts',(56.9382163286209,-85.725,9.72748959064484));
#41079=CARTESIAN_POINT('Ctrl Pts',(57.1101125478745,-85.725,9.57094156742096));
#41080=CARTESIAN_POINT('Ctrl Pts',(57.8360673189163,-85.725,9.4067188501358));
#41081=CARTESIAN_POINT('',(58.8321443796158,-85.725,9.11971354484558));
#41082=CARTESIAN_POINT('Ctrl Pts',(57.8360673189163,-85.725,9.4067188501358));
#41083=CARTESIAN_POINT('Ctrl Pts',(58.5620220899582,-85.725,9.24249672889709));
#41084=CARTESIAN_POINT('Ctrl Pts',(58.8321443796158,-85.725,9.11971354484558));
#41085=CARTESIAN_POINT('',(59.412295460701,-85.725,8.66081202030182));
#41086=CARTESIAN_POINT('Ctrl Pts',(58.8321443796158,-85.725,9.11971354484558));
#41087=CARTESIAN_POINT('Ctrl Pts',(59.2250510454178,-85.725,8.93860900402069));
#41088=CARTESIAN_POINT('Ctrl Pts',(59.412295460701,-85.725,8.66081202030182));
#41089=CARTESIAN_POINT('',(59.5995398759842,-85.725,8.02080535888672));
#41090=CARTESIAN_POINT('Ctrl Pts',(59.412295460701,-85.725,8.66081202030182));
#41091=CARTESIAN_POINT('Ctrl Pts',(59.5995398759842,-85.725,8.38301503658295));
#41092=CARTESIAN_POINT('Ctrl Pts',(59.5995398759842,-85.725,8.02080535888672));
#41093=CARTESIAN_POINT('',(59.3938776254654,-85.725,7.34396362304687));
#41094=CARTESIAN_POINT('Ctrl Pts',(59.5995398759842,-85.725,8.02080535888672));
#41095=CARTESIAN_POINT('Ctrl Pts',(59.5995398759842,-85.725,7.66166472434997));
#41096=CARTESIAN_POINT('Ctrl Pts',(59.3938776254654,-85.725,7.34396362304687));
#41097=CARTESIAN_POINT('',(58.8029834032059,-85.725,6.84976184368133));
#41098=CARTESIAN_POINT('Ctrl Pts',(59.3938776254654,-85.725,7.34396362304687));
#41099=CARTESIAN_POINT('Ctrl Pts',(59.1882153749466,-85.725,7.02626252174377));
#41100=CARTESIAN_POINT('Ctrl Pts',(58.8029834032059,-85.725,6.84976184368133));
#41101=CARTESIAN_POINT('Ctrl Pts',(58.8029834032059,-85.725,6.84976184368133));
#41102=CARTESIAN_POINT('Ctrl Pts',(58.417752623558,-85.725,6.6732611656189));
#41103=CARTESIAN_POINT('Ctrl Pts',(57.9358288049698,-85.725,6.6732611656189));
#41104=CARTESIAN_POINT('',(49.7768934965134,-85.725,7.0799800157547));
#41105=CARTESIAN_POINT('',(48.6902626752853,-85.725,6.67019152641296));
#41106=CARTESIAN_POINT('Ctrl Pts',(49.7768934965134,-85.725,7.0799800157547));
#41107=CARTESIAN_POINT('Ctrl Pts',(49.3471523523331,-85.725,6.67019152641296));
#41108=CARTESIAN_POINT('Ctrl Pts',(48.6902626752853,-85.725,6.67019152641296));
#41109=CARTESIAN_POINT('',(47.7064635753632,-85.725,7.02319288253784));
#41110=CARTESIAN_POINT('Ctrl Pts',(48.6902626752853,-85.725,6.67019152641296));
#41111=CARTESIAN_POINT('Ctrl Pts',(48.0978345274925,-85.725,6.67019152641296));
#41112=CARTESIAN_POINT('Ctrl Pts',(47.7064635753632,-85.725,7.02319288253784));
#41113=CARTESIAN_POINT('',(47.2598400115967,-85.725,7.93792688846588));
#41114=CARTESIAN_POINT('Ctrl Pts',(47.7064635753632,-85.725,7.02319288253784));
#41115=CARTESIAN_POINT('Ctrl Pts',(47.3150923252106,-85.725,7.37619423866272));
#41116=CARTESIAN_POINT('Ctrl Pts',(47.2598400115967,-85.725,7.93792688846588));
#41117=CARTESIAN_POINT('',(47.812363743782,-85.725,8.01159644126892));
#41118=CARTESIAN_POINT('',(43.1733746033117,-85.725,7.39306689126227));
#41119=CARTESIAN_POINT('',(48.136204123497,-85.725,7.33475470542908));
#41120=CARTESIAN_POINT('Ctrl Pts',(47.812363743782,-85.725,8.01159644126892));
#41121=CARTESIAN_POINT('Ctrl Pts',(47.9075207710266,-85.725,7.54195117950439));
#41122=CARTESIAN_POINT('Ctrl Pts',(48.136204123497,-85.725,7.33475470542908));
#41123=CARTESIAN_POINT('',(48.6933323144913,-85.725,7.12755823135376));
#41124=CARTESIAN_POINT('Ctrl Pts',(48.136204123497,-85.725,7.33475470542908));
#41125=CARTESIAN_POINT('Ctrl Pts',(48.3648877739906,-85.725,7.12755823135376));
#41126=CARTESIAN_POINT('Ctrl Pts',(48.6933323144913,-85.725,7.12755823135376));
#41127=CARTESIAN_POINT('',(49.351756811142,-85.725,7.3976811170578));
#41128=CARTESIAN_POINT('Ctrl Pts',(48.6933323144913,-85.725,7.12755823135376));
#41129=CARTESIAN_POINT('Ctrl Pts',(49.0831687450409,-85.725,7.12755823135376));
#41130=CARTESIAN_POINT('Ctrl Pts',(49.351756811142,-85.725,7.3976811170578));
#41131=CARTESIAN_POINT('',(49.620344877243,-85.725,8.06684875488281));
#41132=CARTESIAN_POINT('Ctrl Pts',(49.351756811142,-85.725,7.3976811170578));
#41133=CARTESIAN_POINT('Ctrl Pts',(49.620344877243,-85.725,7.66780400276184));
#41134=CARTESIAN_POINT('Ctrl Pts',(49.620344877243,-85.725,8.06684875488281));
#41135=CARTESIAN_POINT('',(49.3717088699341,-85.725,8.69457745552063));
#41136=CARTESIAN_POINT('Ctrl Pts',(49.620344877243,-85.725,8.06684875488281));
#41137=CARTESIAN_POINT('Ctrl Pts',(49.620344877243,-85.725,8.44747626781464));
#41138=CARTESIAN_POINT('Ctrl Pts',(49.3717088699341,-85.725,8.69457745552063));
#41139=CARTESIAN_POINT('',(48.7393763065338,-85.725,8.94167864322662));
#41140=CARTESIAN_POINT('Ctrl Pts',(49.3717088699341,-85.725,8.69457745552063));
#41141=CARTESIAN_POINT('Ctrl Pts',(49.1230734586716,-85.725,8.94167864322662));
#41142=CARTESIAN_POINT('Ctrl Pts',(48.7393763065338,-85.725,8.94167864322662));
#41143=CARTESIAN_POINT('',(48.3495398759842,-85.725,8.88028705120087));
#41144=CARTESIAN_POINT('Ctrl Pts',(48.7393763065338,-85.725,8.94167864322662));
#41145=CARTESIAN_POINT('Ctrl Pts',(48.5828276872635,-85.725,8.94167864322662));
#41146=CARTESIAN_POINT('Ctrl Pts',(48.3495398759842,-85.725,8.88028705120087));
#41147=CARTESIAN_POINT('',(48.4109314680099,-85.725,9.36527991294861));
#41148=CARTESIAN_POINT('',(47.7305213298712,-85.725,3.99004774891496));
#41149=CARTESIAN_POINT('',(48.4999492168427,-85.725,9.35914063453674));
#41150=CARTESIAN_POINT('Ctrl Pts',(48.4109314680099,-85.725,9.36527991294861));
#41151=CARTESIAN_POINT('Ctrl Pts',(48.4661837816238,-85.725,9.35914063453674));
#41152=CARTESIAN_POINT('Ctrl Pts',(48.4999492168427,-85.725,9.35914063453674));
#41153=CARTESIAN_POINT('',(49.1353514194489,-85.725,9.54331481456757));
#41154=CARTESIAN_POINT('Ctrl Pts',(48.4999492168427,-85.725,9.35914063453674));
#41155=CARTESIAN_POINT('Ctrl Pts',(48.8529505729675,-85.725,9.35914063453674));
#41156=CARTESIAN_POINT('Ctrl Pts',(49.1353514194489,-85.725,9.54331481456757));
#41157=CARTESIAN_POINT('',(49.4177528619766,-85.725,10.111187338829));
#41158=CARTESIAN_POINT('Ctrl Pts',(49.1353514194489,-85.725,9.54331481456757));
#41159=CARTESIAN_POINT('Ctrl Pts',(49.4177528619766,-85.725,9.72748959064484));
#41160=CARTESIAN_POINT('Ctrl Pts',(49.4177528619766,-85.725,10.111187338829));
#41161=CARTESIAN_POINT('',(49.2120906114578,-85.725,10.6145974397659));
#41162=CARTESIAN_POINT('Ctrl Pts',(49.4177528619766,-85.725,10.111187338829));
#41163=CARTESIAN_POINT('Ctrl Pts',(49.4177528619766,-85.725,10.4150750637054));
#41164=CARTESIAN_POINT('Ctrl Pts',(49.2120906114578,-85.725,10.6145974397659));
#41165=CARTESIAN_POINT('',(48.6810540556908,-85.725,10.8141201138496));
#41166=CARTESIAN_POINT('Ctrl Pts',(49.2120906114578,-85.725,10.6145974397659));
#41167=CARTESIAN_POINT('Ctrl Pts',(49.0064295530319,-85.725,10.8141201138496));
#41168=CARTESIAN_POINT('Ctrl Pts',(48.6810540556908,-85.725,10.8141201138496));
#41169=CARTESIAN_POINT('',(48.1438782215118,-85.725,10.6115280985832));
#41170=CARTESIAN_POINT('Ctrl Pts',(48.6810540556908,-85.725,10.8141201138496));
#41171=CARTESIAN_POINT('Ctrl Pts',(48.3587484955788,-85.725,10.8141201138496));
#41172=CARTESIAN_POINT('Ctrl Pts',(48.1438782215118,-85.725,10.6115280985832));
#41173=CARTESIAN_POINT('',(47.8676160573959,-85.725,10.0037517547607));
#41174=CARTESIAN_POINT('Ctrl Pts',(48.1438782215118,-85.725,10.6115280985832));
#41175=CARTESIAN_POINT('Ctrl Pts',(47.9290076494217,-85.725,10.4089357852936));
#41176=CARTESIAN_POINT('Ctrl Pts',(47.8676160573959,-85.725,10.0037517547607));
#41177=CARTESIAN_POINT('',(47.3150923252106,-85.725,10.1019784212112));
#41178=CARTESIAN_POINT('',(44.9163087580087,-85.725,10.528429810748));
#41179=CARTESIAN_POINT('',(47.7755289673805,-85.725,10.9629946351051));
#41180=CARTESIAN_POINT('Ctrl Pts',(47.3150923252106,-85.725,10.1019784212112));
#41181=CARTESIAN_POINT('Ctrl Pts',(47.4163883328438,-85.725,10.6575717926025));
#41182=CARTESIAN_POINT('Ctrl Pts',(47.7755289673805,-85.725,10.9629946351051));
#41183=CARTESIAN_POINT('',(48.6687757968903,-85.725,11.2684174776077));
#41184=CARTESIAN_POINT('Ctrl Pts',(47.7755289673805,-85.725,10.9629946351051));
#41185=CARTESIAN_POINT('Ctrl Pts',(48.134669303894,-85.725,11.2684174776077));
#41186=CARTESIAN_POINT('Ctrl Pts',(48.6687757968903,-85.725,11.2684174776077));
#41187=CARTESIAN_POINT('',(49.3471523523331,-85.725,11.1103343367577));
#41188=CARTESIAN_POINT('Ctrl Pts',(48.6687757968903,-85.725,11.2684174776077));
#41189=CARTESIAN_POINT('Ctrl Pts',(49.0371247529984,-85.725,11.2684174776077));
#41190=CARTESIAN_POINT('Ctrl Pts',(49.3471523523331,-85.725,11.1103343367577));
#41191=CARTESIAN_POINT('',(49.8214020729065,-85.725,10.6790586709976));
#41192=CARTESIAN_POINT('Ctrl Pts',(49.3471523523331,-85.725,11.1103343367577));
#41193=CARTESIAN_POINT('Ctrl Pts',(49.6571799516678,-85.725,10.9522508978844));
#41194=CARTESIAN_POINT('Ctrl Pts',(49.8214020729065,-85.725,10.6790586709976));
#41195=CARTESIAN_POINT('',(49.9856241941452,-85.725,10.0989087820053));
#41196=CARTESIAN_POINT('Ctrl Pts',(49.8214020729065,-85.725,10.6790586709976));
#41197=CARTESIAN_POINT('Ctrl Pts',(49.9856241941452,-85.725,10.4058664441109));
#41198=CARTESIAN_POINT('Ctrl Pts',(49.9856241941452,-85.725,10.0989087820053));
#41199=CARTESIAN_POINT('',(49.8290761709213,-85.725,9.56787192821503));
#41200=CARTESIAN_POINT('Ctrl Pts',(49.9856241941452,-85.725,10.0989087820053));
#41201=CARTESIAN_POINT('Ctrl Pts',(49.9856241941452,-85.725,9.80729901790619));
#41202=CARTESIAN_POINT('Ctrl Pts',(49.8290761709213,-85.725,9.56787192821503));
#41203=CARTESIAN_POINT('',(49.3655695915222,-85.725,9.1872444152832));
#41204=CARTESIAN_POINT('Ctrl Pts',(49.8290761709213,-85.725,9.56787192821503));
#41205=CARTESIAN_POINT('Ctrl Pts',(49.672527551651,-85.725,9.32844483852386));
#41206=CARTESIAN_POINT('Ctrl Pts',(49.3655695915222,-85.725,9.1872444152832));
#41207=CARTESIAN_POINT('',(49.9856241941452,-85.725,8.80508208274841));
#41208=CARTESIAN_POINT('Ctrl Pts',(49.3655695915222,-85.725,9.1872444152832));
#41209=CARTESIAN_POINT('Ctrl Pts',(49.7646149396896,-85.725,9.09515702724457));
#41210=CARTESIAN_POINT('Ctrl Pts',(49.9856241941452,-85.725,8.80508208274841));
#41211=CARTESIAN_POINT('',(50.2066334486008,-85.725,8.07912731170654));
#41212=CARTESIAN_POINT('Ctrl Pts',(49.9856241941452,-85.725,8.80508208274841));
#41213=CARTESIAN_POINT('Ctrl Pts',(50.2066334486008,-85.725,8.51500713825226));
#41214=CARTESIAN_POINT('Ctrl Pts',(50.2066334486008,-85.725,8.07912731170654));
#41215=CARTESIAN_POINT('Ctrl Pts',(50.2066334486008,-85.725,8.07912731170654));
#41216=CARTESIAN_POINT('Ctrl Pts',(50.2066334486008,-85.725,7.48976850509643));
#41217=CARTESIAN_POINT('Ctrl Pts',(49.7768934965134,-85.725,7.0799800157547));
#41218=CARTESIAN_POINT('',(69.2472215890884,-85.725,11.2500002384186));
#41219=CARTESIAN_POINT('',(69.8427196741104,-85.725,11.2500002384186));
#41220=CARTESIAN_POINT('',(54.6236107945442,-85.725,11.2500002384186));
#41221=CARTESIAN_POINT('',(69.8427196741104,-85.725,6.75000035762787));
#41222=CARTESIAN_POINT('',(69.8427196741104,-85.725,5.62500011920929));
#41223=CARTESIAN_POINT('',(69.2472215890884,-85.725,6.75000035762787));
#41224=CARTESIAN_POINT('',(54.9213598370552,-85.725,6.75000035762787));
#41225=CARTESIAN_POINT('',(69.2472215890884,-85.725,3.37500017881393));
#41226=CARTESIAN_POINT('',(76.8014498949051,-85.725,6.6732611656189));
#41227=CARTESIAN_POINT('',(75.7777472734451,-85.725,6.8512966632843));
#41228=CARTESIAN_POINT('Ctrl Pts',(76.8014498949051,-85.725,6.6732611656189));
#41229=CARTESIAN_POINT('Ctrl Pts',(76.1906048059464,-85.725,6.6732611656189));
#41230=CARTESIAN_POINT('Ctrl Pts',(75.7777472734451,-85.725,6.8512966632843));
#41231=CARTESIAN_POINT('',(75.1300665140152,-85.725,7.38693737983704));
#41232=CARTESIAN_POINT('Ctrl Pts',(75.7777472734451,-85.725,6.8512966632843));
#41233=CARTESIAN_POINT('Ctrl Pts',(75.3648873567581,-85.725,7.02933156490326));
#41234=CARTESIAN_POINT('Ctrl Pts',(75.1300665140152,-85.725,7.38693737983704));
#41235=CARTESIAN_POINT('',(74.8829647302628,-85.725,8.19577121734619));
#41236=CARTESIAN_POINT('Ctrl Pts',(75.1300665140152,-85.725,7.38693737983704));
#41237=CARTESIAN_POINT('Ctrl Pts',(74.8952432870865,-85.725,7.74454319477081));
#41238=CARTESIAN_POINT('Ctrl Pts',(74.8829647302628,-85.725,8.19577121734619));
#41239=CARTESIAN_POINT('',(75.4446979761124,-85.725,8.24488425254822));
#41240=CARTESIAN_POINT('',(57.2182322749014,-85.725,6.65132172405981));
#41241=CARTESIAN_POINT('',(75.6304069757462,-85.725,7.69082570075989));
#41242=CARTESIAN_POINT('Ctrl Pts',(75.4446979761124,-85.725,8.24488425254822));
#41243=CARTESIAN_POINT('Ctrl Pts',(75.4846020936966,-85.725,7.907231092453));
#41244=CARTESIAN_POINT('Ctrl Pts',(75.6304069757462,-85.725,7.69082570075989));
#41245=CARTESIAN_POINT('',(76.0831686258316,-85.725,7.34089398384094));
#41246=CARTESIAN_POINT('Ctrl Pts',(75.6304069757462,-85.725,7.69082570075989));
#41247=CARTESIAN_POINT('Ctrl Pts',(75.7762118577957,-85.725,7.47442030906677));
#41248=CARTESIAN_POINT('Ctrl Pts',(76.0831686258316,-85.725,7.34089398384094));
#41249=CARTESIAN_POINT('',(76.7738243341446,-85.725,7.20736706256866));
#41250=CARTESIAN_POINT('Ctrl Pts',(76.0831686258316,-85.725,7.34089398384094));
#41251=CARTESIAN_POINT('Ctrl Pts',(76.3901277780533,-85.725,7.20736706256866));
#41252=CARTESIAN_POINT('Ctrl Pts',(76.7738243341446,-85.725,7.20736706256866));
#41253=CARTESIAN_POINT('',(77.3754616975784,-85.725,7.3086633682251));
#41254=CARTESIAN_POINT('Ctrl Pts',(76.7738243341446,-85.725,7.20736706256866));
#41255=CARTESIAN_POINT('Ctrl Pts',(77.1145459413528,-85.725,7.20736706256866));
#41256=CARTESIAN_POINT('Ctrl Pts',(77.3754616975784,-85.725,7.3086633682251));
#41257=CARTESIAN_POINT('',(77.7637621164322,-85.725,7.58645975589752));
#41258=CARTESIAN_POINT('Ctrl Pts',(77.3754616975784,-85.725,7.3086633682251));
#41259=CARTESIAN_POINT('Ctrl Pts',(77.6363750696182,-85.725,7.40995967388153));
#41260=CARTESIAN_POINT('Ctrl Pts',(77.7637621164322,-85.725,7.58645975589752));
#41261=CARTESIAN_POINT('',(77.8911491632462,-85.725,7.97169172763824));
#41262=CARTESIAN_POINT('Ctrl Pts',(77.7637621164322,-85.725,7.58645975589752));
#41263=CARTESIAN_POINT('Ctrl Pts',(77.8911491632462,-85.725,7.76296103000641));
#41264=CARTESIAN_POINT('Ctrl Pts',(77.8911491632462,-85.725,7.97169172763824));
#41265=CARTESIAN_POINT('',(77.7683659791946,-85.725,8.34157609939575));
#41266=CARTESIAN_POINT('Ctrl Pts',(77.8911491632462,-85.725,7.97169172763824));
#41267=CARTESIAN_POINT('Ctrl Pts',(77.8911491632462,-85.725,8.18349266052246));
#41268=CARTESIAN_POINT('Ctrl Pts',(77.7683659791946,-85.725,8.34157609939575));
#41269=CARTESIAN_POINT('',(77.3631831407547,-85.725,8.60709452629089));
#41270=CARTESIAN_POINT('Ctrl Pts',(77.7683659791946,-85.725,8.34157609939575));
#41271=CARTESIAN_POINT('Ctrl Pts',(77.6455851793289,-85.725,8.4996589422226));
#41272=CARTESIAN_POINT('Ctrl Pts',(77.3631831407547,-85.725,8.60709452629089));
#41273=CARTESIAN_POINT('',(76.5620228052139,-85.725,8.82656896114349));
#41274=CARTESIAN_POINT('Ctrl Pts',(77.3631831407547,-85.725,8.60709452629089));
#41275=CARTESIAN_POINT('Ctrl Pts',(77.1820780038834,-85.725,8.677694439888));
#41276=CARTESIAN_POINT('Ctrl Pts',(76.5620228052139,-85.725,8.82656896114349));
#41277=CARTESIAN_POINT('',(75.6933327913284,-85.725,9.1074355840683));
#41278=CARTESIAN_POINT('Ctrl Pts',(76.5620228052139,-85.725,8.82656896114349));
#41279=CARTESIAN_POINT('Ctrl Pts',(75.9419699907303,-85.725,8.97544348239899));
#41280=CARTESIAN_POINT('Ctrl Pts',(75.6933327913284,-85.725,9.1074355840683));
#41281=CARTESIAN_POINT('',(75.2129431962967,-85.725,9.52643239498138));
#41282=CARTESIAN_POINT('Ctrl Pts',(75.6933327913284,-85.725,9.1074355840683));
#41283=CARTESIAN_POINT('Ctrl Pts',(75.37102663517,-85.725,9.27626216411591));
#41284=CARTESIAN_POINT('Ctrl Pts',(75.2129431962967,-85.725,9.52643239498138));
#41285=CARTESIAN_POINT('',(75.0548621416092,-85.725,10.0866302251816));
#41286=CARTESIAN_POINT('Ctrl Pts',(75.2129431962967,-85.725,9.52643239498138));
#41287=CARTESIAN_POINT('Ctrl Pts',(75.0548621416092,-85.725,9.77660322189331));
#41288=CARTESIAN_POINT('Ctrl Pts',(75.0548621416092,-85.725,10.0866302251816));
#41289=CARTESIAN_POINT('',(75.2482434511185,-85.725,10.723567545414));
#41290=CARTESIAN_POINT('Ctrl Pts',(75.0548621416092,-85.725,10.0866302251816));
#41291=CARTESIAN_POINT('Ctrl Pts',(75.0548621416092,-85.725,10.427353322506));
#41292=CARTESIAN_POINT('Ctrl Pts',(75.2482434511185,-85.725,10.723567545414));
#41293=CARTESIAN_POINT('',(75.8130475282669,-85.725,11.1732607483864));
#41294=CARTESIAN_POINT('Ctrl Pts',(75.2482434511185,-85.725,10.723567545414));
#41295=CARTESIAN_POINT('Ctrl Pts',(75.4416271448135,-85.725,11.019781768322));
#41296=CARTESIAN_POINT('Ctrl Pts',(75.8130475282669,-85.725,11.1732607483864));
#41297=CARTESIAN_POINT('',(76.6387625932693,-85.725,11.3267394304276));
#41298=CARTESIAN_POINT('Ctrl Pts',(75.8130475282669,-85.725,11.1732607483864));
#41299=CARTESIAN_POINT('Ctrl Pts',(76.1844655275345,-85.725,11.3267394304276));
#41300=CARTESIAN_POINT('Ctrl Pts',(76.6387625932693,-85.725,11.3267394304276));
#41301=CARTESIAN_POINT('',(77.521266579628,-85.725,11.1655866503716));
#41302=CARTESIAN_POINT('Ctrl Pts',(76.6387625932693,-85.725,11.3267394304276));
#41303=CARTESIAN_POINT('Ctrl Pts',(77.1391030550003,-85.725,11.3267394304276));
#41304=CARTESIAN_POINT('Ctrl Pts',(77.521266579628,-85.725,11.1655866503716));
#41305=CARTESIAN_POINT('',(78.1090899705887,-85.725,10.6913369297981));
#41306=CARTESIAN_POINT('Ctrl Pts',(77.521266579628,-85.725,11.1655866503716));
#41307=CARTESIAN_POINT('Ctrl Pts',(77.9034277200699,-85.725,11.0044338703156));
#41308=CARTESIAN_POINT('Ctrl Pts',(78.1090899705887,-85.725,10.6913369297981));
#41309=CARTESIAN_POINT('',(78.3300992250443,-85.725,9.98226487636566));
#41310=CARTESIAN_POINT('Ctrl Pts',(78.1090899705887,-85.725,10.6913369297981));
#41311=CARTESIAN_POINT('Ctrl Pts',(78.3147522211075,-85.725,10.3782402873039));
#41312=CARTESIAN_POINT('Ctrl Pts',(78.3300992250443,-85.725,9.98226487636566));
#41313=CARTESIAN_POINT('',(77.7591582536697,-85.725,9.9392911195755));
#41314=CARTESIAN_POINT('',(58.899456308451,-85.725,8.51975339997975));
#41315=CARTESIAN_POINT('',(77.4475952386856,-85.725,10.5839019417763));
#41316=CARTESIAN_POINT('Ctrl Pts',(77.7591582536697,-85.725,9.9392911195755));
#41317=CARTESIAN_POINT('Ctrl Pts',(77.7131148576736,-85.725,10.3659620285034));
#41318=CARTESIAN_POINT('Ctrl Pts',(77.4475952386856,-85.725,10.5839019417763));
#41319=CARTESIAN_POINT('',(76.6633197069168,-85.725,10.8018418550491));
#41320=CARTESIAN_POINT('Ctrl Pts',(77.4475952386856,-85.725,10.5839019417763));
#41321=CARTESIAN_POINT('Ctrl Pts',(77.1820780038834,-85.725,10.8018418550491));
#41322=CARTESIAN_POINT('Ctrl Pts',(76.6633197069168,-85.725,10.8018418550491));
#41323=CARTESIAN_POINT('',(75.8759733438492,-85.725,10.6038540005684));
#41324=CARTESIAN_POINT('Ctrl Pts',(76.6633197069168,-85.725,10.8018418550491));
#41325=CARTESIAN_POINT('Ctrl Pts',(76.1230727434158,-85.725,10.8018418550491));
#41326=CARTESIAN_POINT('Ctrl Pts',(75.8759733438492,-85.725,10.6038540005684));
#41327=CARTESIAN_POINT('',(75.6288715600967,-85.725,10.1265349388123));
#41328=CARTESIAN_POINT('Ctrl Pts',(75.8759733438492,-85.725,10.6038540005684));
#41329=CARTESIAN_POINT('Ctrl Pts',(75.6288715600967,-85.725,10.4058664441109));
#41330=CARTESIAN_POINT('Ctrl Pts',(75.6288715600967,-85.725,10.1265349388123));
#41331=CARTESIAN_POINT('',(75.8038374185562,-85.725,9.72748959064484));
#41332=CARTESIAN_POINT('Ctrl Pts',(75.6288715600967,-85.725,10.1265349388123));
#41333=CARTESIAN_POINT('Ctrl Pts',(75.6288715600967,-85.725,9.88403820991516));
#41334=CARTESIAN_POINT('Ctrl Pts',(75.8038374185562,-85.725,9.72748959064484));
#41335=CARTESIAN_POINT('',(76.7016884088516,-85.725,9.4067188501358));
#41336=CARTESIAN_POINT('Ctrl Pts',(75.8038374185562,-85.725,9.72748959064484));
#41337=CARTESIAN_POINT('Ctrl Pts',(75.9757348299026,-85.725,9.57094156742096));
#41338=CARTESIAN_POINT('Ctrl Pts',(76.7016884088516,-85.725,9.4067188501358));
#41339=CARTESIAN_POINT('',(77.6977654695511,-85.725,9.11971354484558));
#41340=CARTESIAN_POINT('Ctrl Pts',(76.7016884088516,-85.725,9.4067188501358));
#41341=CARTESIAN_POINT('Ctrl Pts',(77.4276443719864,-85.725,9.24249672889709));
#41342=CARTESIAN_POINT('Ctrl Pts',(77.6977654695511,-85.725,9.11971354484558));
#41343=CARTESIAN_POINT('',(78.2779165506363,-85.725,8.66081202030182));
#41344=CARTESIAN_POINT('Ctrl Pts',(77.6977654695511,-85.725,9.11971354484558));
#41345=CARTESIAN_POINT('Ctrl Pts',(78.0906721353531,-85.725,8.93860900402069));
#41346=CARTESIAN_POINT('Ctrl Pts',(78.2779165506363,-85.725,8.66081202030182));
#41347=CARTESIAN_POINT('',(78.4651609659195,-85.725,8.02080535888672));
#41348=CARTESIAN_POINT('Ctrl Pts',(78.2779165506363,-85.725,8.66081202030182));
#41349=CARTESIAN_POINT('Ctrl Pts',(78.4651609659195,-85.725,8.38301503658295));
#41350=CARTESIAN_POINT('Ctrl Pts',(78.4651609659195,-85.725,8.02080535888672));
#41351=CARTESIAN_POINT('',(78.2594987154007,-85.725,7.34396362304687));
#41352=CARTESIAN_POINT('Ctrl Pts',(78.4651609659195,-85.725,8.02080535888672));
#41353=CARTESIAN_POINT('Ctrl Pts',(78.4651609659195,-85.725,7.66166472434997));
#41354=CARTESIAN_POINT('Ctrl Pts',(78.2594987154007,-85.725,7.34396362304687));
#41355=CARTESIAN_POINT('',(77.668606877327,-85.725,6.84976184368133));
#41356=CARTESIAN_POINT('Ctrl Pts',(78.2594987154007,-85.725,7.34396362304687));
#41357=CARTESIAN_POINT('Ctrl Pts',(78.0538388490677,-85.725,7.02626252174377));
#41358=CARTESIAN_POINT('Ctrl Pts',(77.668606877327,-85.725,6.84976184368133));
#41359=CARTESIAN_POINT('Ctrl Pts',(77.668606877327,-85.725,6.84976184368133));
#41360=CARTESIAN_POINT('Ctrl Pts',(77.2833749055862,-85.725,6.6732611656189));
#41361=CARTESIAN_POINT('Ctrl Pts',(76.8014498949051,-85.725,6.6732611656189));
#41362=CARTESIAN_POINT('Origin',(40.25,-85.475,0.));
#41363=CARTESIAN_POINT('',(40.25,-85.475,18.8));
#41364=CARTESIAN_POINT('',(40.,-85.225,18.55));
#41365=CARTESIAN_POINT('',(26.7645833333334,-71.9895833333334,5.31458333333331));
#41366=CARTESIAN_POINT('',(40.,-85.225,0.5));
#41367=CARTESIAN_POINT('',(40.,-85.225,0.));
#41368=CARTESIAN_POINT('',(29.9395833333334,-75.1645833333334,10.5604166666667));
#41369=CARTESIAN_POINT('',(40.0083333333333,-85.2333333333333,19.0416666666667));
#41370=CARTESIAN_POINT('Origin',(40.25,-23.3625,0.25));
#41371=CARTESIAN_POINT('',(40.,-46.725,0.5));
#41372=CARTESIAN_POINT('',(40.,-23.3625,0.5));
#41373=CARTESIAN_POINT('',(40.5,-46.225,0.));
#41374=CARTESIAN_POINT('',(40.,-46.725,0.5));
#41375=CARTESIAN_POINT('',(40.5,-23.3625,0.));
#41376=CARTESIAN_POINT('Origin',(-33.475,-46.475,10.75));
#41377=CARTESIAN_POINT('',(-35.525,-46.725,10.75));
#41378=CARTESIAN_POINT('Origin',(-33.475,-46.725,10.75));
#41379=CARTESIAN_POINT('',(-35.025,-46.225,10.75));
#41380=CARTESIAN_POINT('',(-35.275,-46.475,10.75));
#41381=CARTESIAN_POINT('Origin',(-33.475,-46.225,10.75));
#41382=CARTESIAN_POINT('Origin',(-85.725,-46.725,0.));
#41383=CARTESIAN_POINT('',(-85.225,-46.725,18.55));
#41384=CARTESIAN_POINT('',(40.,-46.725,18.55));
#41385=CARTESIAN_POINT('',(-42.8625,-46.725,18.55));
#41386=CARTESIAN_POINT('',(-85.225,-46.725,0.5));
#41387=CARTESIAN_POINT('',(-85.225,-46.725,0.));
#41388=CARTESIAN_POINT('',(-42.8625,-46.725,0.5));
#41389=CARTESIAN_POINT('',(40.,-46.725,0.));
#41390=CARTESIAN_POINT('',(-35.525,-46.725,3.75));
#41391=CARTESIAN_POINT('Origin',(-33.475,-46.725,3.75));
#41392=CARTESIAN_POINT('Origin',(-33.475,-46.725,10.75));
#41393=CARTESIAN_POINT('',(-35.025,-35.725,10.75));
#41394=CARTESIAN_POINT('',(-35.025,-46.725,10.75));
#41395=CARTESIAN_POINT('Origin',(-33.475,-35.725,10.75));
#41396=CARTESIAN_POINT('Origin',(-33.475,-46.475,3.75));
#41397=CARTESIAN_POINT('',(-35.025,-46.225,3.75));
#41398=CARTESIAN_POINT('',(-35.275,-46.475,3.75));
#41399=CARTESIAN_POINT('Origin',(-33.475,-46.225,3.75));
#41400=CARTESIAN_POINT('Origin',(-33.475,-46.725,3.75));
#41401=CARTESIAN_POINT('',(-35.025,-35.725,3.75));
#41402=CARTESIAN_POINT('',(-35.025,-46.725,3.75));
#41403=CARTESIAN_POINT('Origin',(-33.475,-35.725,3.75));
#41404=CARTESIAN_POINT('Origin',(0.,37.5,9.8));
#41405=CARTESIAN_POINT('',(-4.5,37.5,9.55));
#41406=CARTESIAN_POINT('Origin',(0.,37.5,9.55));
#41407=CARTESIAN_POINT('',(-5.,37.5,10.05));
#41408=CARTESIAN_POINT('',(-4.75,37.5,9.8));
#41409=CARTESIAN_POINT('Origin',(0.,37.5,10.05));
#41410=CARTESIAN_POINT('Origin',(0.,37.5,19.05));
#41411=CARTESIAN_POINT('',(-4.5,37.5,0.4));
#41412=CARTESIAN_POINT('',(-4.5,37.5,19.05));
#41413=CARTESIAN_POINT('Origin',(0.,37.5,0.4));
#41414=CARTESIAN_POINT('Origin',(0.,37.5,10.05));
#41415=CARTESIAN_POINT('',(-7.,37.5,10.05));
#41416=CARTESIAN_POINT('Origin',(0.,37.5,10.05));
#41417=CARTESIAN_POINT('Origin',(-37.5,0.,9.8));
#41418=CARTESIAN_POINT('',(-42.,5.51091059616309E-16,9.55));
#41419=CARTESIAN_POINT('Origin',(-37.5,0.,9.55));
#41420=CARTESIAN_POINT('',(-42.5,-6.12323399573677E-16,10.05));
#41421=CARTESIAN_POINT('',(-42.25,5.81707229594993E-16,9.8));
#41422=CARTESIAN_POINT('Origin',(-37.5,0.,10.05));
#41423=CARTESIAN_POINT('Origin',(-37.5,0.,19.05));
#41424=CARTESIAN_POINT('',(-42.,-5.51091059616309E-16,0.4));
#41425=CARTESIAN_POINT('',(-42.,5.51091059616309E-16,19.05));
#41426=CARTESIAN_POINT('Origin',(-37.5,0.,0.4));
#41427=CARTESIAN_POINT('Origin',(-37.5,0.,10.05));
#41428=CARTESIAN_POINT('',(-44.5,-8.57252759403147E-16,10.05));
#41429=CARTESIAN_POINT('Origin',(-37.5,0.,10.05));
#41430=CARTESIAN_POINT('Origin',(37.5,0.,9.8));
#41431=CARTESIAN_POINT('',(33.,5.51091059616309E-16,9.55));
#41432=CARTESIAN_POINT('Origin',(37.5,0.,9.55));
#41433=CARTESIAN_POINT('',(32.5,-6.12323399573677E-16,10.05));
#41434=CARTESIAN_POINT('',(32.75,5.81707229594993E-16,9.8));
#41435=CARTESIAN_POINT('Origin',(37.5,0.,10.05));
#41436=CARTESIAN_POINT('Origin',(37.5,0.,19.05));
#41437=CARTESIAN_POINT('',(33.,-5.51091059616309E-16,0.4));
#41438=CARTESIAN_POINT('',(33.,5.51091059616309E-16,19.05));
#41439=CARTESIAN_POINT('Origin',(37.5,0.,0.4));
#41440=CARTESIAN_POINT('Origin',(37.5,0.,10.05));
#41441=CARTESIAN_POINT('',(30.5,-8.57252759403147E-16,10.05));
#41442=CARTESIAN_POINT('Origin',(37.5,0.,10.05));
#41443=CARTESIAN_POINT('Origin',(0.,-37.5,9.8));
#41444=CARTESIAN_POINT('',(-4.5,-37.5,9.55));
#41445=CARTESIAN_POINT('Origin',(0.,-37.5,9.55));
#41446=CARTESIAN_POINT('',(-5.,-37.5,10.05));
#41447=CARTESIAN_POINT('',(-4.75,-37.5,9.8));
#41448=CARTESIAN_POINT('Origin',(0.,-37.5,10.05));
#41449=CARTESIAN_POINT('Origin',(0.,-37.5,19.05));
#41450=CARTESIAN_POINT('',(-4.5,-37.5,0.4));
#41451=CARTESIAN_POINT('',(-4.5,-37.5,19.05));
#41452=CARTESIAN_POINT('Origin',(0.,-37.5,0.4));
#41453=CARTESIAN_POINT('Origin',(0.,-37.5,10.05));
#41454=CARTESIAN_POINT('',(-7.,-37.5,10.05));
#41455=CARTESIAN_POINT('Origin',(0.,-37.5,10.05));
#41456=CARTESIAN_POINT('Origin',(20.,-85.475,18.8));
#41457=CARTESIAN_POINT('',(40.5,-85.225,19.05));
#41458=CARTESIAN_POINT('',(20.,-85.225,19.05));
#41459=CARTESIAN_POINT('',(40.5,-85.225,19.05));
#41460=CARTESIAN_POINT('Origin',(40.25,-23.3625,18.8));
#41461=CARTESIAN_POINT('',(40.5,-46.225,19.05));
#41462=CARTESIAN_POINT('',(40.5,-23.3625,19.05));
#41463=CARTESIAN_POINT('',(40.5,-46.225,19.05));
#41464=CARTESIAN_POINT('',(40.,-23.3625,18.55));
#41465=CARTESIAN_POINT('Origin',(-85.725,85.225,18.55));
#41466=CARTESIAN_POINT('',(-85.725,85.225,18.55));
#41467=CARTESIAN_POINT('',(-85.725,85.225,18.55));
#41468=CARTESIAN_POINT('',(-85.225,85.225,19.05));
#41469=CARTESIAN_POINT('Origin',(-85.225,-46.725,18.55));
#41470=CARTESIAN_POINT('',(-85.725,-46.225,18.55));
#41471=CARTESIAN_POINT('',(-85.225,-46.225,19.05));
#41472=CARTESIAN_POINT('',(-85.725,-46.225,18.55));
#41473=CARTESIAN_POINT('',(-85.225,-46.725,18.55));
#41474=CARTESIAN_POINT('',(-85.225,-46.225,19.05));
#41475=CARTESIAN_POINT('Origin',(-85.225,85.225,0.));
#41476=CARTESIAN_POINT('',(-85.225,85.725,0.5));
#41477=CARTESIAN_POINT('',(-85.725,85.225,0.5));
#41478=CARTESIAN_POINT('',(-85.225,85.725,0.5));
#41479=CARTESIAN_POINT('',(-85.225,85.225,0.));
#41480=CARTESIAN_POINT('',(-85.225,85.225,0.));
#41481=CARTESIAN_POINT('',(-85.725,85.225,0.5));
#41482=CARTESIAN_POINT('Origin',(-85.225,-46.225,0.));
#41483=CARTESIAN_POINT('',(-85.725,-46.225,0.5));
#41484=CARTESIAN_POINT('',(-85.725,-46.225,0.5));
#41485=CARTESIAN_POINT('',(-85.225,-46.225,0.));
#41486=CARTESIAN_POINT('',(-85.225,-46.225,0.));
#41487=CARTESIAN_POINT('',(-85.225,-46.725,0.5));
#41488=CARTESIAN_POINT('Origin',(-85.475,42.8625,0.25));
#41489=CARTESIAN_POINT('',(-85.725,42.8625,0.5));
#41490=CARTESIAN_POINT('',(-85.225,42.8625,0.));
#41491=CARTESIAN_POINT('Origin',(-42.8625,-46.475,0.25));
#41492=CARTESIAN_POINT('',(-42.8625,-46.225,0.));
#41493=CARTESIAN_POINT('Origin',(-85.475,-46.475,0.));
#41494=CARTESIAN_POINT('',(-85.725,-46.225,0.));
#41495=CARTESIAN_POINT('Origin',(42.8625,85.475,0.25));
#41496=CARTESIAN_POINT('',(42.8625,85.225,0.));
#41497=CARTESIAN_POINT('',(42.8625,85.725,0.5));
#41498=CARTESIAN_POINT('Origin',(-85.475,85.475,0.));
#41499=CARTESIAN_POINT('',(-85.225,85.725,0.));
#41500=CARTESIAN_POINT('',(-85.725,85.225,0.));
#41501=CARTESIAN_POINT('Origin',(-42.8625,-46.475,18.8));
#41502=CARTESIAN_POINT('',(-42.8625,-46.225,19.05));
#41503=CARTESIAN_POINT('Origin',(-85.475,42.8625,18.8));
#41504=CARTESIAN_POINT('',(-85.225,42.8625,19.05));
#41505=CARTESIAN_POINT('',(-85.725,42.8625,18.55));
#41506=CARTESIAN_POINT('Origin',(40.,-46.725,0.));
#41507=CARTESIAN_POINT('Origin',(0.,0.,19.05));
#41508=CARTESIAN_POINT('',(52.8,-78.,19.05));
#41509=CARTESIAN_POINT('Origin',(56.25,-78.,19.05));
#41510=CARTESIAN_POINT('',(15.3,78.,19.05));
#41511=CARTESIAN_POINT('Origin',(18.75,78.,19.05));
#41512=CARTESIAN_POINT('',(-22.2,78.,19.05));
#41513=CARTESIAN_POINT('Origin',(-18.75,78.,19.05));
#41514=CARTESIAN_POINT('',(-59.7,78.,19.05));
#41515=CARTESIAN_POINT('Origin',(-56.25,78.,19.05));
#41516=CARTESIAN_POINT('',(74.55,18.75,19.05));
#41517=CARTESIAN_POINT('Origin',(78.,18.75,19.05));
#41518=CARTESIAN_POINT('',(74.55,56.25,19.05));
#41519=CARTESIAN_POINT('Origin',(78.,56.25,19.05));
#41520=CARTESIAN_POINT('',(-7.4,-37.5,19.05));
#41521=CARTESIAN_POINT('Origin',(0.,-37.5,19.05));
#41522=CARTESIAN_POINT('',(-44.9,-9.06238631369042E-16,19.05));
#41523=CARTESIAN_POINT('Origin',(-37.5,0.,19.05));
#41524=CARTESIAN_POINT('',(-5.5,-6.73555739531044E-16,19.05));
#41525=CARTESIAN_POINT('Origin',(0.,0.,19.05));
#41526=CARTESIAN_POINT('',(-7.4,37.5,19.05));
#41527=CARTESIAN_POINT('Origin',(0.,37.5,19.05));
#41528=CARTESIAN_POINT('',(30.1,-9.06238631369042E-16,19.05));
#41529=CARTESIAN_POINT('Origin',(37.5,0.,19.05));
#41530=CARTESIAN_POINT('',(52.8,78.,19.05));
#41531=CARTESIAN_POINT('Origin',(56.25,78.,19.05));
#41532=CARTESIAN_POINT('',(-81.45,18.75,19.05));
#41533=CARTESIAN_POINT('Origin',(-78.,18.75,19.05));
#41534=CARTESIAN_POINT('',(-81.45,-18.75,19.05));
#41535=CARTESIAN_POINT('Origin',(-78.,-18.75,19.05));
#41536=CARTESIAN_POINT('',(74.55,-18.75,19.05));
#41537=CARTESIAN_POINT('Origin',(78.,-18.75,19.05));
#41538=CARTESIAN_POINT('',(74.55,-56.25,19.05));
#41539=CARTESIAN_POINT('Origin',(78.,-56.25,19.05));
#41540=CARTESIAN_POINT('',(-81.45,56.25,19.05));
#41541=CARTESIAN_POINT('Origin',(-78.,56.25,19.05));
#41542=CARTESIAN_POINT('Origin',(-85.725,85.725,0.));
#41543=CARTESIAN_POINT('Origin',(0.,0.,0.));
#41544=CARTESIAN_POINT('',(-4.45,5.44967825620572E-16,0.));
#41545=CARTESIAN_POINT('Origin',(0.,0.,0.));
#41546=CARTESIAN_POINT('',(32.6,6.00076931582203E-16,0.));
#41547=CARTESIAN_POINT('Origin',(37.5,0.,0.));
#41548=CARTESIAN_POINT('',(-4.9,37.5,0.));
#41549=CARTESIAN_POINT('Origin',(0.,37.5,0.));
#41550=CARTESIAN_POINT('',(-42.4,6.00076931582203E-16,0.));
#41551=CARTESIAN_POINT('Origin',(-37.5,0.,0.));
#41552=CARTESIAN_POINT('',(-4.9,-37.5,0.));
#41553=CARTESIAN_POINT('Origin',(0.,-37.5,0.));
#41554=CARTESIAN_POINT('Origin',(71.5002890825272,-85.725,7.28103721141815));
#41555=CARTESIAN_POINT('',(71.5002890825272,-85.425,7.28103721141815));
#41556=CARTESIAN_POINT('',(71.5002890825272,-85.725,7.28103721141815));
#41557=CARTESIAN_POINT('',(74.2629071474075,-85.425,7.28103721141815));
#41558=CARTESIAN_POINT('',(71.5002890825272,-85.425,7.28103721141815));
#41559=CARTESIAN_POINT('',(74.2629071474075,-85.725,7.28103721141815));
#41560=CARTESIAN_POINT('Origin',(71.5002890825272,-85.725,8.81275618076324));
#41561=CARTESIAN_POINT('',(71.5002890825272,-85.425,8.81275618076324));
#41562=CARTESIAN_POINT('',(71.5002890825272,-85.725,8.81275618076324));
#41563=CARTESIAN_POINT('',(71.5002890825272,-85.425,8.81275618076324));
#41564=CARTESIAN_POINT('Origin',(73.989715218544,-85.725,8.81275618076324));
#41565=CARTESIAN_POINT('',(73.989715218544,-85.425,8.81275618076324));
#41566=CARTESIAN_POINT('',(73.989715218544,-85.725,8.81275618076324));
#41567=CARTESIAN_POINT('',(73.989715218544,-85.425,8.81275618076324));
#41568=CARTESIAN_POINT('Origin',(73.989715218544,-85.725,9.3407233953476));
#41569=CARTESIAN_POINT('',(73.989715218544,-85.425,9.3407233953476));
#41570=CARTESIAN_POINT('',(73.989715218544,-85.725,9.3407233953476));
#41571=CARTESIAN_POINT('',(73.989715218544,-85.425,9.3407233953476));
#41572=CARTESIAN_POINT('Origin',(71.5002890825272,-85.725,9.3407233953476));
#41573=CARTESIAN_POINT('',(71.5002890825272,-85.425,9.3407233953476));
#41574=CARTESIAN_POINT('',(71.5002890825272,-85.725,9.3407233953476));
#41575=CARTESIAN_POINT('',(71.5002890825272,-85.425,9.3407233953476));
#41576=CARTESIAN_POINT('Origin',(71.5002890825272,-85.725,10.7189633846283));
#41577=CARTESIAN_POINT('',(71.5002890825272,-85.425,10.7189633846283));
#41578=CARTESIAN_POINT('',(71.5002890825272,-85.725,10.7189633846283));
#41579=CARTESIAN_POINT('',(71.5002890825272,-85.425,10.7189633846283));
#41580=CARTESIAN_POINT('Origin',(74.1585417985916,-85.725,10.7189633846283));
#41581=CARTESIAN_POINT('',(74.1585417985916,-85.425,10.7189633846283));
#41582=CARTESIAN_POINT('',(74.1585417985916,-85.725,10.7189633846283));
#41583=CARTESIAN_POINT('',(74.1585417985916,-85.425,10.7189633846283));
#41584=CARTESIAN_POINT('Origin',(74.1585417985916,-85.725,11.2500002384186));
#41585=CARTESIAN_POINT('',(74.1585417985916,-85.425,11.2500002384186));
#41586=CARTESIAN_POINT('',(74.1585417985916,-85.725,11.2500002384186));
#41587=CARTESIAN_POINT('',(74.1585417985916,-85.425,11.2500002384186));
#41588=CARTESIAN_POINT('Origin',(70.9047909975052,-85.725,11.2500002384186));
#41589=CARTESIAN_POINT('',(70.9047909975052,-85.425,11.2500002384186));
#41590=CARTESIAN_POINT('',(70.9047909975052,-85.725,11.2500002384186));
#41591=CARTESIAN_POINT('',(70.9047909975052,-85.425,11.2500002384186));
#41592=CARTESIAN_POINT('Origin',(70.9047909975052,-85.725,6.75000035762787));
#41593=CARTESIAN_POINT('',(70.9047909975052,-85.425,6.75000035762787));
#41594=CARTESIAN_POINT('',(70.9047909975052,-85.725,6.75000035762787));
#41595=CARTESIAN_POINT('',(70.9047909975052,-85.425,6.75000035762787));
#41596=CARTESIAN_POINT('Origin',(74.2629071474075,-85.725,6.75000035762787));
#41597=CARTESIAN_POINT('',(74.2629071474075,-85.425,6.75000035762787));
#41598=CARTESIAN_POINT('',(74.2629071474075,-85.725,6.75000035762787));
#41599=CARTESIAN_POINT('',(74.2629071474075,-85.425,6.75000035762787));
#41600=CARTESIAN_POINT('Origin',(74.2629071474075,-85.725,7.28103721141815));
#41601=CARTESIAN_POINT('',(74.2629071474075,-85.425,7.28103721141815));
#41602=CARTESIAN_POINT('Origin',(72.5838490724564,-85.425,9.00000029802322));
#41603=CARTESIAN_POINT('Origin',(65.901381611824,-85.725,8.74829494953156));
#41604=CARTESIAN_POINT('',(65.901381611824,-85.425,8.74829494953156));
#41605=CARTESIAN_POINT('',(65.901381611824,-85.725,8.74829494953156));
#41606=CARTESIAN_POINT('',(65.210725903511,-85.425,8.74829494953156));
#41607=CARTESIAN_POINT('',(65.901381611824,-85.425,8.74829494953156));
#41608=CARTESIAN_POINT('',(65.210725903511,-85.725,8.74829494953156));
#41609=CARTESIAN_POINT('Ctrl Pts',(66.2328954935074,-85.725,8.72680807113647));
#41610=CARTESIAN_POINT('Ctrl Pts',(66.2328954935074,-85.425,8.72680807113647));
#41611=CARTESIAN_POINT('Ctrl Pts',(66.1315985918045,-85.725,8.74829494953156));
#41612=CARTESIAN_POINT('Ctrl Pts',(66.1315985918045,-85.425,8.74829494953156));
#41613=CARTESIAN_POINT('Ctrl Pts',(65.901381611824,-85.725,8.74829494953156));
#41614=CARTESIAN_POINT('Ctrl Pts',(65.901381611824,-85.425,8.74829494953156));
#41615=CARTESIAN_POINT('',(66.2328954935074,-85.425,8.72680807113647));
#41616=CARTESIAN_POINT('',(66.2328954935074,-85.725,8.72680807113647));
#41617=CARTESIAN_POINT('Ctrl Pts',(66.2328954935074,-85.425,8.72680807113647));
#41618=CARTESIAN_POINT('Ctrl Pts',(66.1315985918045,-85.425,8.74829494953156));
#41619=CARTESIAN_POINT('Ctrl Pts',(65.901381611824,-85.425,8.74829494953156));
#41620=CARTESIAN_POINT('Ctrl Pts',(66.5045520067215,-85.725,8.60709452629089));
#41621=CARTESIAN_POINT('Ctrl Pts',(66.5045520067215,-85.425,8.60709452629089));
#41622=CARTESIAN_POINT('Ctrl Pts',(66.3710280656815,-85.725,8.69304263591766));
#41623=CARTESIAN_POINT('Ctrl Pts',(66.3710280656815,-85.425,8.69304263591766));
#41624=CARTESIAN_POINT('Ctrl Pts',(66.2328954935074,-85.725,8.72680807113647));
#41625=CARTESIAN_POINT('Ctrl Pts',(66.2328954935074,-85.425,8.72680807113647));
#41626=CARTESIAN_POINT('',(66.5045520067215,-85.425,8.60709452629089));
#41627=CARTESIAN_POINT('',(66.5045520067215,-85.725,8.60709452629089));
#41628=CARTESIAN_POINT('Ctrl Pts',(66.5045520067215,-85.425,8.60709452629089));
#41629=CARTESIAN_POINT('Ctrl Pts',(66.3710280656815,-85.425,8.69304263591766));
#41630=CARTESIAN_POINT('Ctrl Pts',(66.2328954935074,-85.425,8.72680807113647));
#41631=CARTESIAN_POINT('Ctrl Pts',(66.8069072961807,-85.725,8.30627584457397));
#41632=CARTESIAN_POINT('Ctrl Pts',(66.8069072961807,-85.425,8.30627584457397));
#41633=CARTESIAN_POINT('Ctrl Pts',(66.6380807161331,-85.725,8.52114641666412));
#41634=CARTESIAN_POINT('Ctrl Pts',(66.6380807161331,-85.425,8.52114641666412));
#41635=CARTESIAN_POINT('Ctrl Pts',(66.5045520067215,-85.725,8.60709452629089));
#41636=CARTESIAN_POINT('Ctrl Pts',(66.5045520067215,-85.425,8.60709452629089));
#41637=CARTESIAN_POINT('',(66.8069072961807,-85.425,8.30627584457397));
#41638=CARTESIAN_POINT('',(66.8069072961807,-85.725,8.30627584457397));
#41639=CARTESIAN_POINT('Ctrl Pts',(66.8069072961807,-85.425,8.30627584457397));
#41640=CARTESIAN_POINT('Ctrl Pts',(66.6380807161331,-85.425,8.52114641666412));
#41641=CARTESIAN_POINT('Ctrl Pts',(66.5045520067215,-85.425,8.60709452629089));
#41642=CARTESIAN_POINT('Ctrl Pts',(67.2366472482681,-85.725,7.68622124195099));
#41643=CARTESIAN_POINT('Ctrl Pts',(67.2366472482681,-85.425,7.68622124195099));
#41644=CARTESIAN_POINT('Ctrl Pts',(66.9757338762283,-85.725,8.09140527248383));
#41645=CARTESIAN_POINT('Ctrl Pts',(66.9757338762283,-85.425,8.09140527248383));
#41646=CARTESIAN_POINT('Ctrl Pts',(66.8069072961807,-85.725,8.30627584457397));
#41647=CARTESIAN_POINT('Ctrl Pts',(66.8069072961807,-85.425,8.30627584457397));
#41648=CARTESIAN_POINT('',(67.2366472482681,-85.425,7.68622124195099));
#41649=CARTESIAN_POINT('',(67.2366472482681,-85.725,7.68622124195099));
#41650=CARTESIAN_POINT('Ctrl Pts',(67.2366472482681,-85.425,7.68622124195099));
#41651=CARTESIAN_POINT('Ctrl Pts',(66.9757338762283,-85.425,8.09140527248383));
#41652=CARTESIAN_POINT('Ctrl Pts',(66.8069072961807,-85.425,8.30627584457397));
#41653=CARTESIAN_POINT('Origin',(67.8321453332901,-85.725,6.75000035762787));
#41654=CARTESIAN_POINT('',(67.8321453332901,-85.425,6.75000035762787));
#41655=CARTESIAN_POINT('',(67.8321453332901,-85.725,6.75000035762787));
#41656=CARTESIAN_POINT('',(67.8321453332901,-85.425,6.75000035762787));
#41657=CARTESIAN_POINT('Origin',(68.5811229944229,-85.725,6.75000035762787));
#41658=CARTESIAN_POINT('',(68.5811229944229,-85.425,6.75000035762787));
#41659=CARTESIAN_POINT('',(68.5811229944229,-85.725,6.75000035762787));
#41660=CARTESIAN_POINT('',(68.5811229944229,-85.425,6.75000035762787));
#41661=CARTESIAN_POINT('Origin',(67.7983804941177,-85.725,7.97476136684418));
#41662=CARTESIAN_POINT('',(67.7983804941177,-85.425,7.97476136684418));
#41663=CARTESIAN_POINT('',(67.7983804941177,-85.725,7.97476136684418));
#41664=CARTESIAN_POINT('',(67.7983804941177,-85.425,7.97476136684418));
#41665=CARTESIAN_POINT('Ctrl Pts',(67.3041793107986,-85.725,8.57332909107208));
#41666=CARTESIAN_POINT('Ctrl Pts',(67.3041793107986,-85.425,8.57332909107208));
#41667=CARTESIAN_POINT('Ctrl Pts',(67.5650926828384,-85.725,8.33390200138092));
#41668=CARTESIAN_POINT('Ctrl Pts',(67.5650926828384,-85.425,8.33390200138092));
#41669=CARTESIAN_POINT('Ctrl Pts',(67.7983804941177,-85.725,7.97476136684418));
#41670=CARTESIAN_POINT('Ctrl Pts',(67.7983804941177,-85.425,7.97476136684418));
#41671=CARTESIAN_POINT('',(67.3041793107986,-85.425,8.57332909107208));
#41672=CARTESIAN_POINT('',(67.3041793107986,-85.725,8.57332909107208));
#41673=CARTESIAN_POINT('Ctrl Pts',(67.3041793107986,-85.425,8.57332909107208));
#41674=CARTESIAN_POINT('Ctrl Pts',(67.5650926828384,-85.425,8.33390200138092));
#41675=CARTESIAN_POINT('Ctrl Pts',(67.7983804941177,-85.425,7.97476136684418));
#41676=CARTESIAN_POINT('Ctrl Pts',(66.945037484169,-85.725,8.79740798473358));
#41677=CARTESIAN_POINT('Ctrl Pts',(66.945037484169,-85.425,8.79740798473358));
#41678=CARTESIAN_POINT('Ctrl Pts',(67.1813961267471,-85.725,8.68383371829987));
#41679=CARTESIAN_POINT('Ctrl Pts',(67.1813961267471,-85.425,8.68383371829987));
#41680=CARTESIAN_POINT('Ctrl Pts',(67.3041793107986,-85.725,8.57332909107208));
#41681=CARTESIAN_POINT('Ctrl Pts',(67.3041793107986,-85.425,8.57332909107208));
#41682=CARTESIAN_POINT('',(66.945037484169,-85.425,8.79740798473358));
#41683=CARTESIAN_POINT('',(66.945037484169,-85.725,8.79740798473358));
#41684=CARTESIAN_POINT('Ctrl Pts',(66.945037484169,-85.425,8.79740798473358));
#41685=CARTESIAN_POINT('Ctrl Pts',(67.1813961267471,-85.425,8.68383371829987));
#41686=CARTESIAN_POINT('Ctrl Pts',(67.3041793107986,-85.425,8.57332909107208));
#41687=CARTESIAN_POINT('Ctrl Pts',(67.9027458429337,-85.725,9.21487057209015));
#41688=CARTESIAN_POINT('Ctrl Pts',(67.9027458429337,-85.425,9.21487057209015));
#41689=CARTESIAN_POINT('Ctrl Pts',(67.5927182435989,-85.725,8.88642573356628));
#41690=CARTESIAN_POINT('Ctrl Pts',(67.5927182435989,-85.425,8.88642573356628));
#41691=CARTESIAN_POINT('Ctrl Pts',(66.945037484169,-85.725,8.79740798473358));
#41692=CARTESIAN_POINT('Ctrl Pts',(66.945037484169,-85.425,8.79740798473358));
#41693=CARTESIAN_POINT('',(67.9027458429337,-85.425,9.21487057209015));
#41694=CARTESIAN_POINT('',(67.9027458429337,-85.725,9.21487057209015));
#41695=CARTESIAN_POINT('Ctrl Pts',(67.9027458429337,-85.425,9.21487057209015));
#41696=CARTESIAN_POINT('Ctrl Pts',(67.5927182435989,-85.425,8.88642573356628));
#41697=CARTESIAN_POINT('Ctrl Pts',(66.945037484169,-85.425,8.79740798473358));
#41698=CARTESIAN_POINT('Ctrl Pts',(68.2127734422684,-85.725,10.0221689939499));
#41699=CARTESIAN_POINT('Ctrl Pts',(68.2127734422684,-85.425,10.0221689939499));
#41700=CARTESIAN_POINT('Ctrl Pts',(68.2127734422684,-85.725,9.54331541061401));
#41701=CARTESIAN_POINT('Ctrl Pts',(68.2127734422684,-85.425,9.54331541061401));
#41702=CARTESIAN_POINT('Ctrl Pts',(67.9027458429337,-85.725,9.21487057209015));
#41703=CARTESIAN_POINT('Ctrl Pts',(67.9027458429337,-85.425,9.21487057209015));
#41704=CARTESIAN_POINT('',(68.2127734422684,-85.425,10.0221689939499));
#41705=CARTESIAN_POINT('',(68.2127734422684,-85.725,10.0221689939499));
#41706=CARTESIAN_POINT('Ctrl Pts',(68.2127734422684,-85.425,10.0221689939499));
#41707=CARTESIAN_POINT('Ctrl Pts',(68.2127734422684,-85.425,9.54331541061401));
#41708=CARTESIAN_POINT('Ctrl Pts',(67.9027458429337,-85.425,9.21487057209015));
#41709=CARTESIAN_POINT('Ctrl Pts',(68.0255290269852,-85.725,10.7005458474159));
#41710=CARTESIAN_POINT('Ctrl Pts',(68.0255290269852,-85.425,10.7005458474159));
#41711=CARTESIAN_POINT('Ctrl Pts',(68.2127734422684,-85.725,10.3935881853104));
#41712=CARTESIAN_POINT('Ctrl Pts',(68.2127734422684,-85.425,10.3935881853104));
#41713=CARTESIAN_POINT('Ctrl Pts',(68.2127734422684,-85.725,10.0221689939499));
#41714=CARTESIAN_POINT('Ctrl Pts',(68.2127734422684,-85.425,10.0221689939499));
#41715=CARTESIAN_POINT('',(68.0255290269852,-85.425,10.7005458474159));
#41716=CARTESIAN_POINT('',(68.0255290269852,-85.725,10.7005458474159));
#41717=CARTESIAN_POINT('Ctrl Pts',(68.0255290269852,-85.425,10.7005458474159));
#41718=CARTESIAN_POINT('Ctrl Pts',(68.2127734422684,-85.425,10.3935881853104));
#41719=CARTESIAN_POINT('Ctrl Pts',(68.2127734422684,-85.425,10.0221689939499));
#41720=CARTESIAN_POINT('Ctrl Pts',(67.5251885652542,-85.725,11.12875187397));
#41721=CARTESIAN_POINT('Ctrl Pts',(67.5251885652542,-85.425,11.12875187397));
#41722=CARTESIAN_POINT('Ctrl Pts',(67.838284611702,-85.725,11.0075035095215));
#41723=CARTESIAN_POINT('Ctrl Pts',(67.838284611702,-85.425,11.0075035095215));
#41724=CARTESIAN_POINT('Ctrl Pts',(68.0255290269852,-85.725,10.7005458474159));
#41725=CARTESIAN_POINT('Ctrl Pts',(68.0255290269852,-85.425,10.7005458474159));
#41726=CARTESIAN_POINT('',(67.5251885652542,-85.425,11.12875187397));
#41727=CARTESIAN_POINT('',(67.5251885652542,-85.725,11.12875187397));
#41728=CARTESIAN_POINT('Ctrl Pts',(67.5251885652542,-85.425,11.12875187397));
#41729=CARTESIAN_POINT('Ctrl Pts',(67.838284611702,-85.425,11.0075035095215));
#41730=CARTESIAN_POINT('Ctrl Pts',(68.0255290269852,-85.425,10.7005458474159));
#41731=CARTESIAN_POINT('Ctrl Pts',(66.6104527711868,-85.725,11.2500002384186));
#41732=CARTESIAN_POINT('Ctrl Pts',(66.6104527711868,-85.425,11.2500002384186));
#41733=CARTESIAN_POINT('Ctrl Pts',(67.2120901346207,-85.725,11.2500002384186));
#41734=CARTESIAN_POINT('Ctrl Pts',(67.2120901346207,-85.425,11.2500002384186));
#41735=CARTESIAN_POINT('Ctrl Pts',(67.5251885652542,-85.725,11.12875187397));
#41736=CARTESIAN_POINT('Ctrl Pts',(67.5251885652542,-85.425,11.12875187397));
#41737=CARTESIAN_POINT('',(66.6104527711868,-85.425,11.2500002384186));
#41738=CARTESIAN_POINT('',(66.6104527711868,-85.725,11.2500002384186));
#41739=CARTESIAN_POINT('Ctrl Pts',(66.6104527711868,-85.425,11.2500002384186));
#41740=CARTESIAN_POINT('Ctrl Pts',(67.2120901346207,-85.425,11.2500002384186));
#41741=CARTESIAN_POINT('Ctrl Pts',(67.5251885652542,-85.425,11.12875187397));
#41742=CARTESIAN_POINT('Origin',(64.6152278184891,-85.725,11.2500002384186));
#41743=CARTESIAN_POINT('',(64.6152278184891,-85.425,11.2500002384186));
#41744=CARTESIAN_POINT('',(64.6152278184891,-85.725,11.2500002384186));
#41745=CARTESIAN_POINT('',(64.6152278184891,-85.425,11.2500002384186));
#41746=CARTESIAN_POINT('Origin',(64.6152278184891,-85.725,6.75000035762787));
#41747=CARTESIAN_POINT('',(64.6152278184891,-85.425,6.75000035762787));
#41748=CARTESIAN_POINT('',(64.6152278184891,-85.725,6.75000035762787));
#41749=CARTESIAN_POINT('',(64.6152278184891,-85.425,6.75000035762787));
#41750=CARTESIAN_POINT('Origin',(65.210725903511,-85.725,6.75000035762787));
#41751=CARTESIAN_POINT('',(65.210725903511,-85.425,6.75000035762787));
#41752=CARTESIAN_POINT('',(65.210725903511,-85.725,6.75000035762787));
#41753=CARTESIAN_POINT('',(65.210725903511,-85.425,6.75000035762787));
#41754=CARTESIAN_POINT('Origin',(65.210725903511,-85.725,8.74829494953156));
#41755=CARTESIAN_POINT('',(65.210725903511,-85.425,8.74829494953156));
#41756=CARTESIAN_POINT('Origin',(66.598175406456,-85.425,9.00000029802322));
#41757=CARTESIAN_POINT('Origin',(61.0207542181015,-85.725,7.28103721141815));
#41758=CARTESIAN_POINT('',(61.0207542181015,-85.425,7.28103721141815));
#41759=CARTESIAN_POINT('',(61.0207542181015,-85.725,7.28103721141815));
#41760=CARTESIAN_POINT('',(63.7833734750748,-85.425,7.28103721141815));
#41761=CARTESIAN_POINT('',(61.0207542181015,-85.425,7.28103721141815));
#41762=CARTESIAN_POINT('',(63.7833734750748,-85.725,7.28103721141815));
#41763=CARTESIAN_POINT('Origin',(61.0207542181015,-85.725,8.81275618076324));
#41764=CARTESIAN_POINT('',(61.0207542181015,-85.425,8.81275618076324));
#41765=CARTESIAN_POINT('',(61.0207542181015,-85.725,8.81275618076324));
#41766=CARTESIAN_POINT('',(61.0207542181015,-85.425,8.81275618076324));
#41767=CARTESIAN_POINT('Origin',(63.5101815462112,-85.725,8.81275618076324));
#41768=CARTESIAN_POINT('',(63.5101815462112,-85.425,8.81275618076324));
#41769=CARTESIAN_POINT('',(63.5101815462112,-85.725,8.81275618076324));
#41770=CARTESIAN_POINT('',(63.5101815462112,-85.425,8.81275618076324));
#41771=CARTESIAN_POINT('Origin',(63.5101815462112,-85.725,9.3407233953476));
#41772=CARTESIAN_POINT('',(63.5101815462112,-85.425,9.3407233953476));
#41773=CARTESIAN_POINT('',(63.5101815462112,-85.725,9.3407233953476));
#41774=CARTESIAN_POINT('',(63.5101815462112,-85.425,9.3407233953476));
#41775=CARTESIAN_POINT('Origin',(61.0207542181015,-85.725,9.3407233953476));
#41776=CARTESIAN_POINT('',(61.0207542181015,-85.425,9.3407233953476));
#41777=CARTESIAN_POINT('',(61.0207542181015,-85.725,9.3407233953476));
#41778=CARTESIAN_POINT('',(61.0207542181015,-85.425,9.3407233953476));
#41779=CARTESIAN_POINT('Origin',(61.0207542181015,-85.725,10.7189633846283));
#41780=CARTESIAN_POINT('',(61.0207542181015,-85.425,10.7189633846283));
#41781=CARTESIAN_POINT('',(61.0207542181015,-85.725,10.7189633846283));
#41782=CARTESIAN_POINT('',(61.0207542181015,-85.425,10.7189633846283));
#41783=CARTESIAN_POINT('Origin',(63.6790081262589,-85.725,10.7189633846283));
#41784=CARTESIAN_POINT('',(63.6790081262589,-85.425,10.7189633846283));
#41785=CARTESIAN_POINT('',(63.6790081262589,-85.725,10.7189633846283));
#41786=CARTESIAN_POINT('',(63.6790081262589,-85.425,10.7189633846283));
#41787=CARTESIAN_POINT('Origin',(63.6790081262589,-85.725,11.2500002384186));
#41788=CARTESIAN_POINT('',(63.6790081262589,-85.425,11.2500002384186));
#41789=CARTESIAN_POINT('',(63.6790081262589,-85.725,11.2500002384186));
#41790=CARTESIAN_POINT('',(63.6790081262589,-85.425,11.2500002384186));
#41791=CARTESIAN_POINT('Origin',(60.4252561330795,-85.725,11.2500002384186));
#41792=CARTESIAN_POINT('',(60.4252561330795,-85.425,11.2500002384186));
#41793=CARTESIAN_POINT('',(60.4252561330795,-85.725,11.2500002384186));
#41794=CARTESIAN_POINT('',(60.4252561330795,-85.425,11.2500002384186));
#41795=CARTESIAN_POINT('Origin',(60.4252561330795,-85.725,6.75000035762787));
#41796=CARTESIAN_POINT('',(60.4252561330795,-85.425,6.75000035762787));
#41797=CARTESIAN_POINT('',(60.4252561330795,-85.725,6.75000035762787));
#41798=CARTESIAN_POINT('',(60.4252561330795,-85.425,6.75000035762787));
#41799=CARTESIAN_POINT('Origin',(63.7833734750748,-85.725,6.75000035762787));
#41800=CARTESIAN_POINT('',(63.7833734750748,-85.425,6.75000035762787));
#41801=CARTESIAN_POINT('',(63.7833734750748,-85.725,6.75000035762787));
#41802=CARTESIAN_POINT('',(63.7833734750748,-85.425,6.75000035762787));
#41803=CARTESIAN_POINT('Origin',(63.7833734750748,-85.725,7.28103721141815));
#41804=CARTESIAN_POINT('',(63.7833734750748,-85.425,7.28103721141815));
#41805=CARTESIAN_POINT('Origin',(62.1043148040771,-85.425,9.00000029802322));
#41806=CARTESIAN_POINT('Ctrl Pts',(51.6278477907181,-85.725,8.033083319664));
#41807=CARTESIAN_POINT('Ctrl Pts',(51.6278477907181,-85.425,8.033083319664));
#41808=CARTESIAN_POINT('Ctrl Pts',(51.827370762825,-85.725,8.7851300239563));
#41809=CARTESIAN_POINT('Ctrl Pts',(51.827370762825,-85.425,8.7851300239563));
#41810=CARTESIAN_POINT('Ctrl Pts',(52.200324177742,-85.725,9.48345863819122));
#41811=CARTESIAN_POINT('Ctrl Pts',(52.200324177742,-85.425,9.48345863819122));
#41812=CARTESIAN_POINT('',(51.6278477907181,-85.425,8.033083319664));
#41813=CARTESIAN_POINT('',(51.6278477907181,-85.725,8.033083319664));
#41814=CARTESIAN_POINT('',(52.200324177742,-85.425,9.48345863819122));
#41815=CARTESIAN_POINT('Ctrl Pts',(51.6278477907181,-85.425,8.033083319664));
#41816=CARTESIAN_POINT('Ctrl Pts',(51.827370762825,-85.425,8.7851300239563));
#41817=CARTESIAN_POINT('Ctrl Pts',(52.200324177742,-85.425,9.48345863819122));
#41818=CARTESIAN_POINT('',(52.200324177742,-85.725,9.48345863819122));
#41819=CARTESIAN_POINT('Ctrl Pts',(51.4191170930862,-85.725,6.75000035762787));
#41820=CARTESIAN_POINT('Ctrl Pts',(51.4191170930862,-85.425,6.75000035762787));
#41821=CARTESIAN_POINT('Ctrl Pts',(51.4283254146576,-85.725,7.28103721141815));
#41822=CARTESIAN_POINT('Ctrl Pts',(51.4283254146576,-85.425,7.28103721141815));
#41823=CARTESIAN_POINT('Ctrl Pts',(51.6278477907181,-85.725,8.033083319664));
#41824=CARTESIAN_POINT('Ctrl Pts',(51.6278477907181,-85.425,8.033083319664));
#41825=CARTESIAN_POINT('',(51.4191170930862,-85.425,6.75000035762787));
#41826=CARTESIAN_POINT('',(51.4191170930862,-85.725,6.75000035762787));
#41827=CARTESIAN_POINT('Ctrl Pts',(51.4191170930862,-85.425,6.75000035762787));
#41828=CARTESIAN_POINT('Ctrl Pts',(51.4283254146576,-85.425,7.28103721141815));
#41829=CARTESIAN_POINT('Ctrl Pts',(51.6278477907181,-85.425,8.033083319664));
#41830=CARTESIAN_POINT('Origin',(51.9869884252548,-85.725,6.75000035762787));
#41831=CARTESIAN_POINT('',(51.9869884252548,-85.425,6.75000035762787));
#41832=CARTESIAN_POINT('',(51.9869884252548,-85.725,6.75000035762787));
#41833=CARTESIAN_POINT('',(51.9869884252548,-85.425,6.75000035762787));
#41834=CARTESIAN_POINT('Ctrl Pts',(52.198789358139,-85.725,7.98703992366791));
#41835=CARTESIAN_POINT('Ctrl Pts',(52.198789358139,-85.425,7.98703992366791));
#41836=CARTESIAN_POINT('Ctrl Pts',(52.0330324172974,-85.725,7.42223763465881));
#41837=CARTESIAN_POINT('Ctrl Pts',(52.0330324172974,-85.425,7.42223763465881));
#41838=CARTESIAN_POINT('Ctrl Pts',(51.9869884252548,-85.725,6.75000035762787));
#41839=CARTESIAN_POINT('Ctrl Pts',(51.9869884252548,-85.425,6.75000035762787));
#41840=CARTESIAN_POINT('',(52.198789358139,-85.425,7.98703992366791));
#41841=CARTESIAN_POINT('',(52.198789358139,-85.725,7.98703992366791));
#41842=CARTESIAN_POINT('Ctrl Pts',(52.198789358139,-85.425,7.98703992366791));
#41843=CARTESIAN_POINT('Ctrl Pts',(52.0330324172974,-85.425,7.42223763465881));
#41844=CARTESIAN_POINT('Ctrl Pts',(51.9869884252548,-85.425,6.75000035762787));
#41845=CARTESIAN_POINT('Ctrl Pts',(52.8510745763779,-85.725,9.54638504981995));
#41846=CARTESIAN_POINT('Ctrl Pts',(52.8510745763779,-85.425,9.54638504981995));
#41847=CARTESIAN_POINT('Ctrl Pts',(52.4290075302124,-85.725,8.78819906711578));
#41848=CARTESIAN_POINT('Ctrl Pts',(52.4290075302124,-85.425,8.78819906711578));
#41849=CARTESIAN_POINT('Ctrl Pts',(52.198789358139,-85.725,7.98703992366791));
#41850=CARTESIAN_POINT('Ctrl Pts',(52.198789358139,-85.425,7.98703992366791));
#41851=CARTESIAN_POINT('',(52.8510745763779,-85.425,9.54638504981995));
#41852=CARTESIAN_POINT('',(52.8510745763779,-85.725,9.54638504981995));
#41853=CARTESIAN_POINT('Ctrl Pts',(52.8510745763779,-85.425,9.54638504981995));
#41854=CARTESIAN_POINT('Ctrl Pts',(52.4290075302124,-85.425,8.78819906711578));
#41855=CARTESIAN_POINT('Ctrl Pts',(52.198789358139,-85.425,7.98703992366791));
#41856=CARTESIAN_POINT('Ctrl Pts',(53.7028821706772,-85.725,10.7619374394417));
#41857=CARTESIAN_POINT('Ctrl Pts',(53.7028821706772,-85.425,10.7619374394417));
#41858=CARTESIAN_POINT('Ctrl Pts',(53.2731410264969,-85.725,10.3045704364777));
#41859=CARTESIAN_POINT('Ctrl Pts',(53.2731410264969,-85.425,10.3045704364777));
#41860=CARTESIAN_POINT('Ctrl Pts',(52.8510745763779,-85.725,9.54638504981995));
#41861=CARTESIAN_POINT('Ctrl Pts',(52.8510745763779,-85.425,9.54638504981995));
#41862=CARTESIAN_POINT('',(53.7028821706772,-85.425,10.7619374394417));
#41863=CARTESIAN_POINT('',(53.7028821706772,-85.725,10.7619374394417));
#41864=CARTESIAN_POINT('Ctrl Pts',(53.7028821706772,-85.425,10.7619374394417));
#41865=CARTESIAN_POINT('Ctrl Pts',(53.2731410264969,-85.425,10.3045704364777));
#41866=CARTESIAN_POINT('Ctrl Pts',(52.8510745763779,-85.425,9.54638504981995));
#41867=CARTESIAN_POINT('Origin',(53.7028821706772,-85.725,11.1916782855988));
#41868=CARTESIAN_POINT('',(53.7028821706772,-85.425,11.1916782855988));
#41869=CARTESIAN_POINT('',(53.7028821706772,-85.725,11.1916782855988));
#41870=CARTESIAN_POINT('',(53.7028821706772,-85.425,11.1916782855988));
#41871=CARTESIAN_POINT('Origin',(50.7898535728455,-85.725,11.1916782855988));
#41872=CARTESIAN_POINT('',(50.7898535728455,-85.425,11.1916782855988));
#41873=CARTESIAN_POINT('',(50.7898535728455,-85.725,11.1916782855988));
#41874=CARTESIAN_POINT('',(50.7898535728455,-85.425,11.1916782855988));
#41875=CARTESIAN_POINT('Origin',(50.7898535728455,-85.725,10.6606414318085));
#41876=CARTESIAN_POINT('',(50.7898535728455,-85.425,10.6606414318085));
#41877=CARTESIAN_POINT('',(50.7898535728455,-85.725,10.6606414318085));
#41878=CARTESIAN_POINT('',(50.7898535728455,-85.425,10.6606414318085));
#41879=CARTESIAN_POINT('Origin',(52.9938098192215,-85.725,10.6606414318085));
#41880=CARTESIAN_POINT('',(52.9938098192215,-85.425,10.6606414318085));
#41881=CARTESIAN_POINT('',(52.9938098192215,-85.725,10.6606414318085));
#41882=CARTESIAN_POINT('',(52.9938098192215,-85.425,10.6606414318085));
#41883=CARTESIAN_POINT('Ctrl Pts',(52.200324177742,-85.725,9.48345863819122));
#41884=CARTESIAN_POINT('Ctrl Pts',(52.200324177742,-85.425,9.48345863819122));
#41885=CARTESIAN_POINT('Ctrl Pts',(52.573277592659,-85.725,10.1817872524261));
#41886=CARTESIAN_POINT('Ctrl Pts',(52.573277592659,-85.425,10.1817872524261));
#41887=CARTESIAN_POINT('Ctrl Pts',(52.9938098192215,-85.725,10.6606414318085));
#41888=CARTESIAN_POINT('Ctrl Pts',(52.9938098192215,-85.425,10.6606414318085));
#41889=CARTESIAN_POINT('Ctrl Pts',(52.200324177742,-85.425,9.48345863819122));
#41890=CARTESIAN_POINT('Ctrl Pts',(52.573277592659,-85.425,10.1817872524261));
#41891=CARTESIAN_POINT('Ctrl Pts',(52.9938098192215,-85.425,10.6606414318085));
#41892=CARTESIAN_POINT('Origin',(52.2463678717613,-85.425,8.97083932161331));
#41893=CARTESIAN_POINT('Ctrl Pts',(57.9358288049698,-85.725,6.6732611656189));
#41894=CARTESIAN_POINT('Ctrl Pts',(57.9358288049698,-85.425,6.6732611656189));
#41895=CARTESIAN_POINT('Ctrl Pts',(57.3249825239182,-85.725,6.6732611656189));
#41896=CARTESIAN_POINT('Ctrl Pts',(57.3249825239182,-85.425,6.6732611656189));
#41897=CARTESIAN_POINT('Ctrl Pts',(56.9121249914169,-85.725,6.8512966632843));
#41898=CARTESIAN_POINT('Ctrl Pts',(56.9121249914169,-85.425,6.8512966632843));
#41899=CARTESIAN_POINT('',(57.9358288049698,-85.425,6.6732611656189));
#41900=CARTESIAN_POINT('',(57.9358288049698,-85.725,6.6732611656189));
#41901=CARTESIAN_POINT('',(56.9121249914169,-85.425,6.8512966632843));
#41902=CARTESIAN_POINT('Ctrl Pts',(57.9358288049698,-85.425,6.6732611656189));
#41903=CARTESIAN_POINT('Ctrl Pts',(57.3249825239182,-85.425,6.6732611656189));
#41904=CARTESIAN_POINT('Ctrl Pts',(56.9121249914169,-85.425,6.8512966632843));
#41905=CARTESIAN_POINT('',(56.9121249914169,-85.725,6.8512966632843));
#41906=CARTESIAN_POINT('Ctrl Pts',(58.8029834032059,-85.725,6.84976184368133));
#41907=CARTESIAN_POINT('Ctrl Pts',(58.8029834032059,-85.425,6.84976184368133));
#41908=CARTESIAN_POINT('Ctrl Pts',(58.417752623558,-85.725,6.6732611656189));
#41909=CARTESIAN_POINT('Ctrl Pts',(58.417752623558,-85.425,6.6732611656189));
#41910=CARTESIAN_POINT('Ctrl Pts',(57.9358288049698,-85.725,6.6732611656189));
#41911=CARTESIAN_POINT('Ctrl Pts',(57.9358288049698,-85.425,6.6732611656189));
#41912=CARTESIAN_POINT('',(58.8029834032059,-85.425,6.84976184368133));
#41913=CARTESIAN_POINT('',(58.8029834032059,-85.725,6.84976184368133));
#41914=CARTESIAN_POINT('Ctrl Pts',(58.8029834032059,-85.425,6.84976184368133));
#41915=CARTESIAN_POINT('Ctrl Pts',(58.417752623558,-85.425,6.6732611656189));
#41916=CARTESIAN_POINT('Ctrl Pts',(57.9358288049698,-85.425,6.6732611656189));
#41917=CARTESIAN_POINT('Ctrl Pts',(59.3938776254654,-85.725,7.34396362304687));
#41918=CARTESIAN_POINT('Ctrl Pts',(59.3938776254654,-85.425,7.34396362304687));
#41919=CARTESIAN_POINT('Ctrl Pts',(59.1882153749466,-85.725,7.02626252174377));
#41920=CARTESIAN_POINT('Ctrl Pts',(59.1882153749466,-85.425,7.02626252174377));
#41921=CARTESIAN_POINT('Ctrl Pts',(58.8029834032059,-85.725,6.84976184368133));
#41922=CARTESIAN_POINT('Ctrl Pts',(58.8029834032059,-85.425,6.84976184368133));
#41923=CARTESIAN_POINT('',(59.3938776254654,-85.425,7.34396362304687));
#41924=CARTESIAN_POINT('',(59.3938776254654,-85.725,7.34396362304687));
#41925=CARTESIAN_POINT('Ctrl Pts',(59.3938776254654,-85.425,7.34396362304687));
#41926=CARTESIAN_POINT('Ctrl Pts',(59.1882153749466,-85.425,7.02626252174377));
#41927=CARTESIAN_POINT('Ctrl Pts',(58.8029834032059,-85.425,6.84976184368133));
#41928=CARTESIAN_POINT('Ctrl Pts',(59.5995398759842,-85.725,8.02080535888672));
#41929=CARTESIAN_POINT('Ctrl Pts',(59.5995398759842,-85.425,8.02080535888672));
#41930=CARTESIAN_POINT('Ctrl Pts',(59.5995398759842,-85.725,7.66166472434997));
#41931=CARTESIAN_POINT('Ctrl Pts',(59.5995398759842,-85.425,7.66166472434997));
#41932=CARTESIAN_POINT('Ctrl Pts',(59.3938776254654,-85.725,7.34396362304687));
#41933=CARTESIAN_POINT('Ctrl Pts',(59.3938776254654,-85.425,7.34396362304687));
#41934=CARTESIAN_POINT('',(59.5995398759842,-85.425,8.02080535888672));
#41935=CARTESIAN_POINT('',(59.5995398759842,-85.725,8.02080535888672));
#41936=CARTESIAN_POINT('Ctrl Pts',(59.5995398759842,-85.425,8.02080535888672));
#41937=CARTESIAN_POINT('Ctrl Pts',(59.5995398759842,-85.425,7.66166472434997));
#41938=CARTESIAN_POINT('Ctrl Pts',(59.3938776254654,-85.425,7.34396362304687));
#41939=CARTESIAN_POINT('Ctrl Pts',(59.412295460701,-85.725,8.66081202030182));
#41940=CARTESIAN_POINT('Ctrl Pts',(59.412295460701,-85.425,8.66081202030182));
#41941=CARTESIAN_POINT('Ctrl Pts',(59.5995398759842,-85.725,8.38301503658295));
#41942=CARTESIAN_POINT('Ctrl Pts',(59.5995398759842,-85.425,8.38301503658295));
#41943=CARTESIAN_POINT('Ctrl Pts',(59.5995398759842,-85.725,8.02080535888672));
#41944=CARTESIAN_POINT('Ctrl Pts',(59.5995398759842,-85.425,8.02080535888672));
#41945=CARTESIAN_POINT('',(59.412295460701,-85.425,8.66081202030182));
#41946=CARTESIAN_POINT('',(59.412295460701,-85.725,8.66081202030182));
#41947=CARTESIAN_POINT('Ctrl Pts',(59.412295460701,-85.425,8.66081202030182));
#41948=CARTESIAN_POINT('Ctrl Pts',(59.5995398759842,-85.425,8.38301503658295));
#41949=CARTESIAN_POINT('Ctrl Pts',(59.5995398759842,-85.425,8.02080535888672));
#41950=CARTESIAN_POINT('Ctrl Pts',(58.8321443796158,-85.725,9.11971354484558));
#41951=CARTESIAN_POINT('Ctrl Pts',(58.8321443796158,-85.425,9.11971354484558));
#41952=CARTESIAN_POINT('Ctrl Pts',(59.2250510454178,-85.725,8.93860900402069));
#41953=CARTESIAN_POINT('Ctrl Pts',(59.2250510454178,-85.425,8.93860900402069));
#41954=CARTESIAN_POINT('Ctrl Pts',(59.412295460701,-85.725,8.66081202030182));
#41955=CARTESIAN_POINT('Ctrl Pts',(59.412295460701,-85.425,8.66081202030182));
#41956=CARTESIAN_POINT('',(58.8321443796158,-85.425,9.11971354484558));
#41957=CARTESIAN_POINT('',(58.8321443796158,-85.725,9.11971354484558));
#41958=CARTESIAN_POINT('Ctrl Pts',(58.8321443796158,-85.425,9.11971354484558));
#41959=CARTESIAN_POINT('Ctrl Pts',(59.2250510454178,-85.425,8.93860900402069));
#41960=CARTESIAN_POINT('Ctrl Pts',(59.412295460701,-85.425,8.66081202030182));
#41961=CARTESIAN_POINT('Ctrl Pts',(57.8360673189163,-85.725,9.4067188501358));
#41962=CARTESIAN_POINT('Ctrl Pts',(57.8360673189163,-85.425,9.4067188501358));
#41963=CARTESIAN_POINT('Ctrl Pts',(58.5620220899582,-85.725,9.24249672889709));
#41964=CARTESIAN_POINT('Ctrl Pts',(58.5620220899582,-85.425,9.24249672889709));
#41965=CARTESIAN_POINT('Ctrl Pts',(58.8321443796158,-85.725,9.11971354484558));
#41966=CARTESIAN_POINT('Ctrl Pts',(58.8321443796158,-85.425,9.11971354484558));
#41967=CARTESIAN_POINT('',(57.8360673189163,-85.425,9.4067188501358));
#41968=CARTESIAN_POINT('',(57.8360673189163,-85.725,9.4067188501358));
#41969=CARTESIAN_POINT('Ctrl Pts',(57.8360673189163,-85.425,9.4067188501358));
#41970=CARTESIAN_POINT('Ctrl Pts',(58.5620220899582,-85.425,9.24249672889709));
#41971=CARTESIAN_POINT('Ctrl Pts',(58.8321443796158,-85.425,9.11971354484558));
#41972=CARTESIAN_POINT('Ctrl Pts',(56.9382163286209,-85.725,9.72748959064484));
#41973=CARTESIAN_POINT('Ctrl Pts',(56.9382163286209,-85.425,9.72748959064484));
#41974=CARTESIAN_POINT('Ctrl Pts',(57.1101125478745,-85.725,9.57094156742096));
#41975=CARTESIAN_POINT('Ctrl Pts',(57.1101125478745,-85.425,9.57094156742096));
#41976=CARTESIAN_POINT('Ctrl Pts',(57.8360673189163,-85.725,9.4067188501358));
#41977=CARTESIAN_POINT('Ctrl Pts',(57.8360673189163,-85.425,9.4067188501358));
#41978=CARTESIAN_POINT('',(56.9382163286209,-85.425,9.72748959064484));
#41979=CARTESIAN_POINT('',(56.9382163286209,-85.725,9.72748959064484));
#41980=CARTESIAN_POINT('Ctrl Pts',(56.9382163286209,-85.425,9.72748959064484));
#41981=CARTESIAN_POINT('Ctrl Pts',(57.1101125478745,-85.425,9.57094156742096));
#41982=CARTESIAN_POINT('Ctrl Pts',(57.8360673189163,-85.425,9.4067188501358));
#41983=CARTESIAN_POINT('Ctrl Pts',(56.7632504701614,-85.725,10.1265349388123));
#41984=CARTESIAN_POINT('Ctrl Pts',(56.7632504701614,-85.425,10.1265349388123));
#41985=CARTESIAN_POINT('Ctrl Pts',(56.7632504701614,-85.725,9.88403820991516));
#41986=CARTESIAN_POINT('Ctrl Pts',(56.7632504701614,-85.425,9.88403820991516));
#41987=CARTESIAN_POINT('Ctrl Pts',(56.9382163286209,-85.725,9.72748959064484));
#41988=CARTESIAN_POINT('Ctrl Pts',(56.9382163286209,-85.425,9.72748959064484));
#41989=CARTESIAN_POINT('',(56.7632504701614,-85.425,10.1265349388123));
#41990=CARTESIAN_POINT('',(56.7632504701614,-85.725,10.1265349388123));
#41991=CARTESIAN_POINT('Ctrl Pts',(56.7632504701614,-85.425,10.1265349388123));
#41992=CARTESIAN_POINT('Ctrl Pts',(56.7632504701614,-85.425,9.88403820991516));
#41993=CARTESIAN_POINT('Ctrl Pts',(56.9382163286209,-85.425,9.72748959064484));
#41994=CARTESIAN_POINT('Ctrl Pts',(57.010351061821,-85.725,10.6038540005684));
#41995=CARTESIAN_POINT('Ctrl Pts',(57.010351061821,-85.425,10.6038540005684));
#41996=CARTESIAN_POINT('Ctrl Pts',(56.7632504701614,-85.725,10.4058664441109));
#41997=CARTESIAN_POINT('Ctrl Pts',(56.7632504701614,-85.425,10.4058664441109));
#41998=CARTESIAN_POINT('Ctrl Pts',(56.7632504701614,-85.725,10.1265349388123));
#41999=CARTESIAN_POINT('Ctrl Pts',(56.7632504701614,-85.425,10.1265349388123));
#42000=CARTESIAN_POINT('',(57.010351061821,-85.425,10.6038540005684));
#42001=CARTESIAN_POINT('',(57.010351061821,-85.725,10.6038540005684));
#42002=CARTESIAN_POINT('Ctrl Pts',(57.010351061821,-85.425,10.6038540005684));
#42003=CARTESIAN_POINT('Ctrl Pts',(56.7632504701614,-85.425,10.4058664441109));
#42004=CARTESIAN_POINT('Ctrl Pts',(56.7632504701614,-85.425,10.1265349388123));
#42005=CARTESIAN_POINT('Ctrl Pts',(57.7976974248886,-85.725,10.8018418550491));
#42006=CARTESIAN_POINT('Ctrl Pts',(57.7976974248886,-85.425,10.8018418550491));
#42007=CARTESIAN_POINT('Ctrl Pts',(57.2574516534805,-85.725,10.8018418550491));
#42008=CARTESIAN_POINT('Ctrl Pts',(57.2574516534805,-85.425,10.8018418550491));
#42009=CARTESIAN_POINT('Ctrl Pts',(57.010351061821,-85.725,10.6038540005684));
#42010=CARTESIAN_POINT('Ctrl Pts',(57.010351061821,-85.425,10.6038540005684));
#42011=CARTESIAN_POINT('',(57.7976974248886,-85.425,10.8018418550491));
#42012=CARTESIAN_POINT('',(57.7976974248886,-85.725,10.8018418550491));
#42013=CARTESIAN_POINT('Ctrl Pts',(57.7976974248886,-85.425,10.8018418550491));
#42014=CARTESIAN_POINT('Ctrl Pts',(57.2574516534805,-85.425,10.8018418550491));
#42015=CARTESIAN_POINT('Ctrl Pts',(57.010351061821,-85.425,10.6038540005684));
#42016=CARTESIAN_POINT('Ctrl Pts',(58.5819741487503,-85.725,10.5839019417763));
#42017=CARTESIAN_POINT('Ctrl Pts',(58.5819741487503,-85.425,10.5839019417763));
#42018=CARTESIAN_POINT('Ctrl Pts',(58.3164557218552,-85.725,10.8018418550491));
#42019=CARTESIAN_POINT('Ctrl Pts',(58.3164557218552,-85.425,10.8018418550491));
#42020=CARTESIAN_POINT('Ctrl Pts',(57.7976974248886,-85.725,10.8018418550491));
#42021=CARTESIAN_POINT('Ctrl Pts',(57.7976974248886,-85.425,10.8018418550491));
#42022=CARTESIAN_POINT('',(58.5819741487503,-85.425,10.5839019417763));
#42023=CARTESIAN_POINT('',(58.5819741487503,-85.725,10.5839019417763));
#42024=CARTESIAN_POINT('Ctrl Pts',(58.5819741487503,-85.425,10.5839019417763));
#42025=CARTESIAN_POINT('Ctrl Pts',(58.3164557218552,-85.425,10.8018418550491));
#42026=CARTESIAN_POINT('Ctrl Pts',(57.7976974248886,-85.425,10.8018418550491));
#42027=CARTESIAN_POINT('Ctrl Pts',(58.8935371637344,-85.725,9.9392911195755));
#42028=CARTESIAN_POINT('Ctrl Pts',(58.8935371637344,-85.425,9.9392911195755));
#42029=CARTESIAN_POINT('Ctrl Pts',(58.8474925756454,-85.725,10.3659620285034));
#42030=CARTESIAN_POINT('Ctrl Pts',(58.8474925756454,-85.425,10.3659620285034));
#42031=CARTESIAN_POINT('Ctrl Pts',(58.5819741487503,-85.725,10.5839019417763));
#42032=CARTESIAN_POINT('Ctrl Pts',(58.5819741487503,-85.425,10.5839019417763));
#42033=CARTESIAN_POINT('',(58.8935371637344,-85.425,9.9392911195755));
#42034=CARTESIAN_POINT('',(58.8935371637344,-85.725,9.9392911195755));
#42035=CARTESIAN_POINT('Ctrl Pts',(58.8935371637344,-85.425,9.9392911195755));
#42036=CARTESIAN_POINT('Ctrl Pts',(58.8474925756454,-85.425,10.3659620285034));
#42037=CARTESIAN_POINT('Ctrl Pts',(58.5819741487503,-85.425,10.5839019417763));
#42038=CARTESIAN_POINT('Origin',(59.4644781351089,-85.725,9.98226487636566));
#42039=CARTESIAN_POINT('',(59.4644781351089,-85.425,9.98226487636566));
#42040=CARTESIAN_POINT('',(59.4644781351089,-85.725,9.98226487636566));
#42041=CARTESIAN_POINT('',(59.4644781351089,-85.425,9.98226487636566));
#42042=CARTESIAN_POINT('Ctrl Pts',(59.2434688806534,-85.725,10.6913369297981));
#42043=CARTESIAN_POINT('Ctrl Pts',(59.2434688806534,-85.425,10.6913369297981));
#42044=CARTESIAN_POINT('Ctrl Pts',(59.4491299390793,-85.725,10.3782402873039));
#42045=CARTESIAN_POINT('Ctrl Pts',(59.4491299390793,-85.425,10.3782402873039));
#42046=CARTESIAN_POINT('Ctrl Pts',(59.4644781351089,-85.725,9.98226487636566));
#42047=CARTESIAN_POINT('Ctrl Pts',(59.4644781351089,-85.425,9.98226487636566));
#42048=CARTESIAN_POINT('',(59.2434688806534,-85.425,10.6913369297981));
#42049=CARTESIAN_POINT('',(59.2434688806534,-85.725,10.6913369297981));
#42050=CARTESIAN_POINT('Ctrl Pts',(59.2434688806534,-85.425,10.6913369297981));
#42051=CARTESIAN_POINT('Ctrl Pts',(59.4491299390793,-85.425,10.3782402873039));
#42052=CARTESIAN_POINT('Ctrl Pts',(59.4644781351089,-85.425,9.98226487636566));
#42053=CARTESIAN_POINT('Ctrl Pts',(58.6556442975998,-85.725,11.1655866503716));
#42054=CARTESIAN_POINT('Ctrl Pts',(58.6556442975998,-85.425,11.1655866503716));
#42055=CARTESIAN_POINT('Ctrl Pts',(59.0378066301346,-85.725,11.0044338703156));
#42056=CARTESIAN_POINT('Ctrl Pts',(59.0378066301346,-85.425,11.0044338703156));
#42057=CARTESIAN_POINT('Ctrl Pts',(59.2434688806534,-85.725,10.6913369297981));
#42058=CARTESIAN_POINT('Ctrl Pts',(59.2434688806534,-85.425,10.6913369297981));
#42059=CARTESIAN_POINT('',(58.6556442975998,-85.425,11.1655866503716));
#42060=CARTESIAN_POINT('',(58.6556442975998,-85.725,11.1655866503716));
#42061=CARTESIAN_POINT('Ctrl Pts',(58.6556442975998,-85.425,11.1655866503716));
#42062=CARTESIAN_POINT('Ctrl Pts',(59.0378066301346,-85.425,11.0044338703156));
#42063=CARTESIAN_POINT('Ctrl Pts',(59.2434688806534,-85.425,10.6913369297981));
#42064=CARTESIAN_POINT('Ctrl Pts',(57.773141503334,-85.725,11.3267394304276));
#42065=CARTESIAN_POINT('Ctrl Pts',(57.773141503334,-85.425,11.3267394304276));
#42066=CARTESIAN_POINT('Ctrl Pts',(58.273481965065,-85.725,11.3267394304276));
#42067=CARTESIAN_POINT('Ctrl Pts',(58.273481965065,-85.425,11.3267394304276));
#42068=CARTESIAN_POINT('Ctrl Pts',(58.6556442975998,-85.725,11.1655866503716));
#42069=CARTESIAN_POINT('Ctrl Pts',(58.6556442975998,-85.425,11.1655866503716));
#42070=CARTESIAN_POINT('',(57.773141503334,-85.425,11.3267394304276));
#42071=CARTESIAN_POINT('',(57.773141503334,-85.725,11.3267394304276));
#42072=CARTESIAN_POINT('Ctrl Pts',(57.773141503334,-85.425,11.3267394304276));
#42073=CARTESIAN_POINT('Ctrl Pts',(58.273481965065,-85.425,11.3267394304276));
#42074=CARTESIAN_POINT('Ctrl Pts',(58.6556442975998,-85.425,11.1655866503716));
#42075=CARTESIAN_POINT('Ctrl Pts',(56.9474240541458,-85.725,11.1732607483864));
#42076=CARTESIAN_POINT('Ctrl Pts',(56.9474240541458,-85.425,11.1732607483864));
#42077=CARTESIAN_POINT('Ctrl Pts',(57.3188432455063,-85.725,11.3267394304276));
#42078=CARTESIAN_POINT('Ctrl Pts',(57.3188432455063,-85.425,11.3267394304276));
#42079=CARTESIAN_POINT('Ctrl Pts',(57.773141503334,-85.725,11.3267394304276));
#42080=CARTESIAN_POINT('Ctrl Pts',(57.773141503334,-85.425,11.3267394304276));
#42081=CARTESIAN_POINT('',(56.9474240541458,-85.425,11.1732607483864));
#42082=CARTESIAN_POINT('',(56.9474240541458,-85.725,11.1732607483864));
#42083=CARTESIAN_POINT('Ctrl Pts',(56.9474240541458,-85.425,11.1732607483864));
#42084=CARTESIAN_POINT('Ctrl Pts',(57.3188432455063,-85.425,11.3267394304276));
#42085=CARTESIAN_POINT('Ctrl Pts',(57.773141503334,-85.425,11.3267394304276));
#42086=CARTESIAN_POINT('Ctrl Pts',(56.3826223611832,-85.725,10.723567545414));
#42087=CARTESIAN_POINT('Ctrl Pts',(56.3826223611832,-85.425,10.723567545414));
#42088=CARTESIAN_POINT('Ctrl Pts',(56.5760060548782,-85.725,11.019781768322));
#42089=CARTESIAN_POINT('Ctrl Pts',(56.5760060548782,-85.425,11.019781768322));
#42090=CARTESIAN_POINT('Ctrl Pts',(56.9474240541458,-85.725,11.1732607483864));
#42091=CARTESIAN_POINT('Ctrl Pts',(56.9474240541458,-85.425,11.1732607483864));
#42092=CARTESIAN_POINT('',(56.3826223611832,-85.425,10.723567545414));
#42093=CARTESIAN_POINT('',(56.3826223611832,-85.725,10.723567545414));
#42094=CARTESIAN_POINT('Ctrl Pts',(56.3826223611832,-85.425,10.723567545414));
#42095=CARTESIAN_POINT('Ctrl Pts',(56.5760060548782,-85.425,11.019781768322));
#42096=CARTESIAN_POINT('Ctrl Pts',(56.9474240541458,-85.425,11.1732607483864));
#42097=CARTESIAN_POINT('Ctrl Pts',(56.1892386674881,-85.725,10.0866302251816));
#42098=CARTESIAN_POINT('Ctrl Pts',(56.1892386674881,-85.425,10.0866302251816));
#42099=CARTESIAN_POINT('Ctrl Pts',(56.1892386674881,-85.725,10.427353322506));
#42100=CARTESIAN_POINT('Ctrl Pts',(56.1892386674881,-85.425,10.427353322506));
#42101=CARTESIAN_POINT('Ctrl Pts',(56.3826223611832,-85.725,10.723567545414));
#42102=CARTESIAN_POINT('Ctrl Pts',(56.3826223611832,-85.425,10.723567545414));
#42103=CARTESIAN_POINT('',(56.1892386674881,-85.425,10.0866302251816));
#42104=CARTESIAN_POINT('',(56.1892386674881,-85.725,10.0866302251816));
#42105=CARTESIAN_POINT('Ctrl Pts',(56.1892386674881,-85.425,10.0866302251816));
#42106=CARTESIAN_POINT('Ctrl Pts',(56.1892386674881,-85.425,10.427353322506));
#42107=CARTESIAN_POINT('Ctrl Pts',(56.3826223611832,-85.425,10.723567545414));
#42108=CARTESIAN_POINT('Ctrl Pts',(56.3473221063614,-85.725,9.52643239498138));
#42109=CARTESIAN_POINT('Ctrl Pts',(56.3473221063614,-85.425,9.52643239498138));
#42110=CARTESIAN_POINT('Ctrl Pts',(56.1892386674881,-85.725,9.77660322189331));
#42111=CARTESIAN_POINT('Ctrl Pts',(56.1892386674881,-85.425,9.77660322189331));
#42112=CARTESIAN_POINT('Ctrl Pts',(56.1892386674881,-85.725,10.0866302251816));
#42113=CARTESIAN_POINT('Ctrl Pts',(56.1892386674881,-85.425,10.0866302251816));
#42114=CARTESIAN_POINT('',(56.3473221063614,-85.425,9.52643239498138));
#42115=CARTESIAN_POINT('',(56.3473221063614,-85.725,9.52643239498138));
#42116=CARTESIAN_POINT('Ctrl Pts',(56.3473221063614,-85.425,9.52643239498138));
#42117=CARTESIAN_POINT('Ctrl Pts',(56.1892386674881,-85.425,9.77660322189331));
#42118=CARTESIAN_POINT('Ctrl Pts',(56.1892386674881,-85.425,10.0866302251816));
#42119=CARTESIAN_POINT('Ctrl Pts',(56.8277117013931,-85.725,9.1074355840683));
#42120=CARTESIAN_POINT('Ctrl Pts',(56.8277117013931,-85.425,9.1074355840683));
#42121=CARTESIAN_POINT('Ctrl Pts',(56.5054055452347,-85.725,9.27626216411591));
#42122=CARTESIAN_POINT('Ctrl Pts',(56.5054055452347,-85.425,9.27626216411591));
#42123=CARTESIAN_POINT('Ctrl Pts',(56.3473221063614,-85.725,9.52643239498138));
#42124=CARTESIAN_POINT('Ctrl Pts',(56.3473221063614,-85.425,9.52643239498138));
#42125=CARTESIAN_POINT('',(56.8277117013931,-85.425,9.1074355840683));
#42126=CARTESIAN_POINT('',(56.8277117013931,-85.725,9.1074355840683));
#42127=CARTESIAN_POINT('Ctrl Pts',(56.8277117013931,-85.425,9.1074355840683));
#42128=CARTESIAN_POINT('Ctrl Pts',(56.5054055452347,-85.425,9.27626216411591));
#42129=CARTESIAN_POINT('Ctrl Pts',(56.3473221063614,-85.425,9.52643239498138));
#42130=CARTESIAN_POINT('Ctrl Pts',(57.6964017152786,-85.725,8.82656896114349));
#42131=CARTESIAN_POINT('Ctrl Pts',(57.6964017152786,-85.425,8.82656896114349));
#42132=CARTESIAN_POINT('Ctrl Pts',(57.0763465166092,-85.725,8.97544348239899));
#42133=CARTESIAN_POINT('Ctrl Pts',(57.0763465166092,-85.425,8.97544348239899));
#42134=CARTESIAN_POINT('Ctrl Pts',(56.8277117013931,-85.725,9.1074355840683));
#42135=CARTESIAN_POINT('Ctrl Pts',(56.8277117013931,-85.425,9.1074355840683));
#42136=CARTESIAN_POINT('',(57.6964017152786,-85.425,8.82656896114349));
#42137=CARTESIAN_POINT('',(57.6964017152786,-85.725,8.82656896114349));
#42138=CARTESIAN_POINT('Ctrl Pts',(57.6964017152786,-85.425,8.82656896114349));
#42139=CARTESIAN_POINT('Ctrl Pts',(57.0763465166092,-85.425,8.97544348239899));
#42140=CARTESIAN_POINT('Ctrl Pts',(56.8277117013931,-85.425,9.1074355840683));
#42141=CARTESIAN_POINT('Ctrl Pts',(58.4975608587265,-85.725,8.60709452629089));
#42142=CARTESIAN_POINT('Ctrl Pts',(58.4975608587265,-85.425,8.60709452629089));
#42143=CARTESIAN_POINT('Ctrl Pts',(58.3164557218552,-85.725,8.677694439888));
#42144=CARTESIAN_POINT('Ctrl Pts',(58.3164557218552,-85.425,8.677694439888));
#42145=CARTESIAN_POINT('Ctrl Pts',(57.6964017152786,-85.725,8.82656896114349));
#42146=CARTESIAN_POINT('Ctrl Pts',(57.6964017152786,-85.425,8.82656896114349));
#42147=CARTESIAN_POINT('',(58.4975608587265,-85.425,8.60709452629089));
#42148=CARTESIAN_POINT('',(58.4975608587265,-85.725,8.60709452629089));
#42149=CARTESIAN_POINT('Ctrl Pts',(58.4975608587265,-85.425,8.60709452629089));
#42150=CARTESIAN_POINT('Ctrl Pts',(58.3164557218552,-85.425,8.677694439888));
#42151=CARTESIAN_POINT('Ctrl Pts',(57.6964017152786,-85.425,8.82656896114349));
#42152=CARTESIAN_POINT('Ctrl Pts',(58.9027448892593,-85.725,8.34157609939575));
#42153=CARTESIAN_POINT('Ctrl Pts',(58.9027448892593,-85.425,8.34157609939575));
#42154=CARTESIAN_POINT('Ctrl Pts',(58.7799617052078,-85.725,8.4996589422226));
#42155=CARTESIAN_POINT('Ctrl Pts',(58.7799617052078,-85.425,8.4996589422226));
#42156=CARTESIAN_POINT('Ctrl Pts',(58.4975608587265,-85.725,8.60709452629089));
#42157=CARTESIAN_POINT('Ctrl Pts',(58.4975608587265,-85.425,8.60709452629089));
#42158=CARTESIAN_POINT('',(58.9027448892593,-85.425,8.34157609939575));
#42159=CARTESIAN_POINT('',(58.9027448892593,-85.725,8.34157609939575));
#42160=CARTESIAN_POINT('Ctrl Pts',(58.9027448892593,-85.425,8.34157609939575));
#42161=CARTESIAN_POINT('Ctrl Pts',(58.7799617052078,-85.425,8.4996589422226));
#42162=CARTESIAN_POINT('Ctrl Pts',(58.4975608587265,-85.425,8.60709452629089));
#42163=CARTESIAN_POINT('Ctrl Pts',(59.0255280733109,-85.725,7.97169172763824));
#42164=CARTESIAN_POINT('Ctrl Pts',(59.0255280733109,-85.425,7.97169172763824));
#42165=CARTESIAN_POINT('Ctrl Pts',(59.0255280733109,-85.725,8.18349266052246));
#42166=CARTESIAN_POINT('Ctrl Pts',(59.0255280733109,-85.425,8.18349266052246));
#42167=CARTESIAN_POINT('Ctrl Pts',(58.9027448892593,-85.725,8.34157609939575));
#42168=CARTESIAN_POINT('Ctrl Pts',(58.9027448892593,-85.425,8.34157609939575));
#42169=CARTESIAN_POINT('',(59.0255280733109,-85.425,7.97169172763824));
#42170=CARTESIAN_POINT('',(59.0255280733109,-85.725,7.97169172763824));
#42171=CARTESIAN_POINT('Ctrl Pts',(59.0255280733109,-85.425,7.97169172763824));
#42172=CARTESIAN_POINT('Ctrl Pts',(59.0255280733109,-85.425,8.18349266052246));
#42173=CARTESIAN_POINT('Ctrl Pts',(58.9027448892593,-85.425,8.34157609939575));
#42174=CARTESIAN_POINT('Ctrl Pts',(58.8981410264969,-85.725,7.58645975589752));
#42175=CARTESIAN_POINT('Ctrl Pts',(58.8981410264969,-85.425,7.58645975589752));
#42176=CARTESIAN_POINT('Ctrl Pts',(59.0255280733109,-85.725,7.76296103000641));
#42177=CARTESIAN_POINT('Ctrl Pts',(59.0255280733109,-85.425,7.76296103000641));
#42178=CARTESIAN_POINT('Ctrl Pts',(59.0255280733109,-85.725,7.97169172763824));
#42179=CARTESIAN_POINT('Ctrl Pts',(59.0255280733109,-85.425,7.97169172763824));
#42180=CARTESIAN_POINT('',(58.8981410264969,-85.425,7.58645975589752));
#42181=CARTESIAN_POINT('',(58.8981410264969,-85.725,7.58645975589752));
#42182=CARTESIAN_POINT('Ctrl Pts',(58.8981410264969,-85.425,7.58645975589752));
#42183=CARTESIAN_POINT('Ctrl Pts',(59.0255280733109,-85.425,7.76296103000641));
#42184=CARTESIAN_POINT('Ctrl Pts',(59.0255280733109,-85.425,7.97169172763824));
#42185=CARTESIAN_POINT('Ctrl Pts',(58.5098394155502,-85.725,7.3086633682251));
#42186=CARTESIAN_POINT('Ctrl Pts',(58.5098394155502,-85.425,7.3086633682251));
#42187=CARTESIAN_POINT('Ctrl Pts',(58.7707539796829,-85.725,7.40995967388153));
#42188=CARTESIAN_POINT('Ctrl Pts',(58.7707539796829,-85.425,7.40995967388153));
#42189=CARTESIAN_POINT('Ctrl Pts',(58.8981410264969,-85.725,7.58645975589752));
#42190=CARTESIAN_POINT('Ctrl Pts',(58.8981410264969,-85.425,7.58645975589752));
#42191=CARTESIAN_POINT('',(58.5098394155502,-85.425,7.3086633682251));
#42192=CARTESIAN_POINT('',(58.5098394155502,-85.725,7.3086633682251));
#42193=CARTESIAN_POINT('Ctrl Pts',(58.5098394155502,-85.425,7.3086633682251));
#42194=CARTESIAN_POINT('Ctrl Pts',(58.7707539796829,-85.425,7.40995967388153));
#42195=CARTESIAN_POINT('Ctrl Pts',(58.8981410264969,-85.425,7.58645975589752));
#42196=CARTESIAN_POINT('Ctrl Pts',(57.9082020521164,-85.725,7.20736706256866));
#42197=CARTESIAN_POINT('Ctrl Pts',(57.9082020521164,-85.425,7.20736706256866));
#42198=CARTESIAN_POINT('Ctrl Pts',(58.2489248514175,-85.725,7.20736706256866));
#42199=CARTESIAN_POINT('Ctrl Pts',(58.2489248514175,-85.425,7.20736706256866));
#42200=CARTESIAN_POINT('Ctrl Pts',(58.5098394155502,-85.725,7.3086633682251));
#42201=CARTESIAN_POINT('Ctrl Pts',(58.5098394155502,-85.425,7.3086633682251));
#42202=CARTESIAN_POINT('',(57.9082020521164,-85.425,7.20736706256866));
#42203=CARTESIAN_POINT('',(57.9082020521164,-85.725,7.20736706256866));
#42204=CARTESIAN_POINT('Ctrl Pts',(57.9082020521164,-85.425,7.20736706256866));
#42205=CARTESIAN_POINT('Ctrl Pts',(58.2489248514175,-85.425,7.20736706256866));
#42206=CARTESIAN_POINT('Ctrl Pts',(58.5098394155502,-85.425,7.3086633682251));
#42207=CARTESIAN_POINT('Ctrl Pts',(57.2175475358963,-85.725,7.34089398384094));
#42208=CARTESIAN_POINT('Ctrl Pts',(57.2175475358963,-85.425,7.34089398384094));
#42209=CARTESIAN_POINT('Ctrl Pts',(57.5245054960251,-85.725,7.20736706256866));
#42210=CARTESIAN_POINT('Ctrl Pts',(57.5245054960251,-85.425,7.20736706256866));
#42211=CARTESIAN_POINT('Ctrl Pts',(57.9082020521164,-85.725,7.20736706256866));
#42212=CARTESIAN_POINT('Ctrl Pts',(57.9082020521164,-85.425,7.20736706256866));
#42213=CARTESIAN_POINT('',(57.2175475358963,-85.425,7.34089398384094));
#42214=CARTESIAN_POINT('',(57.2175475358963,-85.725,7.34089398384094));
#42215=CARTESIAN_POINT('Ctrl Pts',(57.2175475358963,-85.425,7.34089398384094));
#42216=CARTESIAN_POINT('Ctrl Pts',(57.5245054960251,-85.425,7.20736706256866));
#42217=CARTESIAN_POINT('Ctrl Pts',(57.9082020521164,-85.425,7.20736706256866));
#42218=CARTESIAN_POINT('Ctrl Pts',(56.764784693718,-85.725,7.69082570075989));
#42219=CARTESIAN_POINT('Ctrl Pts',(56.764784693718,-85.425,7.69082570075989));
#42220=CARTESIAN_POINT('Ctrl Pts',(56.9105907678604,-85.725,7.47442030906677));
#42221=CARTESIAN_POINT('Ctrl Pts',(56.9105907678604,-85.425,7.47442030906677));
#42222=CARTESIAN_POINT('Ctrl Pts',(57.2175475358963,-85.725,7.34089398384094));
#42223=CARTESIAN_POINT('Ctrl Pts',(57.2175475358963,-85.425,7.34089398384094));
#42224=CARTESIAN_POINT('',(56.764784693718,-85.425,7.69082570075989));
#42225=CARTESIAN_POINT('',(56.764784693718,-85.725,7.69082570075989));
#42226=CARTESIAN_POINT('Ctrl Pts',(56.764784693718,-85.425,7.69082570075989));
#42227=CARTESIAN_POINT('Ctrl Pts',(56.9105907678604,-85.425,7.47442030906677));
#42228=CARTESIAN_POINT('Ctrl Pts',(57.2175475358963,-85.425,7.34089398384094));
#42229=CARTESIAN_POINT('Ctrl Pts',(56.5790756940842,-85.725,8.24488425254822));
#42230=CARTESIAN_POINT('Ctrl Pts',(56.5790756940842,-85.425,8.24488425254822));
#42231=CARTESIAN_POINT('Ctrl Pts',(56.6189798116684,-85.725,7.907231092453));
#42232=CARTESIAN_POINT('Ctrl Pts',(56.6189798116684,-85.425,7.907231092453));
#42233=CARTESIAN_POINT('Ctrl Pts',(56.764784693718,-85.725,7.69082570075989));
#42234=CARTESIAN_POINT('Ctrl Pts',(56.764784693718,-85.425,7.69082570075989));
#42235=CARTESIAN_POINT('',(56.5790756940842,-85.425,8.24488425254822));
#42236=CARTESIAN_POINT('',(56.5790756940842,-85.725,8.24488425254822));
#42237=CARTESIAN_POINT('Ctrl Pts',(56.5790756940842,-85.425,8.24488425254822));
#42238=CARTESIAN_POINT('Ctrl Pts',(56.6189798116684,-85.425,7.907231092453));
#42239=CARTESIAN_POINT('Ctrl Pts',(56.764784693718,-85.425,7.69082570075989));
#42240=CARTESIAN_POINT('Origin',(56.0173436403275,-85.725,8.19577121734619));
#42241=CARTESIAN_POINT('',(56.0173436403275,-85.425,8.19577121734619));
#42242=CARTESIAN_POINT('',(56.0173436403275,-85.725,8.19577121734619));
#42243=CARTESIAN_POINT('',(56.0173436403275,-85.425,8.19577121734619));
#42244=CARTESIAN_POINT('Ctrl Pts',(56.264444231987,-85.725,7.38693737983704));
#42245=CARTESIAN_POINT('Ctrl Pts',(56.264444231987,-85.425,7.38693737983704));
#42246=CARTESIAN_POINT('Ctrl Pts',(56.0296221971512,-85.725,7.74454319477081));
#42247=CARTESIAN_POINT('Ctrl Pts',(56.0296221971512,-85.425,7.74454319477081));
#42248=CARTESIAN_POINT('Ctrl Pts',(56.0173436403275,-85.725,8.19577121734619));
#42249=CARTESIAN_POINT('Ctrl Pts',(56.0173436403275,-85.425,8.19577121734619));
#42250=CARTESIAN_POINT('',(56.264444231987,-85.425,7.38693737983704));
#42251=CARTESIAN_POINT('',(56.264444231987,-85.725,7.38693737983704));
#42252=CARTESIAN_POINT('Ctrl Pts',(56.264444231987,-85.425,7.38693737983704));
#42253=CARTESIAN_POINT('Ctrl Pts',(56.0296221971512,-85.425,7.74454319477081));
#42254=CARTESIAN_POINT('Ctrl Pts',(56.0173436403275,-85.425,8.19577121734619));
#42255=CARTESIAN_POINT('Ctrl Pts',(56.9121249914169,-85.725,6.8512966632843));
#42256=CARTESIAN_POINT('Ctrl Pts',(56.9121249914169,-85.425,6.8512966632843));
#42257=CARTESIAN_POINT('Ctrl Pts',(56.4992662668228,-85.725,7.02933156490326));
#42258=CARTESIAN_POINT('Ctrl Pts',(56.4992662668228,-85.425,7.02933156490326));
#42259=CARTESIAN_POINT('Ctrl Pts',(56.264444231987,-85.725,7.38693737983704));
#42260=CARTESIAN_POINT('Ctrl Pts',(56.264444231987,-85.425,7.38693737983704));
#42261=CARTESIAN_POINT('Ctrl Pts',(56.9121249914169,-85.425,6.8512966632843));
#42262=CARTESIAN_POINT('Ctrl Pts',(56.4992662668228,-85.425,7.02933156490326));
#42263=CARTESIAN_POINT('Ctrl Pts',(56.264444231987,-85.425,7.38693737983704));
#42264=CARTESIAN_POINT('Origin',(57.8084417581558,-85.425,9.00000029802322));
#42265=CARTESIAN_POINT('Ctrl Pts',(49.7768934965134,-85.725,7.0799800157547));
#42266=CARTESIAN_POINT('Ctrl Pts',(49.7768934965134,-85.425,7.0799800157547));
#42267=CARTESIAN_POINT('Ctrl Pts',(49.3471523523331,-85.725,6.67019152641296));
#42268=CARTESIAN_POINT('Ctrl Pts',(49.3471523523331,-85.425,6.67019152641296));
#42269=CARTESIAN_POINT('Ctrl Pts',(48.6902626752853,-85.725,6.67019152641296));
#42270=CARTESIAN_POINT('Ctrl Pts',(48.6902626752853,-85.425,6.67019152641296));
#42271=CARTESIAN_POINT('',(49.7768934965134,-85.425,7.0799800157547));
#42272=CARTESIAN_POINT('',(49.7768934965134,-85.725,7.0799800157547));
#42273=CARTESIAN_POINT('',(48.6902626752853,-85.425,6.67019152641296));
#42274=CARTESIAN_POINT('Ctrl Pts',(49.7768934965134,-85.425,7.0799800157547));
#42275=CARTESIAN_POINT('Ctrl Pts',(49.3471523523331,-85.425,6.67019152641296));
#42276=CARTESIAN_POINT('Ctrl Pts',(48.6902626752853,-85.425,6.67019152641296));
#42277=CARTESIAN_POINT('',(48.6902626752853,-85.725,6.67019152641296));
#42278=CARTESIAN_POINT('Ctrl Pts',(50.2066334486008,-85.725,8.07912731170654));
#42279=CARTESIAN_POINT('Ctrl Pts',(50.2066334486008,-85.425,8.07912731170654));
#42280=CARTESIAN_POINT('Ctrl Pts',(50.2066334486008,-85.725,7.48976850509643));
#42281=CARTESIAN_POINT('Ctrl Pts',(50.2066334486008,-85.425,7.48976850509643));
#42282=CARTESIAN_POINT('Ctrl Pts',(49.7768934965134,-85.725,7.0799800157547));
#42283=CARTESIAN_POINT('Ctrl Pts',(49.7768934965134,-85.425,7.0799800157547));
#42284=CARTESIAN_POINT('',(50.2066334486008,-85.425,8.07912731170654));
#42285=CARTESIAN_POINT('',(50.2066334486008,-85.725,8.07912731170654));
#42286=CARTESIAN_POINT('Ctrl Pts',(50.2066334486008,-85.425,8.07912731170654));
#42287=CARTESIAN_POINT('Ctrl Pts',(50.2066334486008,-85.425,7.48976850509643));
#42288=CARTESIAN_POINT('Ctrl Pts',(49.7768934965134,-85.425,7.0799800157547));
#42289=CARTESIAN_POINT('Ctrl Pts',(49.9856241941452,-85.725,8.80508208274841));
#42290=CARTESIAN_POINT('Ctrl Pts',(49.9856241941452,-85.425,8.80508208274841));
#42291=CARTESIAN_POINT('Ctrl Pts',(50.2066334486008,-85.725,8.51500713825226));
#42292=CARTESIAN_POINT('Ctrl Pts',(50.2066334486008,-85.425,8.51500713825226));
#42293=CARTESIAN_POINT('Ctrl Pts',(50.2066334486008,-85.725,8.07912731170654));
#42294=CARTESIAN_POINT('Ctrl Pts',(50.2066334486008,-85.425,8.07912731170654));
#42295=CARTESIAN_POINT('',(49.9856241941452,-85.425,8.80508208274841));
#42296=CARTESIAN_POINT('',(49.9856241941452,-85.725,8.80508208274841));
#42297=CARTESIAN_POINT('Ctrl Pts',(49.9856241941452,-85.425,8.80508208274841));
#42298=CARTESIAN_POINT('Ctrl Pts',(50.2066334486008,-85.425,8.51500713825226));
#42299=CARTESIAN_POINT('Ctrl Pts',(50.2066334486008,-85.425,8.07912731170654));
#42300=CARTESIAN_POINT('Ctrl Pts',(49.3655695915222,-85.725,9.1872444152832));
#42301=CARTESIAN_POINT('Ctrl Pts',(49.3655695915222,-85.425,9.1872444152832));
#42302=CARTESIAN_POINT('Ctrl Pts',(49.7646149396896,-85.725,9.09515702724457));
#42303=CARTESIAN_POINT('Ctrl Pts',(49.7646149396896,-85.425,9.09515702724457));
#42304=CARTESIAN_POINT('Ctrl Pts',(49.9856241941452,-85.725,8.80508208274841));
#42305=CARTESIAN_POINT('Ctrl Pts',(49.9856241941452,-85.425,8.80508208274841));
#42306=CARTESIAN_POINT('',(49.3655695915222,-85.425,9.1872444152832));
#42307=CARTESIAN_POINT('',(49.3655695915222,-85.725,9.1872444152832));
#42308=CARTESIAN_POINT('Ctrl Pts',(49.3655695915222,-85.425,9.1872444152832));
#42309=CARTESIAN_POINT('Ctrl Pts',(49.7646149396896,-85.425,9.09515702724457));
#42310=CARTESIAN_POINT('Ctrl Pts',(49.9856241941452,-85.425,8.80508208274841));
#42311=CARTESIAN_POINT('Ctrl Pts',(49.8290761709213,-85.725,9.56787192821503));
#42312=CARTESIAN_POINT('Ctrl Pts',(49.8290761709213,-85.425,9.56787192821503));
#42313=CARTESIAN_POINT('Ctrl Pts',(49.672527551651,-85.725,9.32844483852386));
#42314=CARTESIAN_POINT('Ctrl Pts',(49.672527551651,-85.425,9.32844483852386));
#42315=CARTESIAN_POINT('Ctrl Pts',(49.3655695915222,-85.725,9.1872444152832));
#42316=CARTESIAN_POINT('Ctrl Pts',(49.3655695915222,-85.425,9.1872444152832));
#42317=CARTESIAN_POINT('',(49.8290761709213,-85.425,9.56787192821503));
#42318=CARTESIAN_POINT('',(49.8290761709213,-85.725,9.56787192821503));
#42319=CARTESIAN_POINT('Ctrl Pts',(49.8290761709213,-85.425,9.56787192821503));
#42320=CARTESIAN_POINT('Ctrl Pts',(49.672527551651,-85.425,9.32844483852386));
#42321=CARTESIAN_POINT('Ctrl Pts',(49.3655695915222,-85.425,9.1872444152832));
#42322=CARTESIAN_POINT('Ctrl Pts',(49.9856241941452,-85.725,10.0989087820053));
#42323=CARTESIAN_POINT('Ctrl Pts',(49.9856241941452,-85.425,10.0989087820053));
#42324=CARTESIAN_POINT('Ctrl Pts',(49.9856241941452,-85.725,9.80729901790619));
#42325=CARTESIAN_POINT('Ctrl Pts',(49.9856241941452,-85.425,9.80729901790619));
#42326=CARTESIAN_POINT('Ctrl Pts',(49.8290761709213,-85.725,9.56787192821503));
#42327=CARTESIAN_POINT('Ctrl Pts',(49.8290761709213,-85.425,9.56787192821503));
#42328=CARTESIAN_POINT('',(49.9856241941452,-85.425,10.0989087820053));
#42329=CARTESIAN_POINT('',(49.9856241941452,-85.725,10.0989087820053));
#42330=CARTESIAN_POINT('Ctrl Pts',(49.9856241941452,-85.425,10.0989087820053));
#42331=CARTESIAN_POINT('Ctrl Pts',(49.9856241941452,-85.425,9.80729901790619));
#42332=CARTESIAN_POINT('Ctrl Pts',(49.8290761709213,-85.425,9.56787192821503));
#42333=CARTESIAN_POINT('Ctrl Pts',(49.8214020729065,-85.725,10.6790586709976));
#42334=CARTESIAN_POINT('Ctrl Pts',(49.8214020729065,-85.425,10.6790586709976));
#42335=CARTESIAN_POINT('Ctrl Pts',(49.9856241941452,-85.725,10.4058664441109));
#42336=CARTESIAN_POINT('Ctrl Pts',(49.9856241941452,-85.425,10.4058664441109));
#42337=CARTESIAN_POINT('Ctrl Pts',(49.9856241941452,-85.725,10.0989087820053));
#42338=CARTESIAN_POINT('Ctrl Pts',(49.9856241941452,-85.425,10.0989087820053));
#42339=CARTESIAN_POINT('',(49.8214020729065,-85.425,10.6790586709976));
#42340=CARTESIAN_POINT('',(49.8214020729065,-85.725,10.6790586709976));
#42341=CARTESIAN_POINT('Ctrl Pts',(49.8214020729065,-85.425,10.6790586709976));
#42342=CARTESIAN_POINT('Ctrl Pts',(49.9856241941452,-85.425,10.4058664441109));
#42343=CARTESIAN_POINT('Ctrl Pts',(49.9856241941452,-85.425,10.0989087820053));
#42344=CARTESIAN_POINT('Ctrl Pts',(49.3471523523331,-85.725,11.1103343367577));
#42345=CARTESIAN_POINT('Ctrl Pts',(49.3471523523331,-85.425,11.1103343367577));
#42346=CARTESIAN_POINT('Ctrl Pts',(49.6571799516678,-85.725,10.9522508978844));
#42347=CARTESIAN_POINT('Ctrl Pts',(49.6571799516678,-85.425,10.9522508978844));
#42348=CARTESIAN_POINT('Ctrl Pts',(49.8214020729065,-85.725,10.6790586709976));
#42349=CARTESIAN_POINT('Ctrl Pts',(49.8214020729065,-85.425,10.6790586709976));
#42350=CARTESIAN_POINT('',(49.3471523523331,-85.425,11.1103343367577));
#42351=CARTESIAN_POINT('',(49.3471523523331,-85.725,11.1103343367577));
#42352=CARTESIAN_POINT('Ctrl Pts',(49.3471523523331,-85.425,11.1103343367577));
#42353=CARTESIAN_POINT('Ctrl Pts',(49.6571799516678,-85.425,10.9522508978844));
#42354=CARTESIAN_POINT('Ctrl Pts',(49.8214020729065,-85.425,10.6790586709976));
#42355=CARTESIAN_POINT('Ctrl Pts',(48.6687757968903,-85.725,11.2684174776077));
#42356=CARTESIAN_POINT('Ctrl Pts',(48.6687757968903,-85.425,11.2684174776077));
#42357=CARTESIAN_POINT('Ctrl Pts',(49.0371247529984,-85.725,11.2684174776077));
#42358=CARTESIAN_POINT('Ctrl Pts',(49.0371247529984,-85.425,11.2684174776077));
#42359=CARTESIAN_POINT('Ctrl Pts',(49.3471523523331,-85.725,11.1103343367577));
#42360=CARTESIAN_POINT('Ctrl Pts',(49.3471523523331,-85.425,11.1103343367577));
#42361=CARTESIAN_POINT('',(48.6687757968903,-85.425,11.2684174776077));
#42362=CARTESIAN_POINT('',(48.6687757968903,-85.725,11.2684174776077));
#42363=CARTESIAN_POINT('Ctrl Pts',(48.6687757968903,-85.425,11.2684174776077));
#42364=CARTESIAN_POINT('Ctrl Pts',(49.0371247529984,-85.425,11.2684174776077));
#42365=CARTESIAN_POINT('Ctrl Pts',(49.3471523523331,-85.425,11.1103343367577));
#42366=CARTESIAN_POINT('Ctrl Pts',(47.7755289673805,-85.725,10.9629946351051));
#42367=CARTESIAN_POINT('Ctrl Pts',(47.7755289673805,-85.425,10.9629946351051));
#42368=CARTESIAN_POINT('Ctrl Pts',(48.134669303894,-85.725,11.2684174776077));
#42369=CARTESIAN_POINT('Ctrl Pts',(48.134669303894,-85.425,11.2684174776077));
#42370=CARTESIAN_POINT('Ctrl Pts',(48.6687757968903,-85.725,11.2684174776077));
#42371=CARTESIAN_POINT('Ctrl Pts',(48.6687757968903,-85.425,11.2684174776077));
#42372=CARTESIAN_POINT('',(47.7755289673805,-85.425,10.9629946351051));
#42373=CARTESIAN_POINT('',(47.7755289673805,-85.725,10.9629946351051));
#42374=CARTESIAN_POINT('Ctrl Pts',(47.7755289673805,-85.425,10.9629946351051));
#42375=CARTESIAN_POINT('Ctrl Pts',(48.134669303894,-85.425,11.2684174776077));
#42376=CARTESIAN_POINT('Ctrl Pts',(48.6687757968903,-85.425,11.2684174776077));
#42377=CARTESIAN_POINT('Ctrl Pts',(47.3150923252106,-85.725,10.1019784212112));
#42378=CARTESIAN_POINT('Ctrl Pts',(47.3150923252106,-85.425,10.1019784212112));
#42379=CARTESIAN_POINT('Ctrl Pts',(47.4163883328438,-85.725,10.6575717926025));
#42380=CARTESIAN_POINT('Ctrl Pts',(47.4163883328438,-85.425,10.6575717926025));
#42381=CARTESIAN_POINT('Ctrl Pts',(47.7755289673805,-85.725,10.9629946351051));
#42382=CARTESIAN_POINT('Ctrl Pts',(47.7755289673805,-85.425,10.9629946351051));
#42383=CARTESIAN_POINT('',(47.3150923252106,-85.425,10.1019784212112));
#42384=CARTESIAN_POINT('',(47.3150923252106,-85.725,10.1019784212112));
#42385=CARTESIAN_POINT('Ctrl Pts',(47.3150923252106,-85.425,10.1019784212112));
#42386=CARTESIAN_POINT('Ctrl Pts',(47.4163883328438,-85.425,10.6575717926025));
#42387=CARTESIAN_POINT('Ctrl Pts',(47.7755289673805,-85.425,10.9629946351051));
#42388=CARTESIAN_POINT('Origin',(47.8676160573959,-85.725,10.0037517547607));
#42389=CARTESIAN_POINT('',(47.8676160573959,-85.425,10.0037517547607));
#42390=CARTESIAN_POINT('',(47.8676160573959,-85.725,10.0037517547607));
#42391=CARTESIAN_POINT('',(47.8676160573959,-85.425,10.0037517547607));
#42392=CARTESIAN_POINT('Ctrl Pts',(48.1438782215118,-85.725,10.6115280985832));
#42393=CARTESIAN_POINT('Ctrl Pts',(48.1438782215118,-85.425,10.6115280985832));
#42394=CARTESIAN_POINT('Ctrl Pts',(47.9290076494217,-85.725,10.4089357852936));
#42395=CARTESIAN_POINT('Ctrl Pts',(47.9290076494217,-85.425,10.4089357852936));
#42396=CARTESIAN_POINT('Ctrl Pts',(47.8676160573959,-85.725,10.0037517547607));
#42397=CARTESIAN_POINT('Ctrl Pts',(47.8676160573959,-85.425,10.0037517547607));
#42398=CARTESIAN_POINT('',(48.1438782215118,-85.425,10.6115280985832));
#42399=CARTESIAN_POINT('',(48.1438782215118,-85.725,10.6115280985832));
#42400=CARTESIAN_POINT('Ctrl Pts',(48.1438782215118,-85.425,10.6115280985832));
#42401=CARTESIAN_POINT('Ctrl Pts',(47.9290076494217,-85.425,10.4089357852936));
#42402=CARTESIAN_POINT('Ctrl Pts',(47.8676160573959,-85.425,10.0037517547607));
#42403=CARTESIAN_POINT('Ctrl Pts',(48.6810540556908,-85.725,10.8141201138496));
#42404=CARTESIAN_POINT('Ctrl Pts',(48.6810540556908,-85.425,10.8141201138496));
#42405=CARTESIAN_POINT('Ctrl Pts',(48.3587484955788,-85.725,10.8141201138496));
#42406=CARTESIAN_POINT('Ctrl Pts',(48.3587484955788,-85.425,10.8141201138496));
#42407=CARTESIAN_POINT('Ctrl Pts',(48.1438782215118,-85.725,10.6115280985832));
#42408=CARTESIAN_POINT('Ctrl Pts',(48.1438782215118,-85.425,10.6115280985832));
#42409=CARTESIAN_POINT('',(48.6810540556908,-85.425,10.8141201138496));
#42410=CARTESIAN_POINT('',(48.6810540556908,-85.725,10.8141201138496));
#42411=CARTESIAN_POINT('Ctrl Pts',(48.6810540556908,-85.425,10.8141201138496));
#42412=CARTESIAN_POINT('Ctrl Pts',(48.3587484955788,-85.425,10.8141201138496));
#42413=CARTESIAN_POINT('Ctrl Pts',(48.1438782215118,-85.425,10.6115280985832));
#42414=CARTESIAN_POINT('Ctrl Pts',(49.2120906114578,-85.725,10.6145974397659));
#42415=CARTESIAN_POINT('Ctrl Pts',(49.2120906114578,-85.425,10.6145974397659));
#42416=CARTESIAN_POINT('Ctrl Pts',(49.0064295530319,-85.725,10.8141201138496));
#42417=CARTESIAN_POINT('Ctrl Pts',(49.0064295530319,-85.425,10.8141201138496));
#42418=CARTESIAN_POINT('Ctrl Pts',(48.6810540556908,-85.725,10.8141201138496));
#42419=CARTESIAN_POINT('Ctrl Pts',(48.6810540556908,-85.425,10.8141201138496));
#42420=CARTESIAN_POINT('',(49.2120906114578,-85.425,10.6145974397659));
#42421=CARTESIAN_POINT('',(49.2120906114578,-85.725,10.6145974397659));
#42422=CARTESIAN_POINT('Ctrl Pts',(49.2120906114578,-85.425,10.6145974397659));
#42423=CARTESIAN_POINT('Ctrl Pts',(49.0064295530319,-85.425,10.8141201138496));
#42424=CARTESIAN_POINT('Ctrl Pts',(48.6810540556908,-85.425,10.8141201138496));
#42425=CARTESIAN_POINT('Ctrl Pts',(49.4177528619766,-85.725,10.111187338829));
#42426=CARTESIAN_POINT('Ctrl Pts',(49.4177528619766,-85.425,10.111187338829));
#42427=CARTESIAN_POINT('Ctrl Pts',(49.4177528619766,-85.725,10.4150750637054));
#42428=CARTESIAN_POINT('Ctrl Pts',(49.4177528619766,-85.425,10.4150750637054));
#42429=CARTESIAN_POINT('Ctrl Pts',(49.2120906114578,-85.725,10.6145974397659));
#42430=CARTESIAN_POINT('Ctrl Pts',(49.2120906114578,-85.425,10.6145974397659));
#42431=CARTESIAN_POINT('',(49.4177528619766,-85.425,10.111187338829));
#42432=CARTESIAN_POINT('',(49.4177528619766,-85.725,10.111187338829));
#42433=CARTESIAN_POINT('Ctrl Pts',(49.4177528619766,-85.425,10.111187338829));
#42434=CARTESIAN_POINT('Ctrl Pts',(49.4177528619766,-85.425,10.4150750637054));
#42435=CARTESIAN_POINT('Ctrl Pts',(49.2120906114578,-85.425,10.6145974397659));
#42436=CARTESIAN_POINT('Ctrl Pts',(49.1353514194489,-85.725,9.54331481456757));
#42437=CARTESIAN_POINT('Ctrl Pts',(49.1353514194489,-85.425,9.54331481456757));
#42438=CARTESIAN_POINT('Ctrl Pts',(49.4177528619766,-85.725,9.72748959064484));
#42439=CARTESIAN_POINT('Ctrl Pts',(49.4177528619766,-85.425,9.72748959064484));
#42440=CARTESIAN_POINT('Ctrl Pts',(49.4177528619766,-85.725,10.111187338829));
#42441=CARTESIAN_POINT('Ctrl Pts',(49.4177528619766,-85.425,10.111187338829));
#42442=CARTESIAN_POINT('',(49.1353514194489,-85.425,9.54331481456757));
#42443=CARTESIAN_POINT('',(49.1353514194489,-85.725,9.54331481456757));
#42444=CARTESIAN_POINT('Ctrl Pts',(49.1353514194489,-85.425,9.54331481456757));
#42445=CARTESIAN_POINT('Ctrl Pts',(49.4177528619766,-85.425,9.72748959064484));
#42446=CARTESIAN_POINT('Ctrl Pts',(49.4177528619766,-85.425,10.111187338829));
#42447=CARTESIAN_POINT('Ctrl Pts',(48.4999492168427,-85.725,9.35914063453674));
#42448=CARTESIAN_POINT('Ctrl Pts',(48.4999492168427,-85.425,9.35914063453674));
#42449=CARTESIAN_POINT('Ctrl Pts',(48.8529505729675,-85.725,9.35914063453674));
#42450=CARTESIAN_POINT('Ctrl Pts',(48.8529505729675,-85.425,9.35914063453674));
#42451=CARTESIAN_POINT('Ctrl Pts',(49.1353514194489,-85.725,9.54331481456757));
#42452=CARTESIAN_POINT('Ctrl Pts',(49.1353514194489,-85.425,9.54331481456757));
#42453=CARTESIAN_POINT('',(48.4999492168427,-85.425,9.35914063453674));
#42454=CARTESIAN_POINT('',(48.4999492168427,-85.725,9.35914063453674));
#42455=CARTESIAN_POINT('Ctrl Pts',(48.4999492168427,-85.425,9.35914063453674));
#42456=CARTESIAN_POINT('Ctrl Pts',(48.8529505729675,-85.425,9.35914063453674));
#42457=CARTESIAN_POINT('Ctrl Pts',(49.1353514194489,-85.425,9.54331481456757));
#42458=CARTESIAN_POINT('Ctrl Pts',(48.4109314680099,-85.725,9.36527991294861));
#42459=CARTESIAN_POINT('Ctrl Pts',(48.4109314680099,-85.425,9.36527991294861));
#42460=CARTESIAN_POINT('Ctrl Pts',(48.4661837816238,-85.725,9.35914063453674));
#42461=CARTESIAN_POINT('Ctrl Pts',(48.4661837816238,-85.425,9.35914063453674));
#42462=CARTESIAN_POINT('Ctrl Pts',(48.4999492168427,-85.725,9.35914063453674));
#42463=CARTESIAN_POINT('Ctrl Pts',(48.4999492168427,-85.425,9.35914063453674));
#42464=CARTESIAN_POINT('',(48.4109314680099,-85.425,9.36527991294861));
#42465=CARTESIAN_POINT('',(48.4109314680099,-85.725,9.36527991294861));
#42466=CARTESIAN_POINT('Ctrl Pts',(48.4109314680099,-85.425,9.36527991294861));
#42467=CARTESIAN_POINT('Ctrl Pts',(48.4661837816238,-85.425,9.35914063453674));
#42468=CARTESIAN_POINT('Ctrl Pts',(48.4999492168427,-85.425,9.35914063453674));
#42469=CARTESIAN_POINT('Origin',(48.3495398759842,-85.725,8.88028705120087));
#42470=CARTESIAN_POINT('',(48.3495398759842,-85.425,8.88028705120087));
#42471=CARTESIAN_POINT('',(48.3495398759842,-85.725,8.88028705120087));
#42472=CARTESIAN_POINT('',(48.3495398759842,-85.425,8.88028705120087));
#42473=CARTESIAN_POINT('Ctrl Pts',(48.7393763065338,-85.725,8.94167864322662));
#42474=CARTESIAN_POINT('Ctrl Pts',(48.7393763065338,-85.425,8.94167864322662));
#42475=CARTESIAN_POINT('Ctrl Pts',(48.5828276872635,-85.725,8.94167864322662));
#42476=CARTESIAN_POINT('Ctrl Pts',(48.5828276872635,-85.425,8.94167864322662));
#42477=CARTESIAN_POINT('Ctrl Pts',(48.3495398759842,-85.725,8.88028705120087));
#42478=CARTESIAN_POINT('Ctrl Pts',(48.3495398759842,-85.425,8.88028705120087));
#42479=CARTESIAN_POINT('',(48.7393763065338,-85.425,8.94167864322662));
#42480=CARTESIAN_POINT('',(48.7393763065338,-85.725,8.94167864322662));
#42481=CARTESIAN_POINT('Ctrl Pts',(48.7393763065338,-85.425,8.94167864322662));
#42482=CARTESIAN_POINT('Ctrl Pts',(48.5828276872635,-85.425,8.94167864322662));
#42483=CARTESIAN_POINT('Ctrl Pts',(48.3495398759842,-85.425,8.88028705120087));
#42484=CARTESIAN_POINT('Ctrl Pts',(49.3717088699341,-85.725,8.69457745552063));
#42485=CARTESIAN_POINT('Ctrl Pts',(49.3717088699341,-85.425,8.69457745552063));
#42486=CARTESIAN_POINT('Ctrl Pts',(49.1230734586716,-85.725,8.94167864322662));
#42487=CARTESIAN_POINT('Ctrl Pts',(49.1230734586716,-85.425,8.94167864322662));
#42488=CARTESIAN_POINT('Ctrl Pts',(48.7393763065338,-85.725,8.94167864322662));
#42489=CARTESIAN_POINT('Ctrl Pts',(48.7393763065338,-85.425,8.94167864322662));
#42490=CARTESIAN_POINT('',(49.3717088699341,-85.425,8.69457745552063));
#42491=CARTESIAN_POINT('',(49.3717088699341,-85.725,8.69457745552063));
#42492=CARTESIAN_POINT('Ctrl Pts',(49.3717088699341,-85.425,8.69457745552063));
#42493=CARTESIAN_POINT('Ctrl Pts',(49.1230734586716,-85.425,8.94167864322662));
#42494=CARTESIAN_POINT('Ctrl Pts',(48.7393763065338,-85.425,8.94167864322662));
#42495=CARTESIAN_POINT('Ctrl Pts',(49.620344877243,-85.725,8.06684875488281));
#42496=CARTESIAN_POINT('Ctrl Pts',(49.620344877243,-85.425,8.06684875488281));
#42497=CARTESIAN_POINT('Ctrl Pts',(49.620344877243,-85.725,8.44747626781464));
#42498=CARTESIAN_POINT('Ctrl Pts',(49.620344877243,-85.425,8.44747626781464));
#42499=CARTESIAN_POINT('Ctrl Pts',(49.3717088699341,-85.725,8.69457745552063));
#42500=CARTESIAN_POINT('Ctrl Pts',(49.3717088699341,-85.425,8.69457745552063));
#42501=CARTESIAN_POINT('',(49.620344877243,-85.425,8.06684875488281));
#42502=CARTESIAN_POINT('',(49.620344877243,-85.725,8.06684875488281));
#42503=CARTESIAN_POINT('Ctrl Pts',(49.620344877243,-85.425,8.06684875488281));
#42504=CARTESIAN_POINT('Ctrl Pts',(49.620344877243,-85.425,8.44747626781464));
#42505=CARTESIAN_POINT('Ctrl Pts',(49.3717088699341,-85.425,8.69457745552063));
#42506=CARTESIAN_POINT('Ctrl Pts',(49.351756811142,-85.725,7.3976811170578));
#42507=CARTESIAN_POINT('Ctrl Pts',(49.351756811142,-85.425,7.3976811170578));
#42508=CARTESIAN_POINT('Ctrl Pts',(49.620344877243,-85.725,7.66780400276184));
#42509=CARTESIAN_POINT('Ctrl Pts',(49.620344877243,-85.425,7.66780400276184));
#42510=CARTESIAN_POINT('Ctrl Pts',(49.620344877243,-85.725,8.06684875488281));
#42511=CARTESIAN_POINT('Ctrl Pts',(49.620344877243,-85.425,8.06684875488281));
#42512=CARTESIAN_POINT('',(49.351756811142,-85.425,7.3976811170578));
#42513=CARTESIAN_POINT('',(49.351756811142,-85.725,7.3976811170578));
#42514=CARTESIAN_POINT('Ctrl Pts',(49.351756811142,-85.425,7.3976811170578));
#42515=CARTESIAN_POINT('Ctrl Pts',(49.620344877243,-85.425,7.66780400276184));
#42516=CARTESIAN_POINT('Ctrl Pts',(49.620344877243,-85.425,8.06684875488281));
#42517=CARTESIAN_POINT('Ctrl Pts',(48.6933323144913,-85.725,7.12755823135376));
#42518=CARTESIAN_POINT('Ctrl Pts',(48.6933323144913,-85.425,7.12755823135376));
#42519=CARTESIAN_POINT('Ctrl Pts',(49.0831687450409,-85.725,7.12755823135376));
#42520=CARTESIAN_POINT('Ctrl Pts',(49.0831687450409,-85.425,7.12755823135376));
#42521=CARTESIAN_POINT('Ctrl Pts',(49.351756811142,-85.725,7.3976811170578));
#42522=CARTESIAN_POINT('Ctrl Pts',(49.351756811142,-85.425,7.3976811170578));
#42523=CARTESIAN_POINT('',(48.6933323144913,-85.425,7.12755823135376));
#42524=CARTESIAN_POINT('',(48.6933323144913,-85.725,7.12755823135376));
#42525=CARTESIAN_POINT('Ctrl Pts',(48.6933323144913,-85.425,7.12755823135376));
#42526=CARTESIAN_POINT('Ctrl Pts',(49.0831687450409,-85.425,7.12755823135376));
#42527=CARTESIAN_POINT('Ctrl Pts',(49.351756811142,-85.425,7.3976811170578));
#42528=CARTESIAN_POINT('Ctrl Pts',(48.136204123497,-85.725,7.33475470542908));
#42529=CARTESIAN_POINT('Ctrl Pts',(48.136204123497,-85.425,7.33475470542908));
#42530=CARTESIAN_POINT('Ctrl Pts',(48.3648877739906,-85.725,7.12755823135376));
#42531=CARTESIAN_POINT('Ctrl Pts',(48.3648877739906,-85.425,7.12755823135376));
#42532=CARTESIAN_POINT('Ctrl Pts',(48.6933323144913,-85.725,7.12755823135376));
#42533=CARTESIAN_POINT('Ctrl Pts',(48.6933323144913,-85.425,7.12755823135376));
#42534=CARTESIAN_POINT('',(48.136204123497,-85.425,7.33475470542908));
#42535=CARTESIAN_POINT('',(48.136204123497,-85.725,7.33475470542908));
#42536=CARTESIAN_POINT('Ctrl Pts',(48.136204123497,-85.425,7.33475470542908));
#42537=CARTESIAN_POINT('Ctrl Pts',(48.3648877739906,-85.425,7.12755823135376));
#42538=CARTESIAN_POINT('Ctrl Pts',(48.6933323144913,-85.425,7.12755823135376));
#42539=CARTESIAN_POINT('Ctrl Pts',(47.812363743782,-85.725,8.01159644126892));
#42540=CARTESIAN_POINT('Ctrl Pts',(47.812363743782,-85.425,8.01159644126892));
#42541=CARTESIAN_POINT('Ctrl Pts',(47.9075207710266,-85.725,7.54195117950439));
#42542=CARTESIAN_POINT('Ctrl Pts',(47.9075207710266,-85.425,7.54195117950439));
#42543=CARTESIAN_POINT('Ctrl Pts',(48.136204123497,-85.725,7.33475470542908));
#42544=CARTESIAN_POINT('Ctrl Pts',(48.136204123497,-85.425,7.33475470542908));
#42545=CARTESIAN_POINT('',(47.812363743782,-85.425,8.01159644126892));
#42546=CARTESIAN_POINT('',(47.812363743782,-85.725,8.01159644126892));
#42547=CARTESIAN_POINT('Ctrl Pts',(47.812363743782,-85.425,8.01159644126892));
#42548=CARTESIAN_POINT('Ctrl Pts',(47.9075207710266,-85.425,7.54195117950439));
#42549=CARTESIAN_POINT('Ctrl Pts',(48.136204123497,-85.425,7.33475470542908));
#42550=CARTESIAN_POINT('Origin',(47.2598400115967,-85.725,7.93792688846588));
#42551=CARTESIAN_POINT('',(47.2598400115967,-85.425,7.93792688846588));
#42552=CARTESIAN_POINT('',(47.2598400115967,-85.725,7.93792688846588));
#42553=CARTESIAN_POINT('',(47.2598400115967,-85.425,7.93792688846588));
#42554=CARTESIAN_POINT('Ctrl Pts',(47.7064635753632,-85.725,7.02319288253784));
#42555=CARTESIAN_POINT('Ctrl Pts',(47.7064635753632,-85.425,7.02319288253784));
#42556=CARTESIAN_POINT('Ctrl Pts',(47.3150923252106,-85.725,7.37619423866272));
#42557=CARTESIAN_POINT('Ctrl Pts',(47.3150923252106,-85.425,7.37619423866272));
#42558=CARTESIAN_POINT('Ctrl Pts',(47.2598400115967,-85.725,7.93792688846588));
#42559=CARTESIAN_POINT('Ctrl Pts',(47.2598400115967,-85.425,7.93792688846588));
#42560=CARTESIAN_POINT('',(47.7064635753632,-85.425,7.02319288253784));
#42561=CARTESIAN_POINT('',(47.7064635753632,-85.725,7.02319288253784));
#42562=CARTESIAN_POINT('Ctrl Pts',(47.7064635753632,-85.425,7.02319288253784));
#42563=CARTESIAN_POINT('Ctrl Pts',(47.3150923252106,-85.425,7.37619423866272));
#42564=CARTESIAN_POINT('Ctrl Pts',(47.2598400115967,-85.425,7.93792688846588));
#42565=CARTESIAN_POINT('Ctrl Pts',(48.6902626752853,-85.725,6.67019152641296));
#42566=CARTESIAN_POINT('Ctrl Pts',(48.6902626752853,-85.425,6.67019152641296));
#42567=CARTESIAN_POINT('Ctrl Pts',(48.0978345274925,-85.725,6.67019152641296));
#42568=CARTESIAN_POINT('Ctrl Pts',(48.0978345274925,-85.425,6.67019152641296));
#42569=CARTESIAN_POINT('Ctrl Pts',(47.7064635753632,-85.725,7.02319288253784));
#42570=CARTESIAN_POINT('Ctrl Pts',(47.7064635753632,-85.425,7.02319288253784));
#42571=CARTESIAN_POINT('Ctrl Pts',(48.6902626752853,-85.425,6.67019152641296));
#42572=CARTESIAN_POINT('Ctrl Pts',(48.0978345274925,-85.425,6.67019152641296));
#42573=CARTESIAN_POINT('Ctrl Pts',(47.7064635753632,-85.425,7.02319288253784));
#42574=CARTESIAN_POINT('Origin',(48.7332367300987,-85.425,8.96930450201035));
#42575=CARTESIAN_POINT('Origin',(69.2472215890884,-85.725,11.2500002384186));
#42576=CARTESIAN_POINT('',(69.2472215890884,-85.425,11.2500002384186));
#42577=CARTESIAN_POINT('',(69.2472215890884,-85.725,11.2500002384186));
#42578=CARTESIAN_POINT('',(69.8427196741104,-85.425,11.2500002384186));
#42579=CARTESIAN_POINT('',(69.2472215890884,-85.425,11.2500002384186));
#42580=CARTESIAN_POINT('',(69.8427196741104,-85.725,11.2500002384186));
#42581=CARTESIAN_POINT('Origin',(69.2472215890884,-85.725,6.75000035762787));
#42582=CARTESIAN_POINT('',(69.2472215890884,-85.425,6.75000035762787));
#42583=CARTESIAN_POINT('',(69.2472215890884,-85.725,6.75000035762787));
#42584=CARTESIAN_POINT('',(69.2472215890884,-85.425,6.75000035762787));
#42585=CARTESIAN_POINT('Origin',(69.8427196741104,-85.725,6.75000035762787));
#42586=CARTESIAN_POINT('',(69.8427196741104,-85.425,6.75000035762787));
#42587=CARTESIAN_POINT('',(69.8427196741104,-85.725,6.75000035762787));
#42588=CARTESIAN_POINT('',(69.8427196741104,-85.425,6.75000035762787));
#42589=CARTESIAN_POINT('Origin',(69.8427196741104,-85.725,11.2500002384186));
#42590=CARTESIAN_POINT('',(69.8427196741104,-85.425,11.2500002384186));
#42591=CARTESIAN_POINT('Origin',(69.5449706315994,-85.425,9.00000029802322));
#42592=CARTESIAN_POINT('Ctrl Pts',(76.8014498949051,-85.725,6.6732611656189));
#42593=CARTESIAN_POINT('Ctrl Pts',(76.8014498949051,-85.425,6.6732611656189));
#42594=CARTESIAN_POINT('Ctrl Pts',(76.1906048059464,-85.725,6.6732611656189));
#42595=CARTESIAN_POINT('Ctrl Pts',(76.1906048059464,-85.425,6.6732611656189));
#42596=CARTESIAN_POINT('Ctrl Pts',(75.7777472734451,-85.725,6.8512966632843));
#42597=CARTESIAN_POINT('Ctrl Pts',(75.7777472734451,-85.425,6.8512966632843));
#42598=CARTESIAN_POINT('',(76.8014498949051,-85.425,6.6732611656189));
#42599=CARTESIAN_POINT('',(76.8014498949051,-85.725,6.6732611656189));
#42600=CARTESIAN_POINT('',(75.7777472734451,-85.425,6.8512966632843));
#42601=CARTESIAN_POINT('Ctrl Pts',(76.8014498949051,-85.425,6.6732611656189));
#42602=CARTESIAN_POINT('Ctrl Pts',(76.1906048059464,-85.425,6.6732611656189));
#42603=CARTESIAN_POINT('Ctrl Pts',(75.7777472734451,-85.425,6.8512966632843));
#42604=CARTESIAN_POINT('',(75.7777472734451,-85.725,6.8512966632843));
#42605=CARTESIAN_POINT('Ctrl Pts',(77.668606877327,-85.725,6.84976184368133));
#42606=CARTESIAN_POINT('Ctrl Pts',(77.668606877327,-85.425,6.84976184368133));
#42607=CARTESIAN_POINT('Ctrl Pts',(77.2833749055862,-85.725,6.6732611656189));
#42608=CARTESIAN_POINT('Ctrl Pts',(77.2833749055862,-85.425,6.6732611656189));
#42609=CARTESIAN_POINT('Ctrl Pts',(76.8014498949051,-85.725,6.6732611656189));
#42610=CARTESIAN_POINT('Ctrl Pts',(76.8014498949051,-85.425,6.6732611656189));
#42611=CARTESIAN_POINT('',(77.668606877327,-85.425,6.84976184368133));
#42612=CARTESIAN_POINT('',(77.668606877327,-85.725,6.84976184368133));
#42613=CARTESIAN_POINT('Ctrl Pts',(77.668606877327,-85.425,6.84976184368133));
#42614=CARTESIAN_POINT('Ctrl Pts',(77.2833749055862,-85.425,6.6732611656189));
#42615=CARTESIAN_POINT('Ctrl Pts',(76.8014498949051,-85.425,6.6732611656189));
#42616=CARTESIAN_POINT('Ctrl Pts',(78.2594987154007,-85.725,7.34396362304687));
#42617=CARTESIAN_POINT('Ctrl Pts',(78.2594987154007,-85.425,7.34396362304687));
#42618=CARTESIAN_POINT('Ctrl Pts',(78.0538388490677,-85.725,7.02626252174377));
#42619=CARTESIAN_POINT('Ctrl Pts',(78.0538388490677,-85.425,7.02626252174377));
#42620=CARTESIAN_POINT('Ctrl Pts',(77.668606877327,-85.725,6.84976184368133));
#42621=CARTESIAN_POINT('Ctrl Pts',(77.668606877327,-85.425,6.84976184368133));
#42622=CARTESIAN_POINT('',(78.2594987154007,-85.425,7.34396362304687));
#42623=CARTESIAN_POINT('',(78.2594987154007,-85.725,7.34396362304687));
#42624=CARTESIAN_POINT('Ctrl Pts',(78.2594987154007,-85.425,7.34396362304687));
#42625=CARTESIAN_POINT('Ctrl Pts',(78.0538388490677,-85.425,7.02626252174377));
#42626=CARTESIAN_POINT('Ctrl Pts',(77.668606877327,-85.425,6.84976184368133));
#42627=CARTESIAN_POINT('Ctrl Pts',(78.4651609659195,-85.725,8.02080535888672));
#42628=CARTESIAN_POINT('Ctrl Pts',(78.4651609659195,-85.425,8.02080535888672));
#42629=CARTESIAN_POINT('Ctrl Pts',(78.4651609659195,-85.725,7.66166472434997));
#42630=CARTESIAN_POINT('Ctrl Pts',(78.4651609659195,-85.425,7.66166472434997));
#42631=CARTESIAN_POINT('Ctrl Pts',(78.2594987154007,-85.725,7.34396362304687));
#42632=CARTESIAN_POINT('Ctrl Pts',(78.2594987154007,-85.425,7.34396362304687));
#42633=CARTESIAN_POINT('',(78.4651609659195,-85.425,8.02080535888672));
#42634=CARTESIAN_POINT('',(78.4651609659195,-85.725,8.02080535888672));
#42635=CARTESIAN_POINT('Ctrl Pts',(78.4651609659195,-85.425,8.02080535888672));
#42636=CARTESIAN_POINT('Ctrl Pts',(78.4651609659195,-85.425,7.66166472434997));
#42637=CARTESIAN_POINT('Ctrl Pts',(78.2594987154007,-85.425,7.34396362304687));
#42638=CARTESIAN_POINT('Ctrl Pts',(78.2779165506363,-85.725,8.66081202030182));
#42639=CARTESIAN_POINT('Ctrl Pts',(78.2779165506363,-85.425,8.66081202030182));
#42640=CARTESIAN_POINT('Ctrl Pts',(78.4651609659195,-85.725,8.38301503658295));
#42641=CARTESIAN_POINT('Ctrl Pts',(78.4651609659195,-85.425,8.38301503658295));
#42642=CARTESIAN_POINT('Ctrl Pts',(78.4651609659195,-85.725,8.02080535888672));
#42643=CARTESIAN_POINT('Ctrl Pts',(78.4651609659195,-85.425,8.02080535888672));
#42644=CARTESIAN_POINT('',(78.2779165506363,-85.425,8.66081202030182));
#42645=CARTESIAN_POINT('',(78.2779165506363,-85.725,8.66081202030182));
#42646=CARTESIAN_POINT('Ctrl Pts',(78.2779165506363,-85.425,8.66081202030182));
#42647=CARTESIAN_POINT('Ctrl Pts',(78.4651609659195,-85.425,8.38301503658295));
#42648=CARTESIAN_POINT('Ctrl Pts',(78.4651609659195,-85.425,8.02080535888672));
#42649=CARTESIAN_POINT('Ctrl Pts',(77.6977654695511,-85.725,9.11971354484558));
#42650=CARTESIAN_POINT('Ctrl Pts',(77.6977654695511,-85.425,9.11971354484558));
#42651=CARTESIAN_POINT('Ctrl Pts',(78.0906721353531,-85.725,8.93860900402069));
#42652=CARTESIAN_POINT('Ctrl Pts',(78.0906721353531,-85.425,8.93860900402069));
#42653=CARTESIAN_POINT('Ctrl Pts',(78.2779165506363,-85.725,8.66081202030182));
#42654=CARTESIAN_POINT('Ctrl Pts',(78.2779165506363,-85.425,8.66081202030182));
#42655=CARTESIAN_POINT('',(77.6977654695511,-85.425,9.11971354484558));
#42656=CARTESIAN_POINT('',(77.6977654695511,-85.725,9.11971354484558));
#42657=CARTESIAN_POINT('Ctrl Pts',(77.6977654695511,-85.425,9.11971354484558));
#42658=CARTESIAN_POINT('Ctrl Pts',(78.0906721353531,-85.425,8.93860900402069));
#42659=CARTESIAN_POINT('Ctrl Pts',(78.2779165506363,-85.425,8.66081202030182));
#42660=CARTESIAN_POINT('Ctrl Pts',(76.7016884088516,-85.725,9.4067188501358));
#42661=CARTESIAN_POINT('Ctrl Pts',(76.7016884088516,-85.425,9.4067188501358));
#42662=CARTESIAN_POINT('Ctrl Pts',(77.4276443719864,-85.725,9.24249672889709));
#42663=CARTESIAN_POINT('Ctrl Pts',(77.4276443719864,-85.425,9.24249672889709));
#42664=CARTESIAN_POINT('Ctrl Pts',(77.6977654695511,-85.725,9.11971354484558));
#42665=CARTESIAN_POINT('Ctrl Pts',(77.6977654695511,-85.425,9.11971354484558));
#42666=CARTESIAN_POINT('',(76.7016884088516,-85.425,9.4067188501358));
#42667=CARTESIAN_POINT('',(76.7016884088516,-85.725,9.4067188501358));
#42668=CARTESIAN_POINT('Ctrl Pts',(76.7016884088516,-85.425,9.4067188501358));
#42669=CARTESIAN_POINT('Ctrl Pts',(77.4276443719864,-85.425,9.24249672889709));
#42670=CARTESIAN_POINT('Ctrl Pts',(77.6977654695511,-85.425,9.11971354484558));
#42671=CARTESIAN_POINT('Ctrl Pts',(75.8038374185562,-85.725,9.72748959064484));
#42672=CARTESIAN_POINT('Ctrl Pts',(75.8038374185562,-85.425,9.72748959064484));
#42673=CARTESIAN_POINT('Ctrl Pts',(75.9757348299026,-85.725,9.57094156742096));
#42674=CARTESIAN_POINT('Ctrl Pts',(75.9757348299026,-85.425,9.57094156742096));
#42675=CARTESIAN_POINT('Ctrl Pts',(76.7016884088516,-85.725,9.4067188501358));
#42676=CARTESIAN_POINT('Ctrl Pts',(76.7016884088516,-85.425,9.4067188501358));
#42677=CARTESIAN_POINT('',(75.8038374185562,-85.425,9.72748959064484));
#42678=CARTESIAN_POINT('',(75.8038374185562,-85.725,9.72748959064484));
#42679=CARTESIAN_POINT('Ctrl Pts',(75.8038374185562,-85.425,9.72748959064484));
#42680=CARTESIAN_POINT('Ctrl Pts',(75.9757348299026,-85.425,9.57094156742096));
#42681=CARTESIAN_POINT('Ctrl Pts',(76.7016884088516,-85.425,9.4067188501358));
#42682=CARTESIAN_POINT('Ctrl Pts',(75.6288715600967,-85.725,10.1265349388123));
#42683=CARTESIAN_POINT('Ctrl Pts',(75.6288715600967,-85.425,10.1265349388123));
#42684=CARTESIAN_POINT('Ctrl Pts',(75.6288715600967,-85.725,9.88403820991516));
#42685=CARTESIAN_POINT('Ctrl Pts',(75.6288715600967,-85.425,9.88403820991516));
#42686=CARTESIAN_POINT('Ctrl Pts',(75.8038374185562,-85.725,9.72748959064484));
#42687=CARTESIAN_POINT('Ctrl Pts',(75.8038374185562,-85.425,9.72748959064484));
#42688=CARTESIAN_POINT('',(75.6288715600967,-85.425,10.1265349388123));
#42689=CARTESIAN_POINT('',(75.6288715600967,-85.725,10.1265349388123));
#42690=CARTESIAN_POINT('Ctrl Pts',(75.6288715600967,-85.425,10.1265349388123));
#42691=CARTESIAN_POINT('Ctrl Pts',(75.6288715600967,-85.425,9.88403820991516));
#42692=CARTESIAN_POINT('Ctrl Pts',(75.8038374185562,-85.425,9.72748959064484));
#42693=CARTESIAN_POINT('Ctrl Pts',(75.8759733438492,-85.725,10.6038540005684));
#42694=CARTESIAN_POINT('Ctrl Pts',(75.8759733438492,-85.425,10.6038540005684));
#42695=CARTESIAN_POINT('Ctrl Pts',(75.6288715600967,-85.725,10.4058664441109));
#42696=CARTESIAN_POINT('Ctrl Pts',(75.6288715600967,-85.425,10.4058664441109));
#42697=CARTESIAN_POINT('Ctrl Pts',(75.6288715600967,-85.725,10.1265349388123));
#42698=CARTESIAN_POINT('Ctrl Pts',(75.6288715600967,-85.425,10.1265349388123));
#42699=CARTESIAN_POINT('',(75.8759733438492,-85.425,10.6038540005684));
#42700=CARTESIAN_POINT('',(75.8759733438492,-85.725,10.6038540005684));
#42701=CARTESIAN_POINT('Ctrl Pts',(75.8759733438492,-85.425,10.6038540005684));
#42702=CARTESIAN_POINT('Ctrl Pts',(75.6288715600967,-85.425,10.4058664441109));
#42703=CARTESIAN_POINT('Ctrl Pts',(75.6288715600967,-85.425,10.1265349388123));
#42704=CARTESIAN_POINT('Ctrl Pts',(76.6633197069168,-85.725,10.8018418550491));
#42705=CARTESIAN_POINT('Ctrl Pts',(76.6633197069168,-85.425,10.8018418550491));
#42706=CARTESIAN_POINT('Ctrl Pts',(76.1230727434158,-85.725,10.8018418550491));
#42707=CARTESIAN_POINT('Ctrl Pts',(76.1230727434158,-85.425,10.8018418550491));
#42708=CARTESIAN_POINT('Ctrl Pts',(75.8759733438492,-85.725,10.6038540005684));
#42709=CARTESIAN_POINT('Ctrl Pts',(75.8759733438492,-85.425,10.6038540005684));
#42710=CARTESIAN_POINT('',(76.6633197069168,-85.425,10.8018418550491));
#42711=CARTESIAN_POINT('',(76.6633197069168,-85.725,10.8018418550491));
#42712=CARTESIAN_POINT('Ctrl Pts',(76.6633197069168,-85.425,10.8018418550491));
#42713=CARTESIAN_POINT('Ctrl Pts',(76.1230727434158,-85.425,10.8018418550491));
#42714=CARTESIAN_POINT('Ctrl Pts',(75.8759733438492,-85.425,10.6038540005684));
#42715=CARTESIAN_POINT('Ctrl Pts',(77.4475952386856,-85.725,10.5839019417763));
#42716=CARTESIAN_POINT('Ctrl Pts',(77.4475952386856,-85.425,10.5839019417763));
#42717=CARTESIAN_POINT('Ctrl Pts',(77.1820780038834,-85.725,10.8018418550491));
#42718=CARTESIAN_POINT('Ctrl Pts',(77.1820780038834,-85.425,10.8018418550491));
#42719=CARTESIAN_POINT('Ctrl Pts',(76.6633197069168,-85.725,10.8018418550491));
#42720=CARTESIAN_POINT('Ctrl Pts',(76.6633197069168,-85.425,10.8018418550491));
#42721=CARTESIAN_POINT('',(77.4475952386856,-85.425,10.5839019417763));
#42722=CARTESIAN_POINT('',(77.4475952386856,-85.725,10.5839019417763));
#42723=CARTESIAN_POINT('Ctrl Pts',(77.4475952386856,-85.425,10.5839019417763));
#42724=CARTESIAN_POINT('Ctrl Pts',(77.1820780038834,-85.425,10.8018418550491));
#42725=CARTESIAN_POINT('Ctrl Pts',(76.6633197069168,-85.425,10.8018418550491));
#42726=CARTESIAN_POINT('Ctrl Pts',(77.7591582536697,-85.725,9.9392911195755));
#42727=CARTESIAN_POINT('Ctrl Pts',(77.7591582536697,-85.425,9.9392911195755));
#42728=CARTESIAN_POINT('Ctrl Pts',(77.7131148576736,-85.725,10.3659620285034));
#42729=CARTESIAN_POINT('Ctrl Pts',(77.7131148576736,-85.425,10.3659620285034));
#42730=CARTESIAN_POINT('Ctrl Pts',(77.4475952386856,-85.725,10.5839019417763));
#42731=CARTESIAN_POINT('Ctrl Pts',(77.4475952386856,-85.425,10.5839019417763));
#42732=CARTESIAN_POINT('',(77.7591582536697,-85.425,9.9392911195755));
#42733=CARTESIAN_POINT('',(77.7591582536697,-85.725,9.9392911195755));
#42734=CARTESIAN_POINT('Ctrl Pts',(77.7591582536697,-85.425,9.9392911195755));
#42735=CARTESIAN_POINT('Ctrl Pts',(77.7131148576736,-85.425,10.3659620285034));
#42736=CARTESIAN_POINT('Ctrl Pts',(77.4475952386856,-85.425,10.5839019417763));
#42737=CARTESIAN_POINT('Origin',(78.3300992250443,-85.725,9.98226487636566));
#42738=CARTESIAN_POINT('',(78.3300992250443,-85.425,9.98226487636566));
#42739=CARTESIAN_POINT('',(78.3300992250443,-85.725,9.98226487636566));
#42740=CARTESIAN_POINT('',(78.3300992250443,-85.425,9.98226487636566));
#42741=CARTESIAN_POINT('Ctrl Pts',(78.1090899705887,-85.725,10.6913369297981));
#42742=CARTESIAN_POINT('Ctrl Pts',(78.1090899705887,-85.425,10.6913369297981));
#42743=CARTESIAN_POINT('Ctrl Pts',(78.3147522211075,-85.725,10.3782402873039));
#42744=CARTESIAN_POINT('Ctrl Pts',(78.3147522211075,-85.425,10.3782402873039));
#42745=CARTESIAN_POINT('Ctrl Pts',(78.3300992250443,-85.725,9.98226487636566));
#42746=CARTESIAN_POINT('Ctrl Pts',(78.3300992250443,-85.425,9.98226487636566));
#42747=CARTESIAN_POINT('',(78.1090899705887,-85.425,10.6913369297981));
#42748=CARTESIAN_POINT('',(78.1090899705887,-85.725,10.6913369297981));
#42749=CARTESIAN_POINT('Ctrl Pts',(78.1090899705887,-85.425,10.6913369297981));
#42750=CARTESIAN_POINT('Ctrl Pts',(78.3147522211075,-85.425,10.3782402873039));
#42751=CARTESIAN_POINT('Ctrl Pts',(78.3300992250443,-85.425,9.98226487636566));
#42752=CARTESIAN_POINT('Ctrl Pts',(77.521266579628,-85.725,11.1655866503716));
#42753=CARTESIAN_POINT('Ctrl Pts',(77.521266579628,-85.425,11.1655866503716));
#42754=CARTESIAN_POINT('Ctrl Pts',(77.9034277200699,-85.725,11.0044338703156));
#42755=CARTESIAN_POINT('Ctrl Pts',(77.9034277200699,-85.425,11.0044338703156));
#42756=CARTESIAN_POINT('Ctrl Pts',(78.1090899705887,-85.725,10.6913369297981));
#42757=CARTESIAN_POINT('Ctrl Pts',(78.1090899705887,-85.425,10.6913369297981));
#42758=CARTESIAN_POINT('',(77.521266579628,-85.425,11.1655866503716));
#42759=CARTESIAN_POINT('',(77.521266579628,-85.725,11.1655866503716));
#42760=CARTESIAN_POINT('Ctrl Pts',(77.521266579628,-85.425,11.1655866503716));
#42761=CARTESIAN_POINT('Ctrl Pts',(77.9034277200699,-85.425,11.0044338703156));
#42762=CARTESIAN_POINT('Ctrl Pts',(78.1090899705887,-85.425,10.6913369297981));
#42763=CARTESIAN_POINT('Ctrl Pts',(76.6387625932693,-85.725,11.3267394304276));
#42764=CARTESIAN_POINT('Ctrl Pts',(76.6387625932693,-85.425,11.3267394304276));
#42765=CARTESIAN_POINT('Ctrl Pts',(77.1391030550003,-85.725,11.3267394304276));
#42766=CARTESIAN_POINT('Ctrl Pts',(77.1391030550003,-85.425,11.3267394304276));
#42767=CARTESIAN_POINT('Ctrl Pts',(77.521266579628,-85.725,11.1655866503716));
#42768=CARTESIAN_POINT('Ctrl Pts',(77.521266579628,-85.425,11.1655866503716));
#42769=CARTESIAN_POINT('',(76.6387625932693,-85.425,11.3267394304276));
#42770=CARTESIAN_POINT('',(76.6387625932693,-85.725,11.3267394304276));
#42771=CARTESIAN_POINT('Ctrl Pts',(76.6387625932693,-85.425,11.3267394304276));
#42772=CARTESIAN_POINT('Ctrl Pts',(77.1391030550003,-85.425,11.3267394304276));
#42773=CARTESIAN_POINT('Ctrl Pts',(77.521266579628,-85.425,11.1655866503716));
#42774=CARTESIAN_POINT('Ctrl Pts',(75.8130475282669,-85.725,11.1732607483864));
#42775=CARTESIAN_POINT('Ctrl Pts',(75.8130475282669,-85.425,11.1732607483864));
#42776=CARTESIAN_POINT('Ctrl Pts',(76.1844655275345,-85.725,11.3267394304276));
#42777=CARTESIAN_POINT('Ctrl Pts',(76.1844655275345,-85.425,11.3267394304276));
#42778=CARTESIAN_POINT('Ctrl Pts',(76.6387625932693,-85.725,11.3267394304276));
#42779=CARTESIAN_POINT('Ctrl Pts',(76.6387625932693,-85.425,11.3267394304276));
#42780=CARTESIAN_POINT('',(75.8130475282669,-85.425,11.1732607483864));
#42781=CARTESIAN_POINT('',(75.8130475282669,-85.725,11.1732607483864));
#42782=CARTESIAN_POINT('Ctrl Pts',(75.8130475282669,-85.425,11.1732607483864));
#42783=CARTESIAN_POINT('Ctrl Pts',(76.1844655275345,-85.425,11.3267394304276));
#42784=CARTESIAN_POINT('Ctrl Pts',(76.6387625932693,-85.425,11.3267394304276));
#42785=CARTESIAN_POINT('Ctrl Pts',(75.2482434511185,-85.725,10.723567545414));
#42786=CARTESIAN_POINT('Ctrl Pts',(75.2482434511185,-85.425,10.723567545414));
#42787=CARTESIAN_POINT('Ctrl Pts',(75.4416271448135,-85.725,11.019781768322));
#42788=CARTESIAN_POINT('Ctrl Pts',(75.4416271448135,-85.425,11.019781768322));
#42789=CARTESIAN_POINT('Ctrl Pts',(75.8130475282669,-85.725,11.1732607483864));
#42790=CARTESIAN_POINT('Ctrl Pts',(75.8130475282669,-85.425,11.1732607483864));
#42791=CARTESIAN_POINT('',(75.2482434511185,-85.425,10.723567545414));
#42792=CARTESIAN_POINT('',(75.2482434511185,-85.725,10.723567545414));
#42793=CARTESIAN_POINT('Ctrl Pts',(75.2482434511185,-85.425,10.723567545414));
#42794=CARTESIAN_POINT('Ctrl Pts',(75.4416271448135,-85.425,11.019781768322));
#42795=CARTESIAN_POINT('Ctrl Pts',(75.8130475282669,-85.425,11.1732607483864));
#42796=CARTESIAN_POINT('Ctrl Pts',(75.0548621416092,-85.725,10.0866302251816));
#42797=CARTESIAN_POINT('Ctrl Pts',(75.0548621416092,-85.425,10.0866302251816));
#42798=CARTESIAN_POINT('Ctrl Pts',(75.0548621416092,-85.725,10.427353322506));
#42799=CARTESIAN_POINT('Ctrl Pts',(75.0548621416092,-85.425,10.427353322506));
#42800=CARTESIAN_POINT('Ctrl Pts',(75.2482434511185,-85.725,10.723567545414));
#42801=CARTESIAN_POINT('Ctrl Pts',(75.2482434511185,-85.425,10.723567545414));
#42802=CARTESIAN_POINT('',(75.0548621416092,-85.425,10.0866302251816));
#42803=CARTESIAN_POINT('',(75.0548621416092,-85.725,10.0866302251816));
#42804=CARTESIAN_POINT('Ctrl Pts',(75.0548621416092,-85.425,10.0866302251816));
#42805=CARTESIAN_POINT('Ctrl Pts',(75.0548621416092,-85.425,10.427353322506));
#42806=CARTESIAN_POINT('Ctrl Pts',(75.2482434511185,-85.425,10.723567545414));
#42807=CARTESIAN_POINT('Ctrl Pts',(75.2129431962967,-85.725,9.52643239498138));
#42808=CARTESIAN_POINT('Ctrl Pts',(75.2129431962967,-85.425,9.52643239498138));
#42809=CARTESIAN_POINT('Ctrl Pts',(75.0548621416092,-85.725,9.77660322189331));
#42810=CARTESIAN_POINT('Ctrl Pts',(75.0548621416092,-85.425,9.77660322189331));
#42811=CARTESIAN_POINT('Ctrl Pts',(75.0548621416092,-85.725,10.0866302251816));
#42812=CARTESIAN_POINT('Ctrl Pts',(75.0548621416092,-85.425,10.0866302251816));
#42813=CARTESIAN_POINT('',(75.2129431962967,-85.425,9.52643239498138));
#42814=CARTESIAN_POINT('',(75.2129431962967,-85.725,9.52643239498138));
#42815=CARTESIAN_POINT('Ctrl Pts',(75.2129431962967,-85.425,9.52643239498138));
#42816=CARTESIAN_POINT('Ctrl Pts',(75.0548621416092,-85.425,9.77660322189331));
#42817=CARTESIAN_POINT('Ctrl Pts',(75.0548621416092,-85.425,10.0866302251816));
#42818=CARTESIAN_POINT('Ctrl Pts',(75.6933327913284,-85.725,9.1074355840683));
#42819=CARTESIAN_POINT('Ctrl Pts',(75.6933327913284,-85.425,9.1074355840683));
#42820=CARTESIAN_POINT('Ctrl Pts',(75.37102663517,-85.725,9.27626216411591));
#42821=CARTESIAN_POINT('Ctrl Pts',(75.37102663517,-85.425,9.27626216411591));
#42822=CARTESIAN_POINT('Ctrl Pts',(75.2129431962967,-85.725,9.52643239498138));
#42823=CARTESIAN_POINT('Ctrl Pts',(75.2129431962967,-85.425,9.52643239498138));
#42824=CARTESIAN_POINT('',(75.6933327913284,-85.425,9.1074355840683));
#42825=CARTESIAN_POINT('',(75.6933327913284,-85.725,9.1074355840683));
#42826=CARTESIAN_POINT('Ctrl Pts',(75.6933327913284,-85.425,9.1074355840683));
#42827=CARTESIAN_POINT('Ctrl Pts',(75.37102663517,-85.425,9.27626216411591));
#42828=CARTESIAN_POINT('Ctrl Pts',(75.2129431962967,-85.425,9.52643239498138));
#42829=CARTESIAN_POINT('Ctrl Pts',(76.5620228052139,-85.725,8.82656896114349));
#42830=CARTESIAN_POINT('Ctrl Pts',(76.5620228052139,-85.425,8.82656896114349));
#42831=CARTESIAN_POINT('Ctrl Pts',(75.9419699907303,-85.725,8.97544348239899));
#42832=CARTESIAN_POINT('Ctrl Pts',(75.9419699907303,-85.425,8.97544348239899));
#42833=CARTESIAN_POINT('Ctrl Pts',(75.6933327913284,-85.725,9.1074355840683));
#42834=CARTESIAN_POINT('Ctrl Pts',(75.6933327913284,-85.425,9.1074355840683));
#42835=CARTESIAN_POINT('',(76.5620228052139,-85.425,8.82656896114349));
#42836=CARTESIAN_POINT('',(76.5620228052139,-85.725,8.82656896114349));
#42837=CARTESIAN_POINT('Ctrl Pts',(76.5620228052139,-85.425,8.82656896114349));
#42838=CARTESIAN_POINT('Ctrl Pts',(75.9419699907303,-85.425,8.97544348239899));
#42839=CARTESIAN_POINT('Ctrl Pts',(75.6933327913284,-85.425,9.1074355840683));
#42840=CARTESIAN_POINT('Ctrl Pts',(77.3631831407547,-85.725,8.60709452629089));
#42841=CARTESIAN_POINT('Ctrl Pts',(77.3631831407547,-85.425,8.60709452629089));
#42842=CARTESIAN_POINT('Ctrl Pts',(77.1820780038834,-85.725,8.677694439888));
#42843=CARTESIAN_POINT('Ctrl Pts',(77.1820780038834,-85.425,8.677694439888));
#42844=CARTESIAN_POINT('Ctrl Pts',(76.5620228052139,-85.725,8.82656896114349));
#42845=CARTESIAN_POINT('Ctrl Pts',(76.5620228052139,-85.425,8.82656896114349));
#42846=CARTESIAN_POINT('',(77.3631831407547,-85.425,8.60709452629089));
#42847=CARTESIAN_POINT('',(77.3631831407547,-85.725,8.60709452629089));
#42848=CARTESIAN_POINT('Ctrl Pts',(77.3631831407547,-85.425,8.60709452629089));
#42849=CARTESIAN_POINT('Ctrl Pts',(77.1820780038834,-85.425,8.677694439888));
#42850=CARTESIAN_POINT('Ctrl Pts',(76.5620228052139,-85.425,8.82656896114349));
#42851=CARTESIAN_POINT('Ctrl Pts',(77.7683659791946,-85.725,8.34157609939575));
#42852=CARTESIAN_POINT('Ctrl Pts',(77.7683659791946,-85.425,8.34157609939575));
#42853=CARTESIAN_POINT('Ctrl Pts',(77.6455851793289,-85.725,8.4996589422226));
#42854=CARTESIAN_POINT('Ctrl Pts',(77.6455851793289,-85.425,8.4996589422226));
#42855=CARTESIAN_POINT('Ctrl Pts',(77.3631831407547,-85.725,8.60709452629089));
#42856=CARTESIAN_POINT('Ctrl Pts',(77.3631831407547,-85.425,8.60709452629089));
#42857=CARTESIAN_POINT('',(77.7683659791946,-85.425,8.34157609939575));
#42858=CARTESIAN_POINT('',(77.7683659791946,-85.725,8.34157609939575));
#42859=CARTESIAN_POINT('Ctrl Pts',(77.7683659791946,-85.425,8.34157609939575));
#42860=CARTESIAN_POINT('Ctrl Pts',(77.6455851793289,-85.425,8.4996589422226));
#42861=CARTESIAN_POINT('Ctrl Pts',(77.3631831407547,-85.425,8.60709452629089));
#42862=CARTESIAN_POINT('Ctrl Pts',(77.8911491632462,-85.725,7.97169172763824));
#42863=CARTESIAN_POINT('Ctrl Pts',(77.8911491632462,-85.425,7.97169172763824));
#42864=CARTESIAN_POINT('Ctrl Pts',(77.8911491632462,-85.725,8.18349266052246));
#42865=CARTESIAN_POINT('Ctrl Pts',(77.8911491632462,-85.425,8.18349266052246));
#42866=CARTESIAN_POINT('Ctrl Pts',(77.7683659791946,-85.725,8.34157609939575));
#42867=CARTESIAN_POINT('Ctrl Pts',(77.7683659791946,-85.425,8.34157609939575));
#42868=CARTESIAN_POINT('',(77.8911491632462,-85.425,7.97169172763824));
#42869=CARTESIAN_POINT('',(77.8911491632462,-85.725,7.97169172763824));
#42870=CARTESIAN_POINT('Ctrl Pts',(77.8911491632462,-85.425,7.97169172763824));
#42871=CARTESIAN_POINT('Ctrl Pts',(77.8911491632462,-85.425,8.18349266052246));
#42872=CARTESIAN_POINT('Ctrl Pts',(77.7683659791946,-85.425,8.34157609939575));
#42873=CARTESIAN_POINT('Ctrl Pts',(77.7637621164322,-85.725,7.58645975589752));
#42874=CARTESIAN_POINT('Ctrl Pts',(77.7637621164322,-85.425,7.58645975589752));
#42875=CARTESIAN_POINT('Ctrl Pts',(77.8911491632462,-85.725,7.76296103000641));
#42876=CARTESIAN_POINT('Ctrl Pts',(77.8911491632462,-85.425,7.76296103000641));
#42877=CARTESIAN_POINT('Ctrl Pts',(77.8911491632462,-85.725,7.97169172763824));
#42878=CARTESIAN_POINT('Ctrl Pts',(77.8911491632462,-85.425,7.97169172763824));
#42879=CARTESIAN_POINT('',(77.7637621164322,-85.425,7.58645975589752));
#42880=CARTESIAN_POINT('',(77.7637621164322,-85.725,7.58645975589752));
#42881=CARTESIAN_POINT('Ctrl Pts',(77.7637621164322,-85.425,7.58645975589752));
#42882=CARTESIAN_POINT('Ctrl Pts',(77.8911491632462,-85.425,7.76296103000641));
#42883=CARTESIAN_POINT('Ctrl Pts',(77.8911491632462,-85.425,7.97169172763824));
#42884=CARTESIAN_POINT('Ctrl Pts',(77.3754616975784,-85.725,7.3086633682251));
#42885=CARTESIAN_POINT('Ctrl Pts',(77.3754616975784,-85.425,7.3086633682251));
#42886=CARTESIAN_POINT('Ctrl Pts',(77.6363750696182,-85.725,7.40995967388153));
#42887=CARTESIAN_POINT('Ctrl Pts',(77.6363750696182,-85.425,7.40995967388153));
#42888=CARTESIAN_POINT('Ctrl Pts',(77.7637621164322,-85.725,7.58645975589752));
#42889=CARTESIAN_POINT('Ctrl Pts',(77.7637621164322,-85.425,7.58645975589752));
#42890=CARTESIAN_POINT('',(77.3754616975784,-85.425,7.3086633682251));
#42891=CARTESIAN_POINT('',(77.3754616975784,-85.725,7.3086633682251));
#42892=CARTESIAN_POINT('Ctrl Pts',(77.3754616975784,-85.425,7.3086633682251));
#42893=CARTESIAN_POINT('Ctrl Pts',(77.6363750696182,-85.425,7.40995967388153));
#42894=CARTESIAN_POINT('Ctrl Pts',(77.7637621164322,-85.425,7.58645975589752));
#42895=CARTESIAN_POINT('Ctrl Pts',(76.7738243341446,-85.725,7.20736706256866));
#42896=CARTESIAN_POINT('Ctrl Pts',(76.7738243341446,-85.425,7.20736706256866));
#42897=CARTESIAN_POINT('Ctrl Pts',(77.1145459413528,-85.725,7.20736706256866));
#42898=CARTESIAN_POINT('Ctrl Pts',(77.1145459413528,-85.425,7.20736706256866));
#42899=CARTESIAN_POINT('Ctrl Pts',(77.3754616975784,-85.725,7.3086633682251));
#42900=CARTESIAN_POINT('Ctrl Pts',(77.3754616975784,-85.425,7.3086633682251));
#42901=CARTESIAN_POINT('',(76.7738243341446,-85.425,7.20736706256866));
#42902=CARTESIAN_POINT('',(76.7738243341446,-85.725,7.20736706256866));
#42903=CARTESIAN_POINT('Ctrl Pts',(76.7738243341446,-85.425,7.20736706256866));
#42904=CARTESIAN_POINT('Ctrl Pts',(77.1145459413528,-85.425,7.20736706256866));
#42905=CARTESIAN_POINT('Ctrl Pts',(77.3754616975784,-85.425,7.3086633682251));
#42906=CARTESIAN_POINT('Ctrl Pts',(76.0831686258316,-85.725,7.34089398384094));
#42907=CARTESIAN_POINT('Ctrl Pts',(76.0831686258316,-85.425,7.34089398384094));
#42908=CARTESIAN_POINT('Ctrl Pts',(76.3901277780533,-85.725,7.20736706256866));
#42909=CARTESIAN_POINT('Ctrl Pts',(76.3901277780533,-85.425,7.20736706256866));
#42910=CARTESIAN_POINT('Ctrl Pts',(76.7738243341446,-85.725,7.20736706256866));
#42911=CARTESIAN_POINT('Ctrl Pts',(76.7738243341446,-85.425,7.20736706256866));
#42912=CARTESIAN_POINT('',(76.0831686258316,-85.425,7.34089398384094));
#42913=CARTESIAN_POINT('',(76.0831686258316,-85.725,7.34089398384094));
#42914=CARTESIAN_POINT('Ctrl Pts',(76.0831686258316,-85.425,7.34089398384094));
#42915=CARTESIAN_POINT('Ctrl Pts',(76.3901277780533,-85.425,7.20736706256866));
#42916=CARTESIAN_POINT('Ctrl Pts',(76.7738243341446,-85.425,7.20736706256866));
#42917=CARTESIAN_POINT('Ctrl Pts',(75.6304069757462,-85.725,7.69082570075989));
#42918=CARTESIAN_POINT('Ctrl Pts',(75.6304069757462,-85.425,7.69082570075989));
#42919=CARTESIAN_POINT('Ctrl Pts',(75.7762118577957,-85.725,7.47442030906677));
#42920=CARTESIAN_POINT('Ctrl Pts',(75.7762118577957,-85.425,7.47442030906677));
#42921=CARTESIAN_POINT('Ctrl Pts',(76.0831686258316,-85.725,7.34089398384094));
#42922=CARTESIAN_POINT('Ctrl Pts',(76.0831686258316,-85.425,7.34089398384094));
#42923=CARTESIAN_POINT('',(75.6304069757462,-85.425,7.69082570075989));
#42924=CARTESIAN_POINT('',(75.6304069757462,-85.725,7.69082570075989));
#42925=CARTESIAN_POINT('Ctrl Pts',(75.6304069757462,-85.425,7.69082570075989));
#42926=CARTESIAN_POINT('Ctrl Pts',(75.7762118577957,-85.425,7.47442030906677));
#42927=CARTESIAN_POINT('Ctrl Pts',(76.0831686258316,-85.425,7.34089398384094));
#42928=CARTESIAN_POINT('Ctrl Pts',(75.4446979761124,-85.725,8.24488425254822));
#42929=CARTESIAN_POINT('Ctrl Pts',(75.4446979761124,-85.425,8.24488425254822));
#42930=CARTESIAN_POINT('Ctrl Pts',(75.4846020936966,-85.725,7.907231092453));
#42931=CARTESIAN_POINT('Ctrl Pts',(75.4846020936966,-85.425,7.907231092453));
#42932=CARTESIAN_POINT('Ctrl Pts',(75.6304069757462,-85.725,7.69082570075989));
#42933=CARTESIAN_POINT('Ctrl Pts',(75.6304069757462,-85.425,7.69082570075989));
#42934=CARTESIAN_POINT('',(75.4446979761124,-85.425,8.24488425254822));
#42935=CARTESIAN_POINT('',(75.4446979761124,-85.725,8.24488425254822));
#42936=CARTESIAN_POINT('Ctrl Pts',(75.4446979761124,-85.425,8.24488425254822));
#42937=CARTESIAN_POINT('Ctrl Pts',(75.4846020936966,-85.425,7.907231092453));
#42938=CARTESIAN_POINT('Ctrl Pts',(75.6304069757462,-85.425,7.69082570075989));
#42939=CARTESIAN_POINT('Origin',(74.8829647302628,-85.725,8.19577121734619));
#42940=CARTESIAN_POINT('',(74.8829647302628,-85.425,8.19577121734619));
#42941=CARTESIAN_POINT('',(74.8829647302628,-85.725,8.19577121734619));
#42942=CARTESIAN_POINT('',(74.8829647302628,-85.425,8.19577121734619));
#42943=CARTESIAN_POINT('Ctrl Pts',(75.1300665140152,-85.725,7.38693737983704));
#42944=CARTESIAN_POINT('Ctrl Pts',(75.1300665140152,-85.425,7.38693737983704));
#42945=CARTESIAN_POINT('Ctrl Pts',(74.8952432870865,-85.725,7.74454319477081));
#42946=CARTESIAN_POINT('Ctrl Pts',(74.8952432870865,-85.425,7.74454319477081));
#42947=CARTESIAN_POINT('Ctrl Pts',(74.8829647302628,-85.725,8.19577121734619));
#42948=CARTESIAN_POINT('Ctrl Pts',(74.8829647302628,-85.425,8.19577121734619));
#42949=CARTESIAN_POINT('',(75.1300665140152,-85.425,7.38693737983704));
#42950=CARTESIAN_POINT('',(75.1300665140152,-85.725,7.38693737983704));
#42951=CARTESIAN_POINT('Ctrl Pts',(75.1300665140152,-85.425,7.38693737983704));
#42952=CARTESIAN_POINT('Ctrl Pts',(74.8952432870865,-85.425,7.74454319477081));
#42953=CARTESIAN_POINT('Ctrl Pts',(74.8829647302628,-85.425,8.19577121734619));
#42954=CARTESIAN_POINT('Ctrl Pts',(75.7777472734451,-85.725,6.8512966632843));
#42955=CARTESIAN_POINT('Ctrl Pts',(75.7777472734451,-85.425,6.8512966632843));
#42956=CARTESIAN_POINT('Ctrl Pts',(75.3648873567581,-85.725,7.02933156490326));
#42957=CARTESIAN_POINT('Ctrl Pts',(75.3648873567581,-85.425,7.02933156490326));
#42958=CARTESIAN_POINT('Ctrl Pts',(75.1300665140152,-85.725,7.38693737983704));
#42959=CARTESIAN_POINT('Ctrl Pts',(75.1300665140152,-85.425,7.38693737983704));
#42960=CARTESIAN_POINT('Ctrl Pts',(75.7777472734451,-85.425,6.8512966632843));
#42961=CARTESIAN_POINT('Ctrl Pts',(75.3648873567581,-85.425,7.02933156490326));
#42962=CARTESIAN_POINT('Ctrl Pts',(75.1300665140152,-85.425,7.38693737983704));
#42963=CARTESIAN_POINT('Origin',(76.6740628480911,-85.425,9.00000029802322));
#42964=CARTESIAN_POINT('Origin',(0.,0.,0.2));
#42965=CARTESIAN_POINT('',(-4.05,-4.95981953654678E-16,0.4));
#42966=CARTESIAN_POINT('',(-4.25,5.20474889637625E-16,0.2));
#42967=CARTESIAN_POINT('Origin',(0.,0.,0.4));
#42968=CARTESIAN_POINT('Origin',(0.,0.,19.05));
#42969=CARTESIAN_POINT('',(-4.05,-4.95981953654678E-16,17.35));
#42970=CARTESIAN_POINT('Origin',(0.,0.,17.35));
#42971=CARTESIAN_POINT('',(-4.05,4.95981953654678E-16,19.05));
#42972=CARTESIAN_POINT('Origin',(56.25,-78.,18.85));
#42973=CARTESIAN_POINT('',(53.2,-78.,18.65));
#42974=CARTESIAN_POINT('',(53.,-78.,18.85));
#42975=CARTESIAN_POINT('Origin',(56.25,-78.,18.65));
#42976=CARTESIAN_POINT('Origin',(56.25,-78.,19.05));
#42977=CARTESIAN_POINT('',(53.2,-78.,7.05));
#42978=CARTESIAN_POINT('',(53.2,-78.,19.05));
#42979=CARTESIAN_POINT('Origin',(56.25,-78.,7.05));
#42980=CARTESIAN_POINT('Origin',(-78.,56.25,18.85));
#42981=CARTESIAN_POINT('',(-81.05,56.25,18.65));
#42982=CARTESIAN_POINT('',(-81.25,56.25,18.85));
#42983=CARTESIAN_POINT('Origin',(-78.,56.25,18.65));
#42984=CARTESIAN_POINT('Origin',(-78.,56.25,19.05));
#42985=CARTESIAN_POINT('',(-81.05,56.25,7.05));
#42986=CARTESIAN_POINT('',(-81.05,56.25,19.05));
#42987=CARTESIAN_POINT('Origin',(-78.,56.25,7.05));
#42988=CARTESIAN_POINT('Origin',(18.75,78.,18.85));
#42989=CARTESIAN_POINT('',(15.7,78.,18.65));
#42990=CARTESIAN_POINT('',(15.5,78.,18.85));
#42991=CARTESIAN_POINT('Origin',(18.75,78.,18.65));
#42992=CARTESIAN_POINT('Origin',(18.75,78.,19.05));
#42993=CARTESIAN_POINT('',(15.7,78.,7.05));
#42994=CARTESIAN_POINT('',(15.7,78.,19.05));
#42995=CARTESIAN_POINT('Origin',(18.75,78.,7.05));
#42996=CARTESIAN_POINT('Origin',(78.,-56.25,18.85));
#42997=CARTESIAN_POINT('',(74.95,-56.25,18.65));
#42998=CARTESIAN_POINT('',(74.75,-56.25,18.85));
#42999=CARTESIAN_POINT('Origin',(78.,-56.25,18.65));
#43000=CARTESIAN_POINT('Origin',(78.,-56.25,19.05));
#43001=CARTESIAN_POINT('',(74.95,-56.25,7.05));
#43002=CARTESIAN_POINT('',(74.95,-56.25,19.05));
#43003=CARTESIAN_POINT('Origin',(78.,-56.25,7.05));
#43004=CARTESIAN_POINT('Origin',(-18.75,78.,18.85));
#43005=CARTESIAN_POINT('',(-21.8,78.,18.65));
#43006=CARTESIAN_POINT('',(-22.,78.,18.85));
#43007=CARTESIAN_POINT('Origin',(-18.75,78.,18.65));
#43008=CARTESIAN_POINT('Origin',(-18.75,78.,19.05));
#43009=CARTESIAN_POINT('',(-21.8,78.,7.05));
#43010=CARTESIAN_POINT('',(-21.8,78.,19.05));
#43011=CARTESIAN_POINT('Origin',(-18.75,78.,7.05));
#43012=CARTESIAN_POINT('Origin',(78.,-18.75,18.85));
#43013=CARTESIAN_POINT('',(74.95,-18.75,18.65));
#43014=CARTESIAN_POINT('',(74.75,-18.75,18.85));
#43015=CARTESIAN_POINT('Origin',(78.,-18.75,18.65));
#43016=CARTESIAN_POINT('Origin',(78.,-18.75,19.05));
#43017=CARTESIAN_POINT('',(74.95,-18.75,7.05));
#43018=CARTESIAN_POINT('',(74.95,-18.75,19.05));
#43019=CARTESIAN_POINT('Origin',(78.,-18.75,7.05));
#43020=CARTESIAN_POINT('Origin',(-56.25,78.,18.85));
#43021=CARTESIAN_POINT('',(-59.3,78.,18.65));
#43022=CARTESIAN_POINT('',(-59.5,78.,18.85));
#43023=CARTESIAN_POINT('Origin',(-56.25,78.,18.65));
#43024=CARTESIAN_POINT('Origin',(-56.25,78.,19.05));
#43025=CARTESIAN_POINT('',(-59.3,78.,7.05));
#43026=CARTESIAN_POINT('',(-59.3,78.,19.05));
#43027=CARTESIAN_POINT('Origin',(-56.25,78.,7.05));
#43028=CARTESIAN_POINT('Origin',(-78.,-18.75,18.85));
#43029=CARTESIAN_POINT('',(-81.05,-18.75,18.65));
#43030=CARTESIAN_POINT('',(-81.25,-18.75,18.85));
#43031=CARTESIAN_POINT('Origin',(-78.,-18.75,18.65));
#43032=CARTESIAN_POINT('Origin',(-78.,-18.75,19.05));
#43033=CARTESIAN_POINT('',(-81.05,-18.75,7.05));
#43034=CARTESIAN_POINT('',(-81.05,-18.75,19.05));
#43035=CARTESIAN_POINT('Origin',(-78.,-18.75,7.05));
#43036=CARTESIAN_POINT('Origin',(78.,18.75,18.85));
#43037=CARTESIAN_POINT('',(74.95,18.75,18.65));
#43038=CARTESIAN_POINT('',(74.75,18.75,18.85));
#43039=CARTESIAN_POINT('Origin',(78.,18.75,18.65));
#43040=CARTESIAN_POINT('Origin',(78.,18.75,19.05));
#43041=CARTESIAN_POINT('',(74.95,18.75,7.05));
#43042=CARTESIAN_POINT('',(74.95,18.75,19.05));
#43043=CARTESIAN_POINT('Origin',(78.,18.75,7.05));
#43044=CARTESIAN_POINT('Origin',(-78.,18.75,18.85));
#43045=CARTESIAN_POINT('',(-81.05,18.75,18.65));
#43046=CARTESIAN_POINT('',(-81.25,18.75,18.85));
#43047=CARTESIAN_POINT('Origin',(-78.,18.75,18.65));
#43048=CARTESIAN_POINT('Origin',(-78.,18.75,19.05));
#43049=CARTESIAN_POINT('',(-81.05,18.75,7.05));
#43050=CARTESIAN_POINT('',(-81.05,18.75,19.05));
#43051=CARTESIAN_POINT('Origin',(-78.,18.75,7.05));
#43052=CARTESIAN_POINT('Origin',(78.,56.25,18.85));
#43053=CARTESIAN_POINT('',(74.95,56.25,18.65));
#43054=CARTESIAN_POINT('',(74.75,56.25,18.85));
#43055=CARTESIAN_POINT('Origin',(78.,56.25,18.65));
#43056=CARTESIAN_POINT('Origin',(78.,56.25,19.05));
#43057=CARTESIAN_POINT('',(74.95,56.25,7.05));
#43058=CARTESIAN_POINT('',(74.95,56.25,19.05));
#43059=CARTESIAN_POINT('Origin',(78.,56.25,7.05));
#43060=CARTESIAN_POINT('Origin',(56.25,78.,18.85));
#43061=CARTESIAN_POINT('',(53.2,78.,18.65));
#43062=CARTESIAN_POINT('',(53.,78.,18.85));
#43063=CARTESIAN_POINT('Origin',(56.25,78.,18.65));
#43064=CARTESIAN_POINT('Origin',(56.25,78.,19.05));
#43065=CARTESIAN_POINT('',(53.2,78.,7.05));
#43066=CARTESIAN_POINT('',(53.2,78.,19.05));
#43067=CARTESIAN_POINT('Origin',(56.25,78.,7.05));
#43068=CARTESIAN_POINT('Origin',(0.,-37.5,18.85));
#43069=CARTESIAN_POINT('',(-7.,-37.5,18.65));
#43070=CARTESIAN_POINT('',(-7.2,-37.5,18.85));
#43071=CARTESIAN_POINT('Origin',(0.,-37.5,18.65));
#43072=CARTESIAN_POINT('Origin',(0.,-37.5,19.05));
#43073=CARTESIAN_POINT('',(-7.,-37.5,19.05));
#43074=CARTESIAN_POINT('Origin',(37.5,0.,18.85));
#43075=CARTESIAN_POINT('',(30.5,8.57252759403147E-16,18.65));
#43076=CARTESIAN_POINT('',(30.3,-8.81745695386095E-16,18.85));
#43077=CARTESIAN_POINT('Origin',(37.5,0.,18.65));
#43078=CARTESIAN_POINT('Origin',(37.5,0.,19.05));
#43079=CARTESIAN_POINT('',(30.5,8.57252759403147E-16,19.05));
#43080=CARTESIAN_POINT('Origin',(-37.5,0.,18.85));
#43081=CARTESIAN_POINT('',(-44.5,8.57252759403147E-16,18.65));
#43082=CARTESIAN_POINT('',(-44.7,-8.81745695386095E-16,18.85));
#43083=CARTESIAN_POINT('Origin',(-37.5,0.,18.65));
#43084=CARTESIAN_POINT('Origin',(-37.5,0.,19.05));
#43085=CARTESIAN_POINT('',(-44.5,8.57252759403147E-16,19.05));
#43086=CARTESIAN_POINT('Origin',(0.,37.5,18.85));
#43087=CARTESIAN_POINT('',(-7.,37.5,18.65));
#43088=CARTESIAN_POINT('',(-7.2,37.5,18.85));
#43089=CARTESIAN_POINT('Origin',(0.,37.5,18.65));
#43090=CARTESIAN_POINT('Origin',(0.,37.5,19.05));
#43091=CARTESIAN_POINT('',(-7.,37.5,19.05));
#43092=CARTESIAN_POINT('Origin',(0.,-37.5,0.2));
#43093=CARTESIAN_POINT('',(-4.7,-37.5,0.2));
#43094=CARTESIAN_POINT('Origin',(37.5,0.,0.2));
#43095=CARTESIAN_POINT('',(32.8,5.75583995599256E-16,0.2));
#43096=CARTESIAN_POINT('Origin',(-37.5,0.,0.2));
#43097=CARTESIAN_POINT('',(-42.2,5.75583995599256E-16,0.2));
#43098=CARTESIAN_POINT('Origin',(0.,37.5,0.2));
#43099=CARTESIAN_POINT('',(-4.7,37.5,0.2));
#43100=CARTESIAN_POINT('Origin',(-33.475,-35.725,3.75));
#43101=CARTESIAN_POINT('Origin',(-33.475,-35.725,10.75));
#43102=CARTESIAN_POINT('Origin',(56.25,78.,7.05));
#43103=CARTESIAN_POINT('Origin',(78.,56.25,7.05));
#43104=CARTESIAN_POINT('Origin',(-78.,18.75,7.05));
#43105=CARTESIAN_POINT('Origin',(78.,18.75,7.05));
#43106=CARTESIAN_POINT('Origin',(-78.,-18.75,7.05));
#43107=CARTESIAN_POINT('Origin',(-56.25,78.,7.05));
#43108=CARTESIAN_POINT('Origin',(78.,-18.75,7.05));
#43109=CARTESIAN_POINT('Origin',(-18.75,78.,7.05));
#43110=CARTESIAN_POINT('Origin',(78.,-56.25,7.05));
#43111=CARTESIAN_POINT('Origin',(18.75,78.,7.05));
#43112=CARTESIAN_POINT('Origin',(-78.,56.25,7.05));
#43113=CARTESIAN_POINT('Origin',(56.25,-78.,7.05));
#43114=CARTESIAN_POINT('Origin',(0.,0.,19.05));
#43115=CARTESIAN_POINT('',(-5.5,-6.73555739531044E-16,17.35));
#43116=CARTESIAN_POINT('',(-5.5,6.73555739531044E-16,19.05));
#43117=CARTESIAN_POINT('Origin',(0.,0.,17.35));
#43118=CARTESIAN_POINT('Origin',(0.,0.,17.35));
#43119=CARTESIAN_POINT('Origin',(85.725,85.725,0.));
#82344=UNCERTAINTY_MEASURE_WITH_UNIT(LENGTH_MEASURE(0.01),#82385,
'DISTANCE_ACCURACY_VALUE',
'Maximum model space distance between geometric entities at asserted c
onnectivities');
#82363=UNCERTAINTY_MEASURE_WITH_UNIT(LENGTH_MEASURE(0.01),#82385,
'DISTANCE_ACCURACY_VALUE',
'Maximum model space distance between geometric entities at asserted c
onnectivities');
#82365=(
GEOMETRIC_REPRESENTATION_CONTEXT(3)
GLOBAL_UNCERTAINTY_ASSIGNED_CONTEXT((#82344))
GLOBAL_UNIT_ASSIGNED_CONTEXT((#82385,#82387,#82388))
REPRESENTATION_CONTEXT('','3D')
);
#82384=(
GEOMETRIC_REPRESENTATION_CONTEXT(3)
GLOBAL_UNCERTAINTY_ASSIGNED_CONTEXT((#82363))
GLOBAL_UNIT_ASSIGNED_CONTEXT((#82385,#82387,#82388))
REPRESENTATION_CONTEXT('','3D')
);
#82385=(
LENGTH_UNIT()
NAMED_UNIT(*)
SI_UNIT(.MILLI.,.METRE.)
);
#82387=(
NAMED_UNIT(*)
PLANE_ANGLE_UNIT()
SI_UNIT($,.RADIAN.)
);
#82388=(
NAMED_UNIT(*)
SI_UNIT($,.STERADIAN.)
SOLID_ANGLE_UNIT()
);
#82390=SHAPE_DEFINITION_REPRESENTATION(#82410,#82466);
#82410=PRODUCT_DEFINITION_SHAPE('',$,#82487);
#82466=SHAPE_REPRESENTATION('',(#30891),#82365);
#82485=PRODUCT_DEFINITION_CONTEXT('part definition',#82547,'design');
#82487=PRODUCT_DEFINITION('2026-10-20-12-38-04-055','01_Base_Plate',#82507,
#82485);
#82507=PRODUCT_DEFINITION_FORMATION('',$,#82550);
#82547=APPLICATION_CONTEXT(
'Core Data for Automotive Mechanical Design Process');
#82548=PRODUCT_CONTEXT('part definition',#82547,'mechanical');
#82550=PRODUCT('2026-10-20-12-38-04-055','01_Base_Plate',$,(#82548));
#82604=COLOUR_RGB('Dark Blue',0.08,0.2,0.34);
#82605=FILL_AREA_STYLE_COLOUR('',#82604);
#82606=FILL_AREA_STYLE('',(#82605));
#82607=SURFACE_STYLE_FILL_AREA(#82606);
#82608=SURFACE_SIDE_STYLE('',(#82607));
#82609=SURFACE_STYLE_USAGE(.BOTH.,#82608);
#82610=PRESENTATION_STYLE_ASSIGNMENT((#82609));
ENDSEC;
END-ISO-10303-21;
